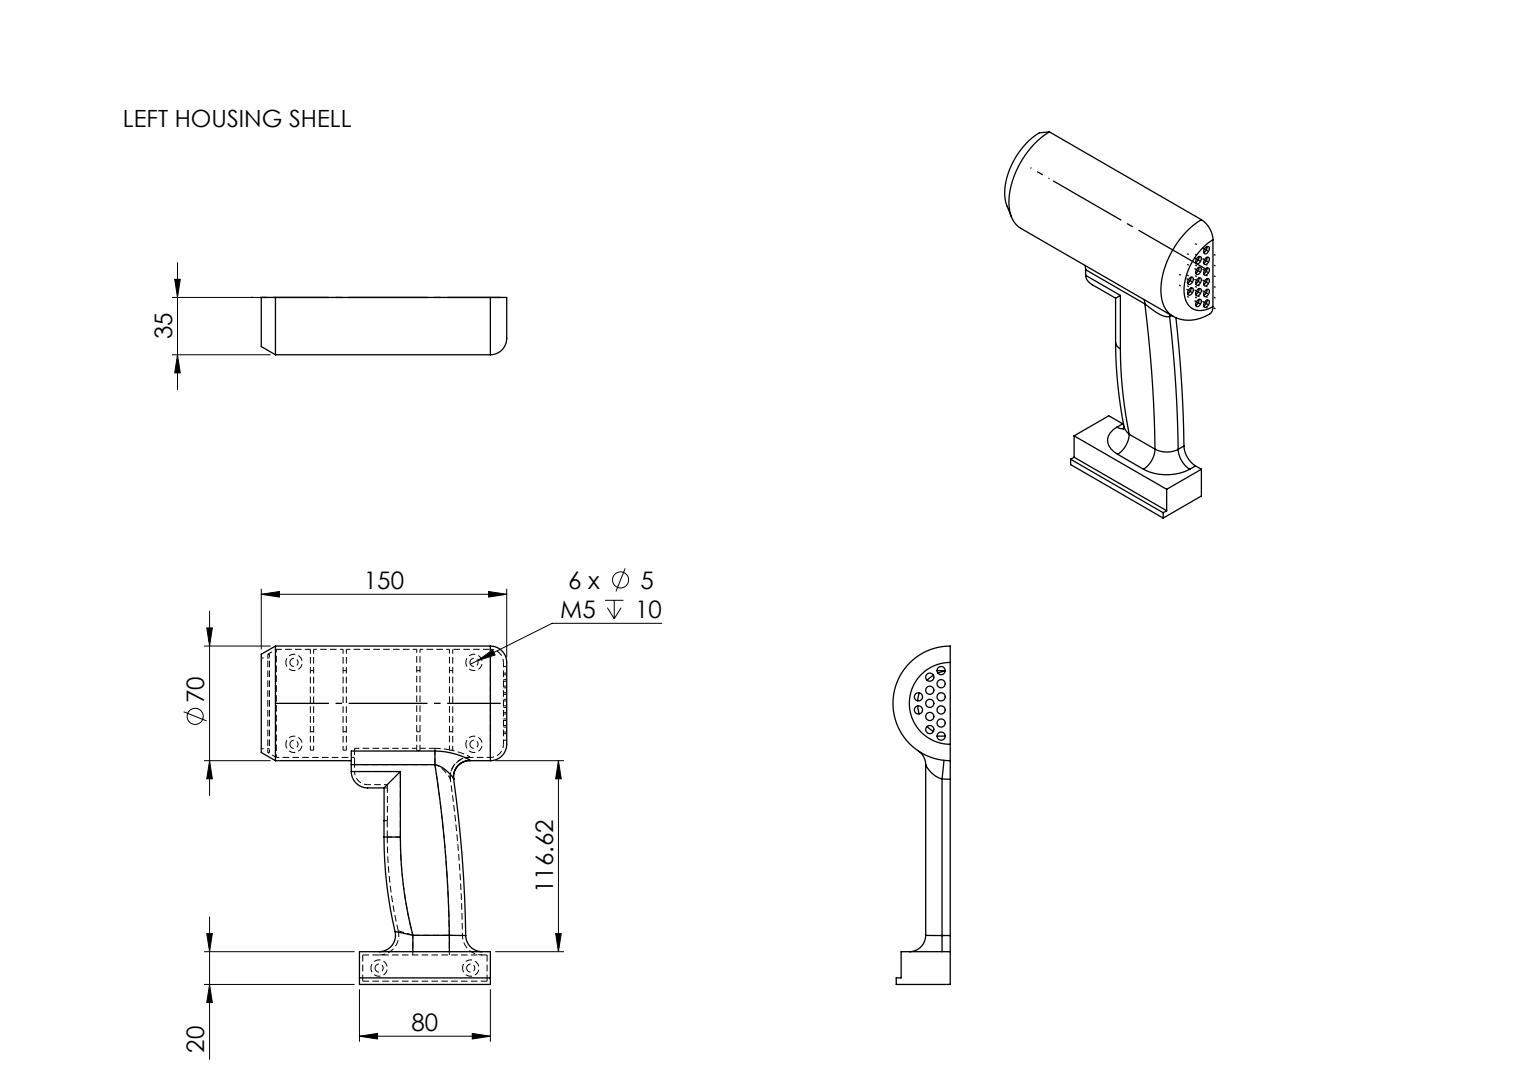
ISO-10303-21;
HEADER;
FILE_DESCRIPTION (('STEP AP214'),
    '1' );
FILE_NAME ('Left Housing Shell.step',
    '2026-10-05T20:22:16',
    ( '' ),
    ( '' ),
    'SwSTEP 2.0',
    'SolidWorks 2026',
    '' );
FILE_SCHEMA (( 'AUTOMOTIVE_DESIGN' ));
ENDSEC;

DATA;
#11=CARTESIAN_POINT ( 'NONE',  ( -70.00000000000000000, 171.6227766016838245, 0.000000000000000000 ) ) ;
#12=ORIENTED_EDGE ( 'NONE', *, *, #6579, .T. ) ;
#17=CARTESIAN_POINT ( 'NONE',  ( 196.0000000000000000, 191.6227766016837677, 3.071800142134975431 ) ) ;
#19=CYLINDRICAL_SURFACE ( 'NONE', #8941, 2.500000000000000444 ) ;
#20=ORIENTED_EDGE ( 'NONE', *, *, #455, .F. ) ;
#21=CARTESIAN_POINT ( 'NONE',  ( -12.77984573873758656, 20.00000000000230216, 11.87289823213939854 ) ) ;
#22=CARTESIAN_POINT ( 'NONE',  ( 14.63750484765316706, 138.5418767416829837, 5.508738673615532377 ) ) ;
#24=CARTESIAN_POINT ( 'NONE',  ( 21.36708699129162881, 19.99999999999999645, 23.94811280430947420 ) ) ;
#25=EDGE_CURVE ( 'NONE', #5251, #13584, #2714, .T. ) ;
#30=CARTESIAN_POINT ( 'NONE',  ( -15.00000000000002132, 100.0000000000000142, 4.999999999999999112 ) ) ;
#33=ADVANCED_FACE ( 'NONE', ( #8260 ), #11261, .F. ) ;
#34=EDGE_CURVE ( 'NONE', #17370, #11003, #7190, .T. ) ;
#39=FACE_OUTER_BOUND ( 'NONE', #11505, .T. ) ;
#42=ORIENTED_EDGE ( 'NONE', *, *, #11841, .T. ) ;
#44=CARTESIAN_POINT ( 'NONE',  ( 9.986687348566183786, 132.8041431104223307, 14.33374896416919064 ) ) ;
#47=CARTESIAN_POINT ( 'NONE',  ( -40.85786437626905609, 120.0000000000000142, 10.85786437626904721 ) ) ;
#52=DIRECTION ( 'NONE',  ( 0.000000000000000000, 0.000000000000000000, -1.000000000000000000 ) ) ;
#53=CARTESIAN_POINT ( 'NONE',  ( -80.79725519073433304, 151.5627461462769929, 26.20297826401936803 ) ) ;
#56=CARTESIAN_POINT ( 'NONE',  ( 14.34366722128227067, 129.4994645064758174, 11.74322308516846647 ) ) ;
#58=CARTESIAN_POINT ( 'NONE',  ( -43.00000000000000000, 144.1839557653416080, 18.33333333333335702 ) ) ;
#59=PLANE ( 'NONE',  #13735 ) ;
#61=EDGE_CURVE ( 'NONE', #735, #11290, #4368, .T. ) ;
#63=FACE_OUTER_BOUND ( 'NONE', #17014, .T. ) ;
#64=ORIENTED_EDGE ( 'NONE', *, *, #1601, .F. ) ;
#66=LINE ( 'NONE', #2892, #16980 ) ;
#69=CARTESIAN_POINT ( 'NONE',  ( 0.000000000000000000, 20.00000000000000000, 25.00000000000000000 ) ) ;
#74=( NAMED_UNIT ( * ) PLANE_ANGLE_UNIT ( ) SI_UNIT ( $, .RADIAN. ) );
#76=ADVANCED_FACE ( 'NONE', ( #15069 ), #3033, .F. ) ;
#78=EDGE_CURVE ( 'NONE', #10896, #7127, #13853, .T. ) ;
#81=EDGE_CURVE ( 'NONE', #4275, #9730, #165, .T. ) ;
#85=DIRECTION ( 'NONE',  ( -1.000000000000000000, -0.000000000000000000, -0.000000000000000000 ) ) ;
#91=LINE ( 'NONE', #4168, #1104 ) ;
#96=EDGE_LOOP ( 'NONE', ( #1824, #2335, #11852, #6103 ) ) ;
#100=PLANE ( 'NONE',  #16536 ) ;
#104=ORIENTED_EDGE ( 'NONE', *, *, #3991, .F. ) ;
#106=DIRECTION ( 'NONE',  ( -1.000000000000000000, 0.000000000000000000, 0.000000000000000000 ) ) ;
#120=ORIENTED_EDGE ( 'NONE', *, *, #14822, .T. ) ;
#124=CARTESIAN_POINT ( 'NONE',  ( 10.15450428991780285, 132.7081580017661224, 14.27405243007192581 ) ) ;
#132=CARTESIAN_POINT ( 'NONE',  ( -24.99999999999999289, 100.0000000000000142, 0.000000000000000000 ) ) ;
#133=CIRCLE ( 'NONE', #1548, 2.499999999999998668 ) ;
#135=CYLINDRICAL_SURFACE ( 'NONE', #5598, 8.000000000000007105 ) ;
#139=LINE ( 'NONE', #14923, #9291 ) ;
#140=FACE_OUTER_BOUND ( 'NONE', #14292, .T. ) ;
#142=CARTESIAN_POINT ( 'NONE',  ( -82.50000000000001421, 196.6227766016838245, 0.000000000000000000 ) ) ;
#143=ORIENTED_EDGE ( 'NONE', *, *, #14951, .F. ) ;
#144=EDGE_CURVE ( 'NONE', #16894, #7251, #3853, .T. ) ;
#154=CARTESIAN_POINT ( 'NONE',  ( 196.0000000000000000, 175.6227766016838530, 21.92820660268601074 ) ) ;
#156=CARTESIAN_POINT ( 'NONE',  ( -3.000000000000000888, 171.6227766016838245, 0.000000000000000000 ) ) ;
#161=DIRECTION ( 'NONE',  ( 0.000000000000000000, 0.000000000000000000, -1.000000000000000000 ) ) ;
#163=EDGE_LOOP ( 'NONE', ( #2201, #7278 ) ) ;
#165=CIRCLE ( 'NONE', #16002, 2.500000000000002220 ) ;
#167=CARTESIAN_POINT ( 'NONE',  ( -7.379000772444994638, 30.00000000000000000, 25.00000000000000000 ) ) ;
#168=CIRCLE ( 'NONE', #8369, 12.00000000000000000 ) ;
#170=CARTESIAN_POINT ( 'NONE',  ( 17.00000000000000000, 154.3022685259950038, 9.999999999999900524 ) ) ;
#172=CARTESIAN_POINT ( 'NONE',  ( 15.46067906867578046, 29.98929614515185804, 13.00000000000000533 ) ) ;
#174=EDGE_CURVE ( 'NONE', #6874, #11959, #3395, .T. ) ;
#179=CARTESIAN_POINT ( 'NONE',  ( 49.99999999999998579, 187.6227766016837961, 12.50000337241049309 ) ) ;
#186=ORIENTED_EDGE ( 'NONE', *, *, #12034, .F. ) ;
#187=CARTESIAN_POINT ( 'NONE',  ( -25.16839285024614625, 19.99999999999999645, 15.12082343620048519 ) ) ;
#189=DIRECTION ( 'NONE',  ( 0.000000000000000000, 1.000000000000000000, 0.000000000000000000 ) ) ;
#190=VERTEX_POINT ( 'NONE', #15337 ) ;
#193=CARTESIAN_POINT ( 'NONE',  ( -95.00000000000000000, 171.6227766016838245, 0.000000000000000000 ) ) ;
#199=CYLINDRICAL_SURFACE ( 'NONE', #1827, 5.000000000000000888 ) ;
#202=FACE_OUTER_BOUND ( 'NONE', #3833, .T. ) ;
#206=B_SPLINE_CURVE_WITH_KNOTS ( 'NONE', 3,
 ( #3287, #16669, #445, #365, #283, #11345, #15732, #8689, #8323, #15407, #4447, #11249, #548, #7099, #5687, #9833, #14096, #7178, #17064, #1960, #11419, #12580, #4538, #1702, #8592, #1874 ),
 .UNSPECIFIED., .F., .F.,
 ( 4, 2, 2, 2, 2, 2, 2, 2, 2, 2, 2, 2, 4 ),
 ( 0.000000000000000000, 0.002002783134349999609, 0.004005566268699999218, 0.008011132537399998435, 0.01001391567174999414, 0.01201669880609998985, 0.01602226507479997952, 0.01802504820914997002, 0.02002783134349995706, 0.02403339761219993806, 0.02603618074654992856, 0.02803896388089991906, 0.03204453014959990353 ),
 .UNSPECIFIED. ) ;
#208=ORIENTED_EDGE ( 'NONE', *, *, #12480, .F. ) ;
#210=CARTESIAN_POINT ( 'NONE',  ( 15.00000000000000000, 204.6227766016838245, -2.020667218593133100E-15 ) ) ;
#212=CARTESIAN_POINT ( 'NONE',  ( 17.58250999372313927, 125.2198453307267414, 1.671679122699602171 ) ) ;
#213=DIRECTION ( 'NONE',  ( -1.000000000000000000, 0.000000000000000000, 0.000000000000000000 ) ) ;
#215=CIRCLE ( 'NONE', #1923, 5.000000000000018652 ) ;
#216=VERTEX_POINT ( 'NONE', #8789 ) ;
#223=CARTESIAN_POINT ( 'NONE',  ( 27.44407568426044364, 136.8394969516870958, 3.888888888888887063 ) ) ;
#225=ORIENTED_EDGE ( 'NONE', *, *, #16801, .F. ) ;
#231=CARTESIAN_POINT ( 'NONE',  ( -45.00000000000000000, 122.0000000000000142, 15.00000000000000000 ) ) ;
#236=LINE ( 'NONE', #5641, #6716 ) ;
#237=EDGE_LOOP ( 'NONE', ( #1431, #15859, #12881, #16657, #10889, #7991, #12906, #8862 ) ) ;
#239=CARTESIAN_POINT ( 'NONE',  ( 196.0000000000000000, 179.6227766016838245, 15.00000337241049486 ) ) ;
#241=AXIS2_PLACEMENT_3D ( 'NONE', #3615, #7420, #699 ) ;
#244=CARTESIAN_POINT ( 'NONE',  ( -100.0000000000000000, 143.9321776784423150, -5.086680500673126297E-15 ) ) ;
#247=FACE_BOUND ( 'NONE', #9621, .T. ) ;
#248=ADVANCED_FACE ( 'NONE', ( #14797, #17095 ), #7707, .F. ) ;
#250=EDGE_CURVE ( 'NONE', #2500, #6282, #1348, .T. ) ;
#252=CIRCLE ( 'NONE', #11000, 2.500000000000000000 ) ;
#254=VERTEX_POINT ( 'NONE', #2317 ) ;
#255=FACE_BOUND ( 'NONE', #9759, .T. ) ;
#262=CIRCLE ( 'NONE', #2818, 2.499999999999998668 ) ;
#264=AXIS2_PLACEMENT_3D ( 'NONE', #14224, #8819, #502 ) ;
#266=CARTESIAN_POINT ( 'NONE',  ( 19.82112781281243130, 29.90253658286262350, 11.35562597552217845 ) ) ;
#276=CARTESIAN_POINT ( 'NONE',  ( -15.53366225407947354, 31.76144936975385136, 11.66511309525283835 ) ) ;
#277=CIRCLE ( 'NONE', #6204, 20.00000000000000355 ) ;
#279=EDGE_CURVE ( 'NONE', #3972, #817, #6479, .T. ) ;
#280=ORIENTED_EDGE ( 'NONE', *, *, #8979, .F. ) ;
#283=CARTESIAN_POINT ( 'NONE',  ( -27.70723240392776887, 18.00000000000000000, 8.328409877367404235 ) ) ;
#288=LINE ( 'NONE', #8596, #3725 ) ;
#291=DIRECTION ( 'NONE',  ( -1.000000000000000000, 0.000000000000000000, 0.000000000000000000 ) ) ;
#292=EDGE_LOOP ( 'NONE', ( #6190, #15449, #12115, #5130, #6244, #17037, #12475 ) ) ;
#294=EDGE_LOOP ( 'NONE', ( #280, #3412, #14427, #14815 ) ) ;
#306=CARTESIAN_POINT ( 'NONE',  ( 16.12877328687227774, 136.8349817083154676, 4.209125965272636272 ) ) ;
#310=CARTESIAN_POINT ( 'NONE',  ( -50.00000000000000000, 171.6227766016838245, 0.000000000000000000 ) ) ;
#312=FACE_OUTER_BOUND ( 'NONE', #3125, .T. ) ;
#315=CIRCLE ( 'NONE', #13889, 10.00000000000000178 ) ;
#317=DIRECTION ( 'NONE',  ( -1.000000000000000000, 0.000000000000000000, 0.000000000000000000 ) ) ;
#319=ORIENTED_EDGE ( 'NONE', *, *, #15425, .T. ) ;
#320=EDGE_CURVE ( 'NONE', #5614, #12465, #7243, .T. ) ;
#322=PLANE ( 'NONE',  #5083 ) ;
#324=DIRECTION ( 'NONE',  ( 0.8571673013836870192, 1.049727191973306873E-16, -0.5150380737757234151 ) ) ;
#333=CARTESIAN_POINT ( 'NONE',  ( -100.0000000000000000, 171.6227766016838245, 0.000000000000000000 ) ) ;
#335=FACE_BOUND ( 'NONE', #8357, .T. ) ;
#339=ORIENTED_EDGE ( 'NONE', *, *, #6159, .F. ) ;
#342=ORIENTED_EDGE ( 'NONE', *, *, #14528, .T. ) ;
#343=FILL_AREA_STYLE_COLOUR ( '', #7574 ) ;
#347=CARTESIAN_POINT ( 'NONE',  ( 25.75727093772393061, 193.9598103731634637, 24.29383909379279061 ) ) ;
#351=CARTESIAN_POINT ( 'NONE',  ( -79.90458729923355463, 201.6232707959690060, 13.74664867617476460 ) ) ;
#354=ORIENTED_EDGE ( 'NONE', *, *, #25, .T. ) ;
#359=CARTESIAN_POINT ( 'NONE',  ( -27.98221281347032274, 19.99999999999999645, 4.999999999999996447 ) ) ;
#364=EDGE_CURVE ( 'NONE', #14743, #3326, #2669, .T. ) ;
#365=CARTESIAN_POINT ( 'NONE',  ( -27.81025873171734375, 18.00000000000000355, 7.666431193274476641 ) ) ;
#368=DIRECTION ( 'NONE',  ( -1.000000000000000000, -0.000000000000000000, -0.000000000000000000 ) ) ;
#370=FACE_OUTER_BOUND ( 'NONE', #15719, .T. ) ;
#380=CARTESIAN_POINT ( 'NONE',  ( 15.95607457770042181, 136.6882381644217048, 2.475222843549475638 ) ) ;
#381=CARTESIAN_POINT ( 'NONE',  ( 13.38958197704232056, 130.3612470323695902, 12.52688079436099144 ) ) ;
#382=ORIENTED_EDGE ( 'NONE', *, *, #10198, .F. ) ;
#385=CARTESIAN_POINT ( 'NONE',  ( -81.89019958151206424, 191.9899036175949618, 25.96511099662697930 ) ) ;
#386=DIRECTION ( 'NONE',  ( 0.000000000000000000, 0.000000000000000000, 1.000000000000000000 ) ) ;
#387=CARTESIAN_POINT ( 'NONE',  ( 17.50698843878764777, 29.94827730614627725, 12.57924512168886011 ) ) ;
#391=ADVANCED_FACE ( 'NONE', ( #9825 ), #19, .F. ) ;
#394=EDGE_CURVE ( 'NONE', #12251, #2211, #12340, .T. ) ;
#400=ORIENTED_EDGE ( 'NONE', *, *, #61, .T. ) ;
#401=CARTESIAN_POINT ( 'NONE',  ( 8.997728150919979129, 132.8900016178789372, 12.55705910147062099 ) ) ;
#402=EDGE_LOOP ( 'NONE', ( #8088, #12658, #10491, #2591 ) ) ;
#404=CARTESIAN_POINT ( 'NONE',  ( 30.00000000000000355, 196.6227766016838245, 35.00200000000000244 ) ) ;
#405=FACE_OUTER_BOUND ( 'NONE', #3645, .T. ) ;
#407=CARTESIAN_POINT ( 'NONE',  ( -96.00000000000001421, 201.6227766016838245, 0.000000000000000000 ) ) ;
#412=CARTESIAN_POINT ( 'NONE',  ( 27.31119513844540947, 142.3932571782017931, 15.32207027268389510 ) ) ;
#414=FACE_BOUND ( 'NONE', #1666, .T. ) ;
#416=AXIS2_PLACEMENT_3D ( 'NONE', #17010, #17352, #6371 ) ;
#420=CARTESIAN_POINT ( 'NONE',  ( -50.00000000000000000, 191.6227766016837961, -1.224646799147353454E-15 ) ) ;
#423=CARTESIAN_POINT ( 'NONE',  ( 40.00000000000000711, 146.6227766016838245, 0.000000000000000000 ) ) ;
#426=FACE_BOUND ( 'NONE', #13934, .T. ) ;
#429=DIRECTION ( 'NONE',  ( -0.000000000000000000, -0.000000000000000000, -1.000000000000000000 ) ) ;
#431=CARTESIAN_POINT ( 'NONE',  ( -80.14161447679168759, 201.6221756766236979, 13.74903839801200789 ) ) ;
#435=EDGE_LOOP ( 'NONE', ( #4715, #8702, #12659, #943, #16358, #4658 ) ) ;
#438=ORIENTED_EDGE ( 'NONE', *, *, #11422, .T. ) ;
#439=CARTESIAN_POINT ( 'NONE',  ( -14.83003349241583813, 19.99999999999883116, 8.298189366023557056 ) ) ;
#445=CARTESIAN_POINT ( 'NONE',  ( -27.94760966554430937, 18.00000000000000355, 6.338314452217974626 ) ) ;
#449=PLANE ( 'NONE',  #5426 ) ;
#455=EDGE_CURVE ( 'NONE', #7796, #10705, #11208, .T. ) ;
#461=DIRECTION ( 'NONE',  ( -0.000000000000000000, -0.000000000000000000, -1.000000000000000000 ) ) ;
#465=CARTESIAN_POINT ( 'NONE',  ( 24.34257225596279639, 138.6622241066778543, 11.80661878326775494 ) ) ;
#466=VECTOR ( 'NONE', #9041, 1000.000000000000000 ) ;
#476=CARTESIAN_POINT ( 'NONE',  ( -78.09342651567857274, 191.9854139975492160, 25.96938468333279104 ) ) ;
#477=DIRECTION ( 'NONE',  ( -1.000000000000000000, -0.000000000000000000, -0.000000000000000000 ) ) ;
#478=CARTESIAN_POINT ( 'NONE',  ( 19.81659905433974700, 29.90262535319825332, 11.35915249282563444 ) ) ;
#481=DIRECTION ( 'NONE',  ( 0.000000000000000000, 1.000000000000000000, 0.000000000000000000 ) ) ;
#484=DIRECTION ( 'NONE',  ( -1.000000000000000000, 0.000000000000000000, 0.000000000000000000 ) ) ;
#488=ORIENTED_EDGE ( 'NONE', *, *, #9995, .F. ) ;
#491=CIRCLE ( 'NONE', #16041, 33.00000000000000000 ) ;
#494=CARTESIAN_POINT ( 'NONE',  ( 40.00000000000000711, 171.6227766016838245, 0.000000000000000000 ) ) ;
#501=CARTESIAN_POINT ( 'NONE',  ( 40.00000000000000711, 204.6227766016838245, -2.020667218593133100E-15 ) ) ;
#502=DIRECTION ( 'NONE',  ( -1.000000000000000000, 0.000000000000000000, 0.000000000000000000 ) ) ;
#504=AXIS2_PLACEMENT_3D ( 'NONE', #14770, #8028, #16194 ) ;
#512=LINE ( 'NONE', #4502, #12581 ) ;
#515=CIRCLE ( 'NONE', #6739, 8.000000000000000000 ) ;
#517=CARTESIAN_POINT ( 'NONE',  ( -75.00000000000002842, 146.6227766016838245, 0.000000000000000000 ) ) ;
#519=ORIENTED_EDGE ( 'NONE', *, *, #4625, .F. ) ;
#520=EDGE_CURVE ( 'NONE', #7447, #15746, #3010, .T. ) ;
#522=ADVANCED_FACE ( 'NONE', ( #13830 ), #1695, .F. ) ;
#524=EDGE_LOOP ( 'NONE', ( #9216, #14969 ) ) ;
#529=CARTESIAN_POINT ( 'NONE',  ( 27.99999999999998224, 9.999999999999998224, 0.000000000000000000 ) ) ;
#530=CARTESIAN_POINT ( 'NONE',  ( -77.50000000000001421, 196.6227766016838245, 10.00000000000000178 ) ) ;
#531=AXIS2_PLACEMENT_3D ( 'NONE', #7704, #6212, #3646 ) ;
#532=CARTESIAN_POINT ( 'NONE',  ( -79.43217333917553447, 201.5917424073650182, 13.81529814621275953 ) ) ;
#536=ORIENTED_EDGE ( 'NONE', *, *, #1514, .F. ) ;
#540=ADVANCED_FACE ( 'NONE', ( #12491 ), #2116, .T. ) ;
#541=CARTESIAN_POINT ( 'NONE',  ( 35.00000000000000711, 146.6227766016838245, 35.00200000000000244 ) ) ;
#544=VERTEX_POINT ( 'NONE', #5945 ) ;
#545=AXIS2_PLACEMENT_3D ( 'NONE', #15355, #5797, #5891 ) ;
#547=AXIS2_PLACEMENT_3D ( 'NONE', #310, #15173, #4211 ) ;
#548=CARTESIAN_POINT ( 'NONE',  ( -22.79696676584440596, 18.00000000000000711, 18.34105320469107170 ) ) ;
#549=CYLINDRICAL_SURFACE ( 'NONE', #11760, 35.00000000000000000 ) ;
#551=CARTESIAN_POINT ( 'NONE',  ( -7.379000772444995526, 18.00000000000000355, 12.99999999999999822 ) ) ;
#552=DIRECTION ( 'NONE',  ( 1.000000000000000000, 0.000000000000000000, 0.000000000000000000 ) ) ;
#557=VECTOR ( 'NONE', #9968, 1000.000000000000114 ) ;
#558=AXIS2_PLACEMENT_3D ( 'NONE', #9560, #17361, #13561 ) ;
#560=CARTESIAN_POINT ( 'NONE',  ( -90.80384757729339640, 204.6227766016838245, 0.000000000000000000 ) ) ;
#563=ORIENTED_EDGE ( 'NONE', *, *, #11755, .F. ) ;
#565=CARTESIAN_POINT ( 'NONE',  ( 23.79315516583586643, 19.99999999999999645, 22.94240041036162836 ) ) ;
#567=CARTESIAN_POINT ( 'NONE',  ( 15.80099858973940030, 127.9994182179736413, 10.08996921773076316 ) ) ;
#570=VERTEX_POINT ( 'NONE', #6023 ) ;
#572=EDGE_CURVE ( 'NONE', #3368, #13835, #6120, .T. ) ;
#573=CIRCLE ( 'NONE', #11580, 2.500000000000000444 ) ;
#576=DIRECTION ( 'NONE',  ( 0.000000000000000000, 0.000000000000000000, 1.000000000000000000 ) ) ;
#577=DIRECTION ( 'NONE',  ( -1.000000000000000000, 1.040834085586084059E-15, 0.000000000000000000 ) ) ;
#578=CARTESIAN_POINT ( 'NONE',  ( 17.01529014380724192, 17.99999999999942801, 12.76845467807931733 ) ) ;
#580=ORIENTED_EDGE ( 'NONE', *, *, #7866, .T. ) ;
#581=CARTESIAN_POINT ( 'NONE',  ( -725.0000000000000000, 30.00000000000000000, 13.00000000000000000 ) ) ;
#582=CARTESIAN_POINT ( 'NONE',  ( 225.0000000000000000, 89.99999999999997158, 4.999999999999999112 ) ) ;
#586=AXIS2_PLACEMENT_3D ( 'NONE', #156, #1313, #13701 ) ;
#587=ORIENTED_EDGE ( 'NONE', *, *, #6448, .T. ) ;
#589=ORIENTED_EDGE ( 'NONE', *, *, #4843, .T. ) ;
#591=CARTESIAN_POINT ( 'NONE',  ( 11.63249183333955017, 139.6944596454877114, 10.84829254633709184 ) ) ;
#592=ORIENTED_EDGE ( 'NONE', *, *, #11333, .F. ) ;
#594=ORIENTED_EDGE ( 'NONE', *, *, #13777, .F. ) ;
#596=DIRECTION ( 'NONE',  ( 1.000000000000000000, 0.000000000000000000, 0.000000000000000000 ) ) ;
#597=CARTESIAN_POINT ( 'NONE',  ( 13.91851620013868995, 127.9827558526829563, 9.294367823883964874 ) ) ;
#605=PLANE ( 'NONE',  #3116 ) ;
#610=ORIENTED_EDGE ( 'NONE', *, *, #4593, .T. ) ;
#611=LINE ( 'NONE', #16893, #6704 ) ;
#618=DIRECTION ( 'NONE',  ( 0.000000000000000000, 0.000000000000000000, -1.000000000000000000 ) ) ;
#620=CARTESIAN_POINT ( 'NONE',  ( -80.49255897422042949, 201.5998317580112200, 13.79770299781518972 ) ) ;
#622=ORIENTED_EDGE ( 'NONE', *, *, #10511, .F. ) ;
#629=LINE ( 'NONE', #6194, #9795 ) ;
#634=CARTESIAN_POINT ( 'NONE',  ( -27.98221281347037959, 20.00000000000000000, 4.999999999999999112 ) ) ;
#639=CARTESIAN_POINT ( 'NONE',  ( -12.55890155933014363, 17.99999999999884182, 7.515612101507582743 ) ) ;
#640=LINE ( 'NONE', #12678, #3519 ) ;
#642=ORIENTED_EDGE ( 'NONE', *, *, #1514, .T. ) ;
#647=VERTEX_POINT ( 'NONE', #3540 ) ;
#649=CARTESIAN_POINT ( 'NONE',  ( 24.93507336697333798, 29.86842105264641845, 5.660862367392566874 ) ) ;
#650=CARTESIAN_POINT ( 'NONE',  ( 14.18611645313626290, 129.6406627243902676, 11.87032202561248617 ) ) ;
#653=DIRECTION ( 'NONE',  ( -1.000000000000000000, -0.000000000000000000, -0.000000000000000000 ) ) ;
#655=CARTESIAN_POINT ( 'NONE',  ( -75.10425368493336862, 195.5720014495396981, 22.70655749026625614 ) ) ;
#658=EDGE_CURVE ( 'NONE', #1654, #17318, #629, .T. ) ;
#660=DIRECTION ( 'NONE',  ( 0.8571673013836867971, 1.049727191973306626E-16, -0.5150380737757237481 ) ) ;
#663=DIRECTION ( 'NONE',  ( 1.000000000000000000, 0.000000000000000000, -0.000000000000000000 ) ) ;
#669=ORIENTED_EDGE ( 'NONE', *, *, #10810, .F. ) ;
#670=ORIENTED_EDGE ( 'NONE', *, *, #4740, .F. ) ;
#673=LINE ( 'NONE', #4749, #14088 ) ;
#674=EDGE_LOOP ( 'NONE', ( #1760, #15151, #9125, #15624 ) ) ;
#676=DIRECTION ( 'NONE',  ( 0.000000000000000000, 1.000000000000000000, 0.000000000000000000 ) ) ;
#677=CARTESIAN_POINT ( 'NONE',  ( 11.61330907248435018, 130.6704317944142986, 11.35602788888950698 ) ) ;
#682=CARTESIAN_POINT ( 'NONE',  ( 32.67951861369070343, 142.3872899932706844, 15.31067380954020862 ) ) ;
#687=EDGE_CURVE ( 'NONE', #15915, #10010, #12076, .T. ) ;
#688=ADVANCED_FACE ( 'NONE', ( #5209 ), #12027, .F. ) ;
#692=ORIENTED_EDGE ( 'NONE', *, *, #13103, .T. ) ;
#693=CARTESIAN_POINT ( 'NONE',  ( 196.0000000000000000, 175.6227766016838245, 8.071800142134975431 ) ) ;
#695=ORIENTED_EDGE ( 'NONE', *, *, #11443, .F. ) ;
#699=DIRECTION ( 'NONE',  ( 0.000000000000000000, 0.000000000000000000, -1.000000000000000000 ) ) ;
#700=EDGE_CURVE ( 'NONE', #11501, #8340, #15923, .T. ) ;
#703=FACE_OUTER_BOUND ( 'NONE', #16932, .T. ) ;
#704=DIRECTION ( 'NONE',  ( 0.000000000000000000, 0.000000000000000000, -1.000000000000000000 ) ) ;
#705=CARTESIAN_POINT ( 'NONE',  ( -75.98683855290481404, 199.6193856840139631, 17.47499078086475777 ) ) ;
#706=CARTESIAN_POINT ( 'NONE',  ( 50.00000000000000000, 171.6227766016838245, 0.000000000000000000 ) ) ;
#708=ORIENTED_EDGE ( 'NONE', *, *, #14469, .F. ) ;
#710=ORIENTED_EDGE ( 'NONE', *, *, #6159, .T. ) ;
#712=DIRECTION ( 'NONE',  ( -0.8571673013836867971, 0.000000000000000000, -0.5150380737757237481 ) ) ;
#715=DIRECTION ( 'NONE',  ( -0.000000000000000000, -0.000000000000000000, -1.000000000000000000 ) ) ;
#716=EDGE_LOOP ( 'NONE', ( #4936, #15212, #7223, #17300 ) ) ;
#719=EDGE_CURVE ( 'NONE', #2134, #4864, #6633, .T. ) ;
#722=VECTOR ( 'NONE', #15291, 1000.000000000000000 ) ;
#723=CARTESIAN_POINT ( 'NONE',  ( 48.00000000000000000, 171.6227766016838245, 10.00000337241048953 ) ) ;
#725=CARTESIAN_POINT ( 'NONE',  ( -9.392228533940972568, 30.65825049985634010, 12.80200153553487752 ) ) ;
#728=ORIENTED_EDGE ( 'NONE', *, *, #8884, .T. ) ;
#729=LINE ( 'NONE', #14192, #7026 ) ;
#734=CIRCLE ( 'NONE', #12313, 12.00000000000000000 ) ;
#735=VERTEX_POINT ( 'NONE', #16202 ) ;
#736=CARTESIAN_POINT ( 'NONE',  ( 20.13757169487763576, 19.99999999999999289, 24.32197800972832624 ) ) ;
#738=CARTESIAN_POINT ( 'NONE',  ( 19.35452547490215736, 29.94096051140668280, 13.97567760708249551 ) ) ;
#740=EDGE_LOOP ( 'NONE', ( #2992, #17252, #2513 ) ) ;
#742=CARTESIAN_POINT ( 'NONE',  ( -27.98221281347037959, 18.00000000000000355, 0.000000000000000000 ) ) ;
#744=CARTESIAN_POINT ( 'NONE',  ( -75.75631164580342158, 193.9611582889532428, 24.29263104154016872 ) ) ;
#745=PLANE ( 'NONE',  #2292 ) ;
#747=AXIS2_PLACEMENT_3D ( 'NONE', #1269, #14466, #10656 ) ;
#748=CARTESIAN_POINT ( 'NONE',  ( -95.00000000000000000, 171.6227766016838245, 0.000000000000000000 ) ) ;
#757=ORIENTED_EDGE ( 'NONE', *, *, #700, .T. ) ;
#758=AXIS2_PLACEMENT_3D ( 'NONE', #15657, #11594, #14252 ) ;
#767=CARTESIAN_POINT ( 'NONE',  ( 6.471945315774715546, 134.1315750335306518, 12.99999999999999822 ) ) ;
#768=DIRECTION ( 'NONE',  ( 1.000000000000000000, 0.000000000000000000, 0.000000000000000000 ) ) ;
#769=CYLINDRICAL_SURFACE ( 'NONE', #12299, 20.00000000000000355 ) ;
#781=ORIENTED_EDGE ( 'NONE', *, *, #1682, .T. ) ;
#783=FACE_OUTER_BOUND ( 'NONE', #7773, .T. ) ;
#786=CARTESIAN_POINT ( 'NONE',  ( 12.82244027866276426, 141.9777490571136696, 18.60671400555900235 ) ) ;
#790=EDGE_CURVE ( 'NONE', #4054, #1871, #14156, .T. ) ;
#792=ADVANCED_FACE ( 'NONE', ( #11571 ), #7415, .T. ) ;
#798=( BOUNDED_CURVE ( )  B_SPLINE_CURVE ( 3, ( #13819, #11137, #7085, #11329 ),
 .UNSPECIFIED., .F., .F. ) 
 B_SPLINE_CURVE_WITH_KNOTS ( ( 4, 4 ),
 ( -8.881784197001252323E-16, 1.570796326794898556 ),
 .UNSPECIFIED. ) 
 CURVE ( )  GEOMETRIC_REPRESENTATION_ITEM ( )  RATIONAL_B_SPLINE_CURVE ( ( 1.000000000000000000, 0.8047378541243643824, 0.8047378541243643824, 1.000000000000000000 ) ) 
 REPRESENTATION_ITEM ( '' )  );
#805=VERTEX_POINT ( 'NONE', #8484 ) ;
#806=CARTESIAN_POINT ( 'NONE',  ( -80.00000000000002842, 146.6227766016838245, 35.00200000000000244 ) ) ;
#808=ORIENTED_EDGE ( 'NONE', *, *, #995, .F. ) ;
#810=VECTOR ( 'NONE', #1968, 1000.000000000000000 ) ;
#812=LINE ( 'NONE', #2307, #4993 ) ;
#813=CARTESIAN_POINT ( 'NONE',  ( -95.00000000000000000, 171.6227766016838245, 0.000000000000000000 ) ) ;
#814=CARTESIAN_POINT ( 'NONE',  ( -10.13698291596435119, 17.99999999999999645, 11.46558158188963539 ) ) ;
#816=CARTESIAN_POINT ( 'NONE',  ( 25.49999999999998579, 9.999999999999998224, 10.00000000000000178 ) ) ;
#817=VERTEX_POINT ( 'NONE', #15375 ) ;
#819=ORIENTED_EDGE ( 'NONE', *, *, #81, .F. ) ;
#823=EDGE_CURVE ( 'NONE', #16300, #1130, #11027, .T. ) ;
#826=DIRECTION ( 'NONE',  ( -1.000000000000000000, 0.000000000000000000, 0.000000000000000000 ) ) ;
#827=VECTOR ( 'NONE', #14654, 1000.000000000000000 ) ;
#828=CARTESIAN_POINT ( 'NONE',  ( 19.05951714192248403, 29.94485528828719367, 14.11495713418740294 ) ) ;
#830=CARTESIAN_POINT ( 'NONE',  ( 196.0000000000000000, 187.6227766016837961, 12.50000337241049309 ) ) ;
#832=VECTOR ( 'NONE', #2538, 1000.000000000000000 ) ;
#837=ORIENTED_EDGE ( 'NONE', *, *, #15585, .T. ) ;
#847=EDGE_CURVE ( 'NONE', #16728, #15915, #15300, .T. ) ;
#855=CARTESIAN_POINT ( 'NONE',  ( -13.87134331504352325, 32.05147385205248867, 10.53504704850738705 ) ) ;
#857=DIRECTION ( 'NONE',  ( 0.000000000000000000, 0.000000000000000000, -1.000000000000000000 ) ) ;
#861=CARTESIAN_POINT ( 'NONE',  ( 26.51307711398865408, 139.5431919169737967, 7.747420853565629706 ) ) ;
#869=CARTESIAN_POINT ( 'NONE',  ( 25.52968048427065284, 198.8808217108463055, 18.60648811928370350 ) ) ;
#870=ORIENTED_EDGE ( 'NONE', *, *, #16889, .F. ) ;
#871=CARTESIAN_POINT ( 'NONE',  ( 0.000000000000000000, 20.00000000000000000, 0.000000000000000000 ) ) ;
#872=CARTESIAN_POINT ( 'NONE',  ( 48.00000000000000711, 175.6227766016838245, 5.571800142134975431 ) ) ;
#873=CIRCLE ( 'NONE', #2278, 5.000000000000004441 ) ;
#875=DIRECTION ( 'NONE',  ( 0.000000000000000000, 0.9938079899999064937, -0.1111111111111109523 ) ) ;
#878=DIRECTION ( 'NONE',  ( 1.000000000000000000, 0.000000000000000000, 0.000000000000000000 ) ) ;
#882=ADVANCED_FACE ( 'NONE', ( #12736 ), #11219, .T. ) ;
#883=DIRECTION ( 'NONE',  ( -0.000000000000000000, -0.000000000000000000, -1.000000000000000000 ) ) ;
#887=CIRCLE ( 'NONE', #13615, 8.000000000000000000 ) ;
#892=FACE_OUTER_BOUND ( 'NONE', #9411, .T. ) ;
#895=ORIENTED_EDGE ( 'NONE', *, *, #16793, .T. ) ;
#900=CARTESIAN_POINT ( 'NONE',  ( -13.23954943057894873, 31.86042443463173157, 11.05847410484002680 ) ) ;
#901=CARTESIAN_POINT ( 'NONE',  ( -27.99999999999998224, 10.00000000000000000, 0.000000000000000000 ) ) ;
#906=CARTESIAN_POINT ( 'NONE',  ( 49.99999999999998579, 171.6227766016838245, 12.50000337241049131 ) ) ;
#911=FACE_OUTER_BOUND ( 'NONE', #5499, .T. ) ;
#912=CARTESIAN_POINT ( 'NONE',  ( 23.61360151038711308, 29.88540148010350705, 10.01045486545366181 ) ) ;
#917=EDGE_CURVE ( 'NONE', #1967, #544, #4724, .T. ) ;
#920=CARTESIAN_POINT ( 'NONE',  ( 48.00000000000000711, 155.6227766016839098, 15.00000337241049486 ) ) ;
#923=DIRECTION ( 'NONE',  ( 0.000000000000000000, 1.387778780781445676E-14, -1.000000000000000000 ) ) ;
#926=ORIENTED_EDGE ( 'NONE', *, *, #9179, .F. ) ;
#934=CARTESIAN_POINT ( 'NONE',  ( 23.09107716886297013, 17.99999999999083045, 5.538990817933215460 ) ) ;
#938=VERTEX_POINT ( 'NONE', #7842 ) ;
#941=DIRECTION ( 'NONE',  ( -0.000000000000000000, -0.000000000000000000, -1.000000000000000000 ) ) ;
#942=CARTESIAN_POINT ( 'NONE',  ( 17.53512989260226362, 29.96507997281579350, 14.66107963853301399 ) ) ;
#943=ORIENTED_EDGE ( 'NONE', *, *, #15549, .T. ) ;
#945=CARTESIAN_POINT ( 'NONE',  ( 30.21607733469937429, 201.6195082837481038, 13.75486997215867291 ) ) ;
#948=ORIENTED_EDGE ( 'NONE', *, *, #5128, .T. ) ;
#949=CARTESIAN_POINT ( 'NONE',  ( -79.08361844431172472, 141.7021811473759669, 13.91989935049637062 ) ) ;
#950=DIRECTION ( 'NONE',  ( 1.000000000000000000, 0.000000000000000000, 0.000000000000000000 ) ) ;
#956=CARTESIAN_POINT ( 'NONE',  ( 48.00000000000000000, 196.6227766016838245, 0.000000000000000000 ) ) ;
#958=ORIENTED_EDGE ( 'NONE', *, *, #11073, .T. ) ;
#961=VECTOR ( 'NONE', #878, 1000.000000000000000 ) ;
#963=ORIENTED_EDGE ( 'NONE', *, *, #823, .F. ) ;
#967=DIRECTION ( 'NONE',  ( -0.000000000000000000, -0.000000000000000000, -1.000000000000000000 ) ) ;
#968=EDGE_CURVE ( 'NONE', #15581, #8813, #1708, .T. ) ;
#973=CARTESIAN_POINT ( 'NONE',  ( -12.54944958582184888, 31.64997543288135873, 11.54276402733058937 ) ) ;
#974=DIRECTION ( 'NONE',  ( -0.000000000000000000, -0.000000000000000000, -1.000000000000000000 ) ) ;
#977=DIRECTION ( 'NONE',  ( -0.000000000000000000, -0.000000000000000000, -1.000000000000000000 ) ) ;
#978=VERTEX_POINT ( 'NONE', #10499 ) ;
#981=ORIENTED_EDGE ( 'NONE', *, *, #16898, .T. ) ;
#983=CARTESIAN_POINT ( 'NONE',  ( 25.87766738269754541, 139.8661988410599406, 8.984976992518891592 ) ) ;
#984=CIRCLE ( 'NONE', #416, 2.500000000000000000 ) ;
#986=CARTESIAN_POINT ( 'NONE',  ( 34.42312820345349422, 19.99999999999999645, 9.539278825327816236 ) ) ;
#995=EDGE_CURVE ( 'NONE', #13884, #3234, #12362, .T. ) ;
#999=ORIENTED_EDGE ( 'NONE', *, *, #17387, .F. ) ;
#1001=AXIS2_PLACEMENT_3D ( 'NONE', #7737, #14563, #8984 ) ;
#1002=DIRECTION ( 'NONE',  ( -1.000000000000000000, 0.000000000000000000, 0.000000000000000000 ) ) ;
#1007=UNCERTAINTY_MEASURE_WITH_UNIT (LENGTH_MEASURE( 1.000000000000000082E-05 ), #2734, 'distance_accuracy_value', 'NONE');
#1011=DIRECTION ( 'NONE',  ( -1.000000000000000000, 0.000000000000000000, 0.000000000000000000 ) ) ;
#1014=CARTESIAN_POINT ( 'NONE',  ( 17.00000000000000000, 171.6227766016838245, 20.00000000000000355 ) ) ;
#1015=CARTESIAN_POINT ( 'NONE',  ( 22.25017171248248005, 17.99999999999771916, 8.611421531743401303 ) ) ;
#1018=CARTESIAN_POINT ( 'NONE',  ( 27.44407568426044008, 138.8271129316868837, 3.666666666666658081 ) ) ;
#1020=DIRECTION ( 'NONE',  ( -0.000000000000000000, -0.000000000000000000, -1.000000000000000000 ) ) ;
#1023=ORIENTED_EDGE ( 'NONE', *, *, #8940, .T. ) ;
#1024=DIRECTION ( 'NONE',  ( 0.000000000000000000, 0.000000000000000000, -1.000000000000000000 ) ) ;
#1027=AXIS2_PLACEMENT_3D ( 'NONE', #6143, #14706, #8870 ) ;
#1033=EDGE_LOOP ( 'NONE', ( #17321, #14333 ) ) ;
#1038=CARTESIAN_POINT ( 'NONE',  ( -82.95659350918997177, 142.5787592618052315, 15.67196037041395229 ) ) ;
#1044=VERTEX_POINT ( 'NONE', #16092 ) ;
#1045=DIRECTION ( 'NONE',  ( -0.000000000000000000, -0.000000000000000000, 1.000000000000000000 ) ) ;
#1046=CARTESIAN_POINT ( 'NONE',  ( -96.00000000000001421, 171.6227766016838245, 0.000000000000000000 ) ) ;
#1048=B_SPLINE_CURVE_WITH_KNOTS ( 'NONE', 3,
 ( #12094, #12187, #1202, #6519, #10675, #4125, #1292, #10927, #56, #16350, #4049, #11910, #9347, #7932, #5456, #17316, #14830, #4218, #5184, #6605, #17502, #15985 ),
 .UNSPECIFIED., .F., .F.,
 ( 4, 2, 2, 2, 2, 2, 2, 2, 2, 2, 4 ),
 ( 0.000000000000000000, 0.002375333402909271790, 0.004750666805818540978, 0.007126000208727810599, 0.009501333611637081955, 0.01068900031309169378, 0.01187666701454630908, 0.01425200041745553273, 0.01543966711891012200, 0.01662733382036471128, 0.01900266722327392452 ),
 .UNSPECIFIED. ) ;
#1050=ORIENTED_EDGE ( 'NONE', *, *, #14204, .T. ) ;
#1051=DIRECTION ( 'NONE',  ( -1.000000000000000000, -0.000000000000000000, -0.000000000000000000 ) ) ;
#1052=EDGE_CURVE ( 'NONE', #16728, #16016, #10683, .T. ) ;
#1056=DIRECTION ( 'NONE',  ( 0.000000000000000000, -1.000000000000000000, 7.341990890863118602E-16 ) ) ;
#1059=ORIENTED_EDGE ( 'NONE', *, *, #1533, .T. ) ;
#1061=CARTESIAN_POINT ( 'NONE',  ( -43.00000000000000000, 130.0000000000000000, 15.00000000000000000 ) ) ;
#1063=CARTESIAN_POINT ( 'NONE',  ( -90.80384757729339640, 204.6227766016838245, 0.000000000000000000 ) ) ;
#1066=DIRECTION ( 'NONE',  ( -1.000000000000000000, 0.000000000000000000, 0.000000000000000000 ) ) ;
#1069=CARTESIAN_POINT ( 'NONE',  ( -725.0000000000000000, 19.99999999999995737, 13.00000000000000000 ) ) ;
#1073=CYLINDRICAL_SURFACE ( 'NONE', #5904, 9.999999999999994671 ) ;
#1074=VERTEX_POINT ( 'NONE', #5461 ) ;
#1075=EDGE_CURVE ( 'NONE', #1461, #805, #9519, .T. ) ;
#1080=CARTESIAN_POINT ( 'NONE',  ( 26.57417986947462651, 139.5089559931849692, 7.600184560211070917 ) ) ;
#1082=VECTOR ( 'NONE', #2070, 1000.000000000000000 ) ;
#1085=ORIENTED_EDGE ( 'NONE', *, *, #3481, .T. ) ;
#1087=CARTESIAN_POINT ( 'NONE',  ( -45.00000000000000000, 171.6227766016838245, 0.000000000000000000 ) ) ;
#1090=ORIENTED_EDGE ( 'NONE', *, *, #11674, .T. ) ;
#1099=ORIENTED_EDGE ( 'NONE', *, *, #6963, .F. ) ;
#1103=EDGE_CURVE ( 'NONE', #1074, #16221, #15014, .T. ) ;
#1104=VECTOR ( 'NONE', #1505, 1000.000000000000000 ) ;
#1107=VECTOR ( 'NONE', #12507, 1000.000000000000000 ) ;
#1108=CARTESIAN_POINT ( 'NONE',  ( -12.31336727611479631, 31.57746213708666971, 11.68681022658133806 ) ) ;
#1109=AXIS2_PLACEMENT_3D ( 'NONE', #12893, #768, #9885 ) ;
#1112=CARTESIAN_POINT ( 'NONE',  ( 20.95008785553089581, 29.88049067427350280, 10.28044474760307914 ) ) ;
#1113=CARTESIAN_POINT ( 'NONE',  ( -84.53126297072897444, 148.7415597018667199, 23.77993541092453000 ) ) ;
#1115=DIRECTION ( 'NONE',  ( -1.000000000000000000, 0.000000000000000000, -8.673617379884037937E-17 ) ) ;
#1117=LINE ( 'NONE', #9603, #8779 ) ;
#1118=CARTESIAN_POINT ( 'NONE',  ( 17.55923266082603007, 17.99999999999999645, 24.87049340120105612 ) ) ;
#1120=ORIENTED_EDGE ( 'NONE', *, *, #16638, .T. ) ;
#1124=AXIS2_PLACEMENT_3D ( 'NONE', #7031, #4466, #16505 ) ;
#1130=VERTEX_POINT ( 'NONE', #142 ) ;
#1136=CARTESIAN_POINT ( 'NONE',  ( -34.99999999999999289, 130.0000000000000000, 15.00000000000000000 ) ) ;
#1141=DIRECTION ( 'NONE',  ( -0.000000000000000000, -0.000000000000000000, -1.000000000000000000 ) ) ;
#1144=DIRECTION ( 'NONE',  ( -1.000000000000000000, -0.000000000000000000, -0.000000000000000000 ) ) ;
#1145=ORIENTED_EDGE ( 'NONE', *, *, #11841, .F. ) ;
#1150=CARTESIAN_POINT ( 'NONE',  ( 34.93420767853316988, 18.00000000000000355, 0.000000000000000000 ) ) ;
#1151=CARTESIAN_POINT ( 'NONE',  ( 49.99999999999998579, 163.6227766016838530, 12.50000337241049309 ) ) ;
#1152=DIRECTION ( 'NONE',  ( -1.000000000000000000, -0.000000000000000000, -0.000000000000000000 ) ) ;
#1154=DIRECTION ( 'NONE',  ( 1.000000000000000000, 0.000000000000000000, 0.000000000000000000 ) ) ;
#1157=AXIS2_PLACEMENT_3D ( 'NONE', #9341, #15001, #16173 ) ;
#1158=CARTESIAN_POINT ( 'NONE',  ( -16.30611068361784532, 32.76923076923076650, 4.999999999999998224 ) ) ;
#1164=VERTEX_POINT ( 'NONE', #10039 ) ;
#1165=LINE ( 'NONE', #11957, #3637 ) ;
#1171=DIRECTION ( 'NONE',  ( -1.156482317317868274E-16, 1.000000000000000000, 0.000000000000000000 ) ) ;
#1172=CARTESIAN_POINT ( 'NONE',  ( 18.85693063297101801, 142.3798671548016159, 15.29581099734062022 ) ) ;
#1175=ORIENTED_EDGE ( 'NONE', *, *, #17079, .T. ) ;
#1178=CYLINDRICAL_SURFACE ( 'NONE', #9082, 2.500000000000000444 ) ;
#1180=ORIENTED_EDGE ( 'NONE', *, *, #2081, .F. ) ;
#1181=DIRECTION ( 'NONE',  ( -1.000000000000000000, -6.938893903907228378E-16, 0.000000000000000000 ) ) ;
#1182=ORIENTED_EDGE ( 'NONE', *, *, #17382, .T. ) ;
#1186=ORIENTED_EDGE ( 'NONE', *, *, #14469, .T. ) ;
#1189=ORIENTED_EDGE ( 'NONE', *, *, #10276, .T. ) ;
#1191=ADVANCED_FACE ( 'NONE', ( #911 ), #322, .T. ) ;
#1193=EDGE_CURVE ( 'NONE', #16427, #7978, #1741, .T. ) ;
#1198=CARTESIAN_POINT ( 'NONE',  ( -75.46486027377252981, 148.7497411309094844, 23.78985390322973714 ) ) ;
#1199=VERTEX_POINT ( 'NONE', #3236 ) ;
#1201=DIRECTION ( 'NONE',  ( 1.000000000000000000, -0.000000000000000000, -0.000000000000000000 ) ) ;
#1202=CARTESIAN_POINT ( 'NONE',  ( 17.39133856982844506, 125.9242906883583970, 6.521754810248964418 ) ) ;
#1207=CARTESIAN_POINT ( 'NONE',  ( 29.50744102577957761, 201.5998317580112200, 13.79770299781523413 ) ) ;
#1215=AXIS2_PLACEMENT_3D ( 'NONE', #10912, #3879, #6436 ) ;
#1218=CARTESIAN_POINT ( 'NONE',  ( -12.63167751028161589, 20.00000000000000355, 24.35243221814332060 ) ) ;
#1220=CARTESIAN_POINT ( 'NONE',  ( -40.00000000000000000, 4.000000000000000000, 30.00000000000000711 ) ) ;
#1222=DIRECTION ( 'NONE',  ( 0.000000000000000000, 0.000000000000000000, -1.000000000000000000 ) ) ;
#1224=ADVANCED_FACE ( 'NONE', ( #3655 ), #8591, .T. ) ;
#1227=VERTEX_POINT ( 'NONE', #10461 ) ;
#1230=LINE ( 'NONE', #13183, #8950 ) ;
#1233=EDGE_CURVE ( 'NONE', #8974, #10007, #14992, .T. ) ;
#1234=CARTESIAN_POINT ( 'NONE',  ( 49.99999999999998579, 183.6227766016837961, 5.571800142134975431 ) ) ;
#1237=CARTESIAN_POINT ( 'NONE',  ( -38.00000000000000000, 2.000000000000000000, 0.000000000000000000 ) ) ;
#1238=LINE ( 'NONE', #9294, #4157 ) ;
#1249=CARTESIAN_POINT ( 'NONE',  ( -40.00000000000000000, 0.000000000000000000, 30.00000000000000355 ) ) ;
#1251=CARTESIAN_POINT ( 'NONE',  ( -10.84365596476886395, 30.77158821550125722, 14.49076147631418721 ) ) ;
#1252=CARTESIAN_POINT ( 'NONE',  ( 15.56337975240378846, 125.2134999403455851, 5.000000000000001776 ) ) ;
#1257=EDGE_CURVE ( 'NONE', #4434, #6774, #2765, .T. ) ;
#1266=CARTESIAN_POINT ( 'NONE',  ( 31.88903224608757014, 151.2561509761041521, 25.96550485207007242 ) ) ;
#1267=ORIENTED_EDGE ( 'NONE', *, *, #10879, .F. ) ;
#1269=CARTESIAN_POINT ( 'NONE',  ( 6.134011831684059501, 134.2062027339443944, 24.99999999999999645 ) ) ;
#1271=VECTOR ( 'NONE', #13608, 1000.000000000000000 ) ;
#1274=ORIENTED_EDGE ( 'NONE', *, *, #7864, .F. ) ;
#1276=ADVANCED_FACE ( 'NONE', ( #8318 ), #3109, .F. ) ;
#1277=DIRECTION ( 'NONE',  ( 0.000000000000000000, 0.000000000000000000, -1.000000000000000000 ) ) ;
#1282=PLANE ( 'NONE',  #4700 ) ;
#1287=CIRCLE ( 'NONE', #12024, 33.00000000000000000 ) ;
#1288=ORIENTED_EDGE ( 'NONE', *, *, #2762, .F. ) ;
#1289=CARTESIAN_POINT ( 'NONE',  ( -95.00000000000000000, 141.6227766016838245, -5.510910596163088767E-15 ) ) ;
#1292=CARTESIAN_POINT ( 'NONE',  ( 15.65639489742288681, 128.1581396164810940, 10.28488489824641761 ) ) ;
#1293=CARTESIAN_POINT ( 'NONE',  ( 24.94691999498327206, 18.00000000000000711, 22.32501294936691139 ) ) ;
#1301=VERTEX_POINT ( 'NONE', #12231 ) ;
#1303=EDGE_LOOP ( 'NONE', ( #11441, #8846, #10583, #13960 ) ) ;
#1305=CARTESIAN_POINT ( 'NONE',  ( -40.00000000000000000, 4.000000000000000000, 33.00000000000000711 ) ) ;
#1312=CARTESIAN_POINT ( 'NONE',  ( 25.49999999999998579, 9.999999999999998224, 0.000000000000000000 ) ) ;
#1313=DIRECTION ( 'NONE',  ( 1.000000000000000000, 0.000000000000000000, 0.000000000000000000 ) ) ;
#1316=ORIENTED_EDGE ( 'NONE', *, *, #2532, .T. ) ;
#1321=VECTOR ( 'NONE', #8240, 1000.000000000000000 ) ;
#1323=VECTOR ( 'NONE', #16410, 1000.000000000000000 ) ;
#1325=DIRECTION ( 'NONE',  ( 0.000000000000000000, 0.000000000000000000, 1.000000000000000000 ) ) ;
#1326=AXIS2_PLACEMENT_3D ( 'NONE', #7125, #1990, #12349 ) ;
#1329=EDGE_CURVE ( 'NONE', #16720, #11161, #11838, .T. ) ;
#1333=DIRECTION ( 'NONE',  ( -0.000000000000000000, -0.000000000000000000, -1.000000000000000000 ) ) ;
#1337=DIRECTION ( 'NONE',  ( -0.000000000000000000, -0.000000000000000000, -1.000000000000000000 ) ) ;
#1339=AXIS2_PLACEMENT_3D ( 'NONE', #16014, #2207, #14432 ) ;
#1344=ORIENTED_EDGE ( 'NONE', *, *, #16537, .T. ) ;
#1348=LINE ( 'NONE', #12051, #466 ) ;
#1349=VERTEX_POINT ( 'NONE', #6910 ) ;
#1350=CARTESIAN_POINT ( 'NONE',  ( -12.14981508666162036, 19.99999999999543121, 12.53017279448777366 ) ) ;
#1356=CYLINDRICAL_SURFACE ( 'NONE', #8665, 27.69059892324149530 ) ;
#1359=DIRECTION ( 'NONE',  ( -1.000000000000000000, 0.000000000000000000, 0.000000000000000000 ) ) ;
#1361=CARTESIAN_POINT ( 'NONE',  ( 29.00744693363358806, 151.5270838226223873, 26.17568438743891335 ) ) ;
#1365=DIRECTION ( 'NONE',  ( -1.000000000000000000, 0.000000000000000000, 0.000000000000000000 ) ) ;
#1366=( BOUNDED_SURFACE ( )  B_SPLINE_SURFACE ( 3, 2, ( 
 ( #1877, #551, #4626 ),
 ( #10001, #15412, #17087 ),
 ( #2309, #9116, #15760 ),
 ( #11605, #6287, #725 ),
 ( #7615, #12844, #11514 ),
 ( #11678, #5050, #3550 ),
 ( #14188, #814, #12937 ),
 ( #6032, #8935, #7699 ),
 ( #13106, #15505, #13029 ),
 ( #3382, #11426, #973 ),
 ( #6373, #11768, #10352 ),
 ( #15857, #14350, #900 ),
 ( #2049, #16835, #7528 ),
 ( #16926, #3642, #6208 ),
 ( #3730, #2127, #17011 ),
 ( #10266, #4959, #4877 ),
 ( #9032, #639, #8853 ),
 ( #4707, #17178, #10190 ),
 ( #14261, #2218, #10448 ),
 ( #14443, #4798, #1963 ),
 ( #7367, #15668, #15591 ),
 ( #12768, #10097, #3466 ),
 ( #7442, #8780, #6118 ),
 ( #13374, #13554, #1158 ) ),
 .UNSPECIFIED., .F., .F., .F. ) 
 B_SPLINE_SURFACE_WITH_KNOTS ( ( 4, 2, 2, 2, 2, 2, 2, 2, 2, 2, 2, 4 ),
 ( 3, 3 ),
 ( 0.01427588378380421734, 0.01824401167166928364, 0.02022807561560181766, 0.02221213955953435168, 0.02618026744739941625, 0.02816433139133195027, 0.03014839533526448428, 0.03411652322312955232, 0.03610058716706208287, 0.03808465111099461342, 0.04205277899885968146, 0.04602090688672474950 ),
 ( 0.000000000000000000, 1.000000000000000000 ),
 .UNSPECIFIED. ) 
 GEOMETRIC_REPRESENTATION_ITEM ( )  RATIONAL_B_SPLINE_SURFACE ( (
 ( 1.000000000000000000, 0.7071067811865476838, 1.000000000000000000),
 ( 1.000000000000000000, 0.7013659285812973154, 1.000000000000000000),
 ( 1.000000000000000000, 0.6957352470445186121, 1.000000000000000000),
 ( 1.000000000000000000, 0.6874449304734518984, 1.000000000000000000),
 ( 1.000000000000000000, 0.6847075230360146758, 1.000000000000000000),
 ( 1.000000000000000000, 0.6792848743381181276, 1.000000000000000000),
 ( 1.000000000000000000, 0.6765866164120997173, 1.000000000000000000),
 ( 1.000000000000000000, 0.6687223666255138754, 1.000000000000000000),
 ( 1.000000000000000000, 0.6637534122519734847, 1.000000000000000000),
 ( 1.000000000000000000, 0.6567012635109988894, 1.000000000000000000),
 ( 1.000000000000000000, 0.6544178910916050862, 1.000000000000000000),
 ( 1.000000000000000000, 0.6499901663948596253, 1.000000000000000000),
 ( 1.000000000000000000, 0.6478648508490586488, 1.000000000000000000),
 ( 1.000000000000000000, 0.6418284244075036504, 1.000000000000000000),
 ( 1.000000000000000000, 0.6382188548936987837, 1.000000000000000000),
 ( 1.000000000000000000, 0.6334349500989925330, 1.000000000000000000),
 ( 1.000000000000000000, 0.6319385063093012622, 1.000000000000000000),
 ( 1.000000000000000000, 0.6292162870120669993, 1.000000000000000000),
 ( 1.000000000000000000, 0.6279881568153810045, 1.000000000000000000),
 ( 1.000000000000000000, 0.6246939197237914021, 1.000000000000000000),
 ( 1.000000000000000000, 0.6230139244306683866, 1.000000000000000000),
 ( 1.000000000000000000, 0.6207349535630238835, 1.000000000000000000),
 ( 1.000000000000000000, 0.6201739322038456459, 1.000000000000000000),
 ( 1.000000000000000000, 0.6201736729460424202, 1.000000000000000000) ) ) 
 REPRESENTATION_ITEM ( '' )  SURFACE ( )  );
#1369=ORIENTED_EDGE ( 'NONE', *, *, #3514, .F. ) ;
#1370=EDGE_LOOP ( 'NONE', ( #2054, #9589, #12874, #6617, #1090, #12711, #3516 ) ) ;
#1373=CARTESIAN_POINT ( 'NONE',  ( 12.56741672263968290, 142.0153054307823481, 18.66563201629009328 ) ) ;
#1377=DIRECTION ( 'NONE',  ( 0.000000000000000000, 0.000000000000000000, -1.000000000000000000 ) ) ;
#1379=DIRECTION ( 'NONE',  ( 0.000000000000000000, 1.000000000000000000, 0.000000000000000000 ) ) ;
#1380=DIRECTION ( 'NONE',  ( 0.000000000000000000, 0.000000000000000000, -1.000000000000000000 ) ) ;
#1381=AXIS2_PLACEMENT_3D ( 'NONE', #2085, #3164, #6248 ) ;
#1382=ORIENTED_EDGE ( 'NONE', *, *, #14861, .F. ) ;
#1388=CARTESIAN_POINT ( 'NONE',  ( 14.93242934743711992, 18.00000000000000355, 25.00000000000000000 ) ) ;
#1390=FACE_OUTER_BOUND ( 'NONE', #16381, .T. ) ;
#1391=AXIS2_PLACEMENT_3D ( 'NONE', #9461, #9297, #14520 ) ;
#1397=ORIENTED_EDGE ( 'NONE', *, *, #15063, .T. ) ;
#1399=CARTESIAN_POINT ( 'NONE',  ( -85.00000000000007105, 146.0036328918051254, 20.82208359987473401 ) ) ;
#1402=DIRECTION ( 'NONE',  ( -1.000000000000000000, 0.000000000000000000, 0.000000000000000000 ) ) ;
#1403=ORIENTED_EDGE ( 'NONE', *, *, #4744, .T. ) ;
#1404=FACE_OUTER_BOUND ( 'NONE', #12164, .T. ) ;
#1405=CIRCLE ( 'NONE', #11292, 2.499999999999998668 ) ;
#1406=AXIS2_PLACEMENT_3D ( 'NONE', #10309, #6169, #7577 ) ;
#1407=DIRECTION ( 'NONE',  ( -2.674902700537819740E-31, 2.312964634635742267E-15, 1.000000000000000000 ) ) ;
#1408=CIRCLE ( 'NONE', #2527, 2.500000000000000444 ) ;
#1414=CARTESIAN_POINT ( 'NONE',  ( 48.00000000000000000, 171.6227766016838245, 0.000000000000000000 ) ) ;
#1418=ORIENTED_EDGE ( 'NONE', *, *, #10636, .F. ) ;
#1431=ORIENTED_EDGE ( 'NONE', *, *, #12069, .F. ) ;
#1435=EDGE_LOOP ( 'NONE', ( #16840, #13854, #4027, #12176 ) ) ;
#1436=CARTESIAN_POINT ( 'NONE',  ( 37.99999999999998579, 20.00000000000000000, 30.00000000000001066 ) ) ;
#1437=CONICAL_SURFACE ( 'NONE', #13880, 2.499999999999998668, 1.029744260000002187 ) ;
#1438=EDGE_CURVE ( 'NONE', #1227, #11461, #1405, .T. ) ;
#1439=ORIENTED_EDGE ( 'NONE', *, *, #968, .T. ) ;
#1442=ORIENTED_EDGE ( 'NONE', *, *, #3814, .T. ) ;
#1444=CIRCLE ( 'NONE', #11332, 5.000000000000004441 ) ;
#1449=ORIENTED_EDGE ( 'NONE', *, *, #16449, .F. ) ;
#1452=CARTESIAN_POINT ( 'NONE',  ( -45.00000000000000000, 120.0000000000000142, 15.00000000000000000 ) ) ;
#1456=CARTESIAN_POINT ( 'NONE',  ( -38.00000000000000000, 2.000000000000000000, 28.00000000000000355 ) ) ;
#1459=DIRECTION ( 'NONE',  ( 0.000000000000000000, 0.000000000000000000, -1.000000000000000000 ) ) ;
#1461=VERTEX_POINT ( 'NONE', #7436 ) ;
#1462=DIRECTION ( 'NONE',  ( 0.000000000000000000, 0.000000000000000000, -1.000000000000000000 ) ) ;
#1466=CARTESIAN_POINT ( 'NONE',  ( 40.00000000000000711, 136.6227766016838245, 0.000000000000000000 ) ) ;
#1471=CARTESIAN_POINT ( 'NONE',  ( -84.24740733152653149, 149.2783667126899445, 24.28707720053398944 ) ) ;
#1472=ORIENTED_EDGE ( 'NONE', *, *, #1487, .T. ) ;
#1473=( BOUNDED_SURFACE ( )  B_SPLINE_SURFACE ( 3, 2, ( 
 ( #15073, #11091, #5618 ),
 ( #212, #9763, #8612 ),
 ( #13759, #380, #4554 ),
 ( #14023, #9853, #7285 ) ),
 .UNSPECIFIED., .F., .F., .F. ) 
 B_SPLINE_SURFACE_WITH_KNOTS ( ( 4, 4 ),
 ( 3, 3 ),
 ( 0.1516087691302827056, 0.1566150273425061523 ),
 ( 0.000000000000000000, 1.000000000000000000 ),
 .UNSPECIFIED. ) 
 GEOMETRIC_REPRESENTATION_ITEM ( )  RATIONAL_B_SPLINE_SURFACE ( (
 ( 1.000000000000000000, 0.6556320892438534109, 1.000000000000000000),
 ( 1.000000000000000000, 0.6556321914870764100, 1.000000000000000000),
 ( 1.000000000000000000, 0.6556957163104859543, 1.000000000000000000),
 ( 1.000000000000000000, 0.6558243695371223092, 1.000000000000000000) ) ) 
 REPRESENTATION_ITEM ( '' )  SURFACE ( )  );
#1477=FACE_OUTER_BOUND ( 'NONE', #237, .T. ) ;
#1480=CARTESIAN_POINT ( 'NONE',  ( 196.0000000000000000, 163.6227766016838530, 10.00000337241049309 ) ) ;
#1482=CARTESIAN_POINT ( 'NONE',  ( -77.50000000000001421, 196.6227766016838245, 10.00000000000000178 ) ) ;
#1487=EDGE_CURVE ( 'NONE', #3421, #15746, #11599, .T. ) ;
#1488=CARTESIAN_POINT ( 'NONE',  ( 49.99999999999998579, 171.6227766016838245, 12.50000337241049131 ) ) ;
#1492=FACE_OUTER_BOUND ( 'NONE', #8201, .T. ) ;
#1496=ORIENTED_EDGE ( 'NONE', *, *, #10090, .T. ) ;
#1502=CARTESIAN_POINT ( 'NONE',  ( 27.13113508426156173, 192.5125816722295156, 25.54797519334865896 ) ) ;
#1503=DIRECTION ( 'NONE',  ( -1.000000000000000000, -6.938893903907228378E-16, -0.000000000000000000 ) ) ;
#1505=DIRECTION ( 'NONE',  ( -0.000000000000000000, -0.000000000000000000, -1.000000000000000000 ) ) ;
#1508=ORIENTED_EDGE ( 'NONE', *, *, #174, .T. ) ;
#1512=CARTESIAN_POINT ( 'NONE',  ( 27.99999999999998224, 9.999999999999998224, 0.000000000000000000 ) ) ;
#1513=ORIENTED_EDGE ( 'NONE', *, *, #15423, .T. ) ;
#1514=EDGE_CURVE ( 'NONE', #12210, #16876, #12837, .T. ) ;
#1515=CARTESIAN_POINT ( 'NONE',  ( -27.84784281930893357, 19.99999999999999645, 7.647248539284095870 ) ) ;
#1519=ORIENTED_EDGE ( 'NONE', *, *, #9584, .F. ) ;
#1520=LINE ( 'NONE', #2601, #13482 ) ;
#1521=LINE ( 'NONE', #13740, #16390 ) ;
#1527=ORIENTED_EDGE ( 'NONE', *, *, #15762, .F. ) ;
#1529=CARTESIAN_POINT ( 'NONE',  ( -23.00000000000000000, 122.0000000000000284, 15.00000000000000000 ) ) ;
#1533=EDGE_CURVE ( 'NONE', #4748, #5251, #15321, .T. ) ;
#1537=CARTESIAN_POINT ( 'NONE',  ( 11.58137902169779920, 142.1604892273610687, 18.89461017025931966 ) ) ;
#1541=DIRECTION ( 'NONE',  ( 1.000000000000000000, 0.000000000000000000, -0.000000000000000000 ) ) ;
#1542=ADVANCED_FACE ( 'NONE', ( #1869 ), #4791, .F. ) ;
#1544=EDGE_CURVE ( 'NONE', #3796, #17220, #2987, .T. ) ;
#1545=FACE_OUTER_BOUND ( 'NONE', #435, .T. ) ;
#1547=LINE ( 'NONE', #5180, #15428 ) ;
#1548=AXIS2_PLACEMENT_3D ( 'NONE', #901, #2310, #7701 ) ;
#1549=ORIENTED_EDGE ( 'NONE', *, *, #279, .F. ) ;
#1551=AXIS2_PLACEMENT_3D ( 'NONE', #11, #2488, #8234 ) ;
#1554=DIRECTION ( 'NONE',  ( -1.000000000000000000, -0.000000000000000000, -0.000000000000000000 ) ) ;
#1563=LINE ( 'NONE', #15191, #7080 ) ;
#1576=AXIS2_PLACEMENT_3D ( 'NONE', #14573, #2356, #8015 ) ;
#1577=VECTOR ( 'NONE', #9354, 1000.000000000000000 ) ;
#1583=VERTEX_POINT ( 'NONE', #10868 ) ;
#1590=DIRECTION ( 'NONE',  ( -0.000000000000000000, 0.000000000000000000, -1.000000000000000000 ) ) ;
#1592=CARTESIAN_POINT ( 'NONE',  ( 21.29916379186985154, 29.87370047437059384, 9.875089623381150261 ) ) ;
#1593=CARTESIAN_POINT ( 'NONE',  ( -45.00000000000000000, 134.2062027339443944, 25.00000000000000000 ) ) ;
#1598=EDGE_CURVE ( 'NONE', #5268, #5255, #15155, .T. ) ;
#1601=EDGE_CURVE ( 'NONE', #647, #15581, #1677, .T. ) ;
#1603=CIRCLE ( 'NONE', #9796, 20.00000000000000355 ) ;
#1618=FACE_OUTER_BOUND ( 'NONE', #10580, .T. ) ;
#1623=CARTESIAN_POINT ( 'NONE',  ( 49.99999999999998579, 151.6227766016839098, 5.571800142134973655 ) ) ;
#1628=EDGE_LOOP ( 'NONE', ( #8218, #8255, #7962, #5508 ) ) ;
#1630=CARTESIAN_POINT ( 'NONE',  ( -100.0000000000000000, 136.6227766016838245, 0.000000000000000000 ) ) ;
#1632=CARTESIAN_POINT ( 'NONE',  ( -48.00000000000000000, 171.6227766016838245, 20.00000000000000355 ) ) ;
#1634=CARTESIAN_POINT ( 'NONE',  ( 13.88882648224844907, 138.0291231684843751, 11.40862608215693008 ) ) ;
#1635=AXIS2_PLACEMENT_3D ( 'NONE', #14995, #2869, #1277 ) ;
#1636=ORIENTED_EDGE ( 'NONE', *, *, #12412, .T. ) ;
#1638=CARTESIAN_POINT ( 'NONE',  ( 40.00000000000000711, 171.6227766016838245, 0.000000000000000000 ) ) ;
#1641=FACE_OUTER_BOUND ( 'NONE', #10671, .T. ) ;
#1643=ORIENTED_EDGE ( 'NONE', *, *, #16262, .F. ) ;
#1645=AXIS2_PLACEMENT_3D ( 'NONE', #1452, #13317, #1181 ) ;
#1646=CARTESIAN_POINT ( 'NONE',  ( 34.93420767853316988, 30.00000000000000000, 0.000000000000000000 ) ) ;
#1650=CARTESIAN_POINT ( 'NONE',  ( 32.50000000000000000, 196.6227766016838245, 10.00000000000000178 ) ) ;
#1654=VERTEX_POINT ( 'NONE', #16205 ) ;
#1657=DIRECTION ( 'NONE',  ( 1.000000000000000000, 0.000000000000000000, 0.000000000000000000 ) ) ;
#1659=CARTESIAN_POINT ( 'NONE',  ( -45.00000000000000000, 130.0000000000000000, 0.000000000000000000 ) ) ;
#1666=EDGE_LOOP ( 'NONE', ( #926, #20 ) ) ;
#1667=DIRECTION ( 'NONE',  ( -1.000000000000000000, 0.000000000000000000, 0.000000000000000000 ) ) ;
#1675=ORIENTED_EDGE ( 'NONE', *, *, #5899, .T. ) ;
#1677=LINE ( 'NONE', #5658, #4973 ) ;
#1682=EDGE_CURVE ( 'NONE', #14446, #5655, #10962, .T. ) ;
#1686=CARTESIAN_POINT ( 'NONE',  ( -80.00000000000001421, 196.6227766016838245, 0.000000000000000000 ) ) ;
#1687=FACE_OUTER_BOUND ( 'NONE', #6399, .T. ) ;
#1689=CARTESIAN_POINT ( 'NONE',  ( -81.15920507698956499, 201.4909985710883404, 14.03234625026782645 ) ) ;
#1691=ORIENTED_EDGE ( 'NONE', *, *, #15361, .T. ) ;
#1695=PLANE ( 'NONE',  #2738 ) ;
#1697=CARTESIAN_POINT ( 'NONE',  ( -14.66060021943786751, 20.00000000000115818, 8.782938007015319570 ) ) ;
#1702=CARTESIAN_POINT ( 'NONE',  ( -10.03891356649073785, 18.00000000000000355, 24.87483525495233394 ) ) ;
#1704=EDGE_CURVE ( 'NONE', #11501, #11034, #7847, .T. ) ;
#1705=EDGE_CURVE ( 'NONE', #12616, #16016, #6950, .T. ) ;
#1708=CIRCLE ( 'NONE', #4246, 5.000000000000018652 ) ;
#1709=DIRECTION ( 'NONE',  ( -1.156482317317868274E-16, 1.000000000000000000, 0.000000000000000000 ) ) ;
#1723=LINE ( 'NONE', #1632, #8183 ) ;
#1724=CARTESIAN_POINT ( 'NONE',  ( 16.97810798871989135, 126.5456571586929044, 7.842726245482330327 ) ) ;
#1730=CARTESIAN_POINT ( 'NONE',  ( 18.93266870823487125, 29.92002005853035840, 11.93384102663519997 ) ) ;
#1738=CARTESIAN_POINT ( 'NONE',  ( 37.99999999999998579, 20.00000000000000000, 28.00000000000001066 ) ) ;
#1739=ORIENTED_EDGE ( 'NONE', *, *, #2762, .T. ) ;
#1741=LINE ( 'NONE', #5801, #6222 ) ;
#1742=ORIENTED_EDGE ( 'NONE', *, *, #3445, .F. ) ;
#1749=DIRECTION ( 'NONE',  ( -1.000000000000000000, 0.000000000000000000, 0.000000000000000000 ) ) ;
#1752=CARTESIAN_POINT ( 'NONE',  ( 31.13043979496999114, 141.7478424248371596, 14.01801864773823070 ) ) ;
#1753=DIRECTION ( 'NONE',  ( -0.000000000000000000, -0.000000000000000000, -1.000000000000000000 ) ) ;
#1754=DIRECTION ( 'NONE',  ( -1.156482317317868274E-16, 1.000000000000000000, 0.000000000000000000 ) ) ;
#1755=DIRECTION ( 'NONE',  ( 0.000000000000000000, 0.000000000000000000, -1.000000000000000000 ) ) ;
#1760=ORIENTED_EDGE ( 'NONE', *, *, #1075, .F. ) ;
#1763=DIRECTION ( 'NONE',  ( -0.000000000000000000, -0.000000000000000000, -1.000000000000000000 ) ) ;
#1765=CARTESIAN_POINT ( 'NONE',  ( 32.57588347945782914, 192.3210352480456891, 25.70268529851925265 ) ) ;
#1766=EDGE_CURVE ( 'NONE', #8027, #5289, #14022, .T. ) ;
#1771=CARTESIAN_POINT ( 'NONE',  ( -83.64566403027420449, 200.0568792608332558, 16.75365501014451297 ) ) ;
#1779=CARTESIAN_POINT ( 'NONE',  ( -25.81900932159183526, 19.99999999999999645, 13.95463872937544991 ) ) ;
#1782=PRODUCT ( 'Left Housing Shell', 'Left Housing Shell', '', ( #15076 ) ) ;
#1787=CARTESIAN_POINT ( 'NONE',  ( -24.99999999999999645, 120.0000000000000284, 15.00000000000000000 ) ) ;
#1790=ORIENTED_EDGE ( 'NONE', *, *, #15077, .T. ) ;
#1796=EDGE_CURVE ( 'NONE', #4487, #8664, #5540, .T. ) ;
#1798=ADVANCED_FACE ( 'NONE', ( #12354 ), #7047, .F. ) ;
#1802=CARTESIAN_POINT ( 'NONE',  ( 14.43747245749253416, 129.4010981426196736, 11.63709869316310908 ) ) ;
#1808=CARTESIAN_POINT ( 'NONE',  ( 18.47042353409679194, 29.92915261368834479, 12.18054208566702279 ) ) ;
#1816=AXIS2_PLACEMENT_3D ( 'NONE', #4935, #14324, #11582 ) ;
#1818=ORIENTED_EDGE ( 'NONE', *, *, #3538, .T. ) ;
#1819=EDGE_CURVE ( 'NONE', #2616, #2637, #12891, .T. ) ;
#1822=CARTESIAN_POINT ( 'NONE',  ( 6.134011831684059501, 134.2062027339443944, 13.00000000000000000 ) ) ;
#1824=ORIENTED_EDGE ( 'NONE', *, *, #17265, .F. ) ;
#1827=AXIS2_PLACEMENT_3D ( 'NONE', #10901, #9486, #1359 ) ;
#1828=CARTESIAN_POINT ( 'NONE',  ( 0.000000000000000000, 20.00000000000000000, 0.000000000000000000 ) ) ;
#1831=EDGE_LOOP ( 'NONE', ( #6276, #7051, #12, #6157 ) ) ;
#1835=ADVANCED_FACE ( 'NONE', ( #4126 ), #5632, .F. ) ;
#1838=DIRECTION ( 'NONE',  ( 1.000000000000000000, 0.000000000000000000, 0.000000000000000000 ) ) ;
#1841=CARTESIAN_POINT ( 'NONE',  ( 14.93242934743711992, 20.00000000000000000, 25.00000000000000000 ) ) ;
#1847=CARTESIAN_POINT ( 'NONE',  ( 48.00000000000000711, 179.6227766016838245, 10.00000337241049309 ) ) ;
#1848=CARTESIAN_POINT ( 'NONE',  ( 21.44211297938456084, 29.87092986353274426, 9.660732976998257726 ) ) ;
#1852=CARTESIAN_POINT ( 'NONE',  ( 15.98317902225257470, 29.97876603371781457, 12.94822346880645902 ) ) ;
#1854=CARTESIAN_POINT ( 'NONE',  ( -78.29008794608814981, 201.3251192758334582, 14.38044245167806423 ) ) ;
#1859=EDGE_CURVE ( 'NONE', #15841, #6861, #3373, .T. ) ;
#1860=ORIENTED_EDGE ( 'NONE', *, *, #2897, .F. ) ;
#1864=EDGE_LOOP ( 'NONE', ( #10980, #15166, #1947, #7705 ) ) ;
#1868=CLOSED_SHELL ( 'NONE', ( #6036, #7114, #11055, #5318, #17494, #5701, #5862, #391, #9641, #2040, #1798, #8408, #12670, #15046, #6749, #6790, #6995, #3837, #14323, #10466, #12178, #17096, #6391, #16760, #7971, #15007, #16774, #3602, #13406, #7593, #2605, #17289, #16476, #16402, #3138, #8922, #8192, #13603, #6578, #11483, #14202, #76, #3297, #15872, #10123, #5597, #13427, #4544, #10743, #540, #11103, #14161, #9647, #7625, #6284, #8136, #8266, #6925, #2131, #1542, #15587, #14762, #12845, #9828, #14511, #16386, #8426, #17332, #9333, #10127, #16315, #2168, #4742, #1191, #15446, #12099, #688, #1835, #4084, #11756, #5647, #15658, #16639, #14788, #15761, #14281, #8463, #5666, #14905, #12248, #7646, #13752, #14715, #16220, #1224, #2524, #4529, #9748, #12628, #5386, #792, #248, #3904, #4562, #13708, #4367, #13052, #7187, #11623, #16026, #6644, #5812, #12131, #10093, #3286, #13601, #13660, #10340, #13898, #7502, #17008, #14142, #10827, #6449, #8259, #3659, #4620, #5448, #16513, #1276, #12774, #12899, #7776, #17063, #12679, #17497, #11566, #4892, #3097, #9739, #8287, #13230, #16316, #14689, #9429, #882, #13111, #15835, #9703, #11699, #16619, #15517, #7312, #33, #6593, #11586, #12738, #5761, #522 ) ) ;
#1869=FACE_OUTER_BOUND ( 'NONE', #11982, .T. ) ;
#1870=CIRCLE ( 'NONE', #12604, 2.500000000000000444 ) ;
#1871=VERTEX_POINT ( 'NONE', #2360 ) ;
#1874=CARTESIAN_POINT ( 'NONE',  ( -7.379000772445021283, 18.00000000000000000, 25.00000000000000355 ) ) ;
#1875=FACE_OUTER_BOUND ( 'NONE', #4435, .T. ) ;
#1877=CARTESIAN_POINT ( 'NONE',  ( -7.379000772444995526, 18.00000000000000000, 25.00000000000000000 ) ) ;
#1879=AXIS2_PLACEMENT_3D ( 'NONE', #17279, #5151, #3919 ) ;
#1880=CARTESIAN_POINT ( 'NONE',  ( 48.00000000000000000, 171.6227766016838245, 15.00000337241049131 ) ) ;
#1884=ORIENTED_EDGE ( 'NONE', *, *, #9370, .T. ) ;
#1885=CARTESIAN_POINT ( 'NONE',  ( 27.48361012698968864, 136.6227766016838245, 0.000000000000000000 ) ) ;
#1886=CARTESIAN_POINT ( 'NONE',  ( 49.99999999999998579, 155.6227766016839098, 12.50000337241049309 ) ) ;
#1888=CARTESIAN_POINT ( 'NONE',  ( -50.00000000000000000, 154.3022685259950038, 9.999999999999900524 ) ) ;
#1889=CARTESIAN_POINT ( 'NONE',  ( 49.99999999999998579, 171.6227766016838245, 10.00000337241048953 ) ) ;
#1890=CARTESIAN_POINT ( 'NONE',  ( 17.19546515351294147, 126.2270863594749670, 7.189547039408070717 ) ) ;
#1892=EDGE_LOOP ( 'NONE', ( #13134, #12511 ) ) ;
#1898=DIRECTION ( 'NONE',  ( 0.000000000000000000, 0.000000000000000000, -1.000000000000000000 ) ) ;
#1900=CARTESIAN_POINT ( 'NONE',  ( 17.75267852353177034, 29.94338869414745830, 12.49131726690029254 ) ) ;
#1906=DIRECTION ( 'NONE',  ( 0.000000000000000000, 0.000000000000000000, -1.000000000000000000 ) ) ;
#1910=CARTESIAN_POINT ( 'NONE',  ( 10.58901158398830766, 139.9616134764785329, 11.54438095561596000 ) ) ;
#1916=CARTESIAN_POINT ( 'NONE',  ( 15.53715976346056493, 125.3980538582347748, 5.670872899454017180 ) ) ;
#1917=LINE ( 'NONE', #1828, #8747 ) ;
#1919=EDGE_CURVE ( 'NONE', #7945, #11482, #11675, .T. ) ;
#1923=AXIS2_PLACEMENT_3D ( 'NONE', #17345, #13283, #11944 ) ;
#1925=CARTESIAN_POINT ( 'NONE',  ( 25.53083208230110657, 144.3624319200458785, 18.60312384224725335 ) ) ;
#1926=LINE ( 'NONE', #14228, #557 ) ;
#1934=DIRECTION ( 'NONE',  ( -1.000000000000000000, 0.000000000000000000, 0.000000000000000000 ) ) ;
#1935=AXIS2_PLACEMENT_3D ( 'NONE', #13905, #1763, #7161 ) ;
#1936=ORIENTED_EDGE ( 'NONE', *, *, #13599, .F. ) ;
#1939=PLANE ( 'NONE',  #10931 ) ;
#1947=ORIENTED_EDGE ( 'NONE', *, *, #3864, .F. ) ;
#1956=AXIS2_PLACEMENT_3D ( 'NONE', #16087, #3964, #1906 ) ;
#1959=VECTOR ( 'NONE', #5162, 1000.000000000000000 ) ;
#1960=CARTESIAN_POINT ( 'NONE',  ( -14.54670497998689171, 17.99999999999999645, 23.76610458325318831 ) ) ;
#1961=CARTESIAN_POINT ( 'NONE',  ( -50.00000000000000000, 204.6227766016838245, -2.020667218593133100E-15 ) ) ;
#1963=CARTESIAN_POINT ( 'NONE',  ( -15.84134677353521070, 32.63429591450738343, 7.614689697697072823 ) ) ;
#1967=VERTEX_POINT ( 'NONE', #14492 ) ;
#1968=DIRECTION ( 'NONE',  ( -0.000000000000000000, -1.000000000000000000, -0.000000000000000000 ) ) ;
#1970=VECTOR ( 'NONE', #3890, 1000.000000000000000 ) ;
#1973=CIRCLE ( 'NONE', #8755, 5.000000000000000888 ) ;
#1974=DIRECTION ( 'NONE',  ( 0.000000000000000000, 0.000000000000000000, -1.000000000000000000 ) ) ;
#1976=CARTESIAN_POINT ( 'NONE',  ( 27.15273249069231198, 19.99999999999999645, 20.88767039909325973 ) ) ;
#1977=CARTESIAN_POINT ( 'NONE',  ( 21.59801423301730239, 20.00000000000000000, 12.60094170202890140 ) ) ;
#1980=VECTOR ( 'NONE', #3970, 1000.000000000000000 ) ;
#1986=CARTESIAN_POINT ( 'NONE',  ( -27.99999999999998224, 10.00000000000000000, 0.000000000000000000 ) ) ;
#1987=CARTESIAN_POINT ( 'NONE',  ( -79.59850409272017657, 191.6349927435749692, 26.23951396249187340 ) ) ;
#1989=CARTESIAN_POINT ( 'NONE',  ( -7.379000772444994638, 20.00000000000000000, 25.00000000000000000 ) ) ;
#1990=DIRECTION ( 'NONE',  ( -1.000000000000000000, -0.000000000000000000, -0.000000000000000000 ) ) ;
#1992=EDGE_CURVE ( 'NONE', #14157, #15093, #16951, .T. ) ;
#1993=EDGE_CURVE ( 'NONE', #17220, #3796, #3393, .T. ) ;
#2000=AXIS2_PLACEMENT_3D ( 'NONE', #12733, #11043, #8650 ) ;
#2003=EDGE_LOOP ( 'NONE', ( #342, #15510, #2783, #16048 ) ) ;
#2005=EDGE_CURVE ( 'NONE', #11482, #7945, #1973, .T. ) ;
#2006=ORIENTED_EDGE ( 'NONE', *, *, #3078, .T. ) ;
#2012=B_SPLINE_CURVE_WITH_KNOTS ( 'NONE', 3,
 ( #7126, #13437, #12202, #2462, #3047, #13264, #5392, #14768, #6624, #16106, #13354, #7949, #3982, #6715, #2725, #16192, #12114, #12015, #2559, #14844, #8452, #1218, #6809, #9272, #17418, #6539 ),
 .UNSPECIFIED., .F., .F.,
 ( 4, 2, 2, 2, 2, 2, 2, 2, 2, 2, 2, 2, 4 ),
 ( 0.000000000000000000, 0.002002783134349993537, 0.004005566268699987074, 0.008011132537399970679, 0.01001391567174996812, 0.01201669880609996383, 0.01602226507479994830, 0.01802504820914994227, 0.02002783134349994318, 0.02403339761219993459, 0.02603618074654993550, 0.02803896388089993641, 0.03204453014959993129 ),
 .UNSPECIFIED. ) ;
#2015=CARTESIAN_POINT ( 'NONE',  ( 34.86532646282766024, 145.4324535730256684, 20.08206597984641917 ) ) ;
#2017=FACE_BOUND ( 'NONE', #3086, .T. ) ;
#2026=ORIENTED_EDGE ( 'NONE', *, *, #9908, .T. ) ;
#2027=CARTESIAN_POINT ( 'NONE',  ( 27.41872110558518116, 136.9783011792879392, 5.130391642808777242 ) ) ;
#2032=DIRECTION ( 'NONE',  ( -1.000000000000000000, 0.000000000000000000, 0.000000000000000000 ) ) ;
#2040=ADVANCED_FACE ( 'NONE', ( #12516 ), #12338, .F. ) ;
#2041=ORIENTED_EDGE ( 'NONE', *, *, #7584, .T. ) ;
#2049=CARTESIAN_POINT ( 'NONE',  ( -21.36854569161881301, 18.00000000000000000, 19.70709815271291632 ) ) ;
#2053=CARTESIAN_POINT ( 'NONE',  ( 30.49999999999998224, 9.999999999999998224, 10.00000000000000178 ) ) ;
#2054=ORIENTED_EDGE ( 'NONE', *, *, #12667, .T. ) ;
#2060=CARTESIAN_POINT ( 'NONE',  ( 19.38030756396766563, 20.00000000000227018, 14.02844645440659654 ) ) ;
#2061=CARTESIAN_POINT ( 'NONE',  ( 17.03671980602049985, 126.4628225884666932, 7.681944018317823364 ) ) ;
#2062=VERTEX_POINT ( 'NONE', #1889 ) ;
#2063=DIRECTION ( 'NONE',  ( -1.000000000000000000, 0.000000000000000000, 0.000000000000000000 ) ) ;
#2064=CARTESIAN_POINT ( 'NONE',  ( -83.41681137195966755, 192.9554221994868044, 25.17938093289616575 ) ) ;
#2070=DIRECTION ( 'NONE',  ( -0.000000000000000000, -0.000000000000000000, -1.000000000000000000 ) ) ;
#2074=DIRECTION ( 'NONE',  ( -1.000000000000000000, -0.000000000000000000, -0.000000000000000000 ) ) ;
#2080=CARTESIAN_POINT ( 'NONE',  ( 30.00000000000000355, 196.6227766016838245, 10.00000000000000178 ) ) ;
#2081=EDGE_CURVE ( 'NONE', #14731, #11875, #1723, .T. ) ;
#2082=ORIENTED_EDGE ( 'NONE', *, *, #6415, .T. ) ;
#2084=CARTESIAN_POINT ( 'NONE',  ( 6.803110712587624676, 134.0269829078799262, 12.98040381008119759 ) ) ;
#2085=CARTESIAN_POINT ( 'NONE',  ( 49.99999999999998579, 155.6227766016839098, 12.50000337241049309 ) ) ;
#2086=CARTESIAN_POINT ( 'NONE',  ( 13.65319468154008042, 138.6827642936709424, 2.302653601763912761 ) ) ;
#2093=PLANE ( 'NONE',  #12038 ) ;
#2095=VERTEX_POINT ( 'NONE', #7116 ) ;
#2097=VECTOR ( 'NONE', #15350, 1000.000000000000000 ) ;
#2098=ORIENTED_EDGE ( 'NONE', *, *, #8388, .F. ) ;
#2105=DIRECTION ( 'NONE',  ( 0.000000000000000000, -1.000000000000000000, 0.000000000000000000 ) ) ;
#2106=CARTESIAN_POINT ( 'NONE',  ( -725.0000000000000000, 19.99999999999995737, 4.999999999999999112 ) ) ;
#2107=EDGE_CURVE ( 'NONE', #6775, #938, #14139, .T. ) ;
#2108=EDGE_CURVE ( 'NONE', #11290, #14157, #14407, .T. ) ;
#2116=CYLINDRICAL_SURFACE ( 'NONE', #9223, 750.0000000000001137 ) ;
#2117=EDGE_LOOP ( 'NONE', ( #2692, #12862 ) ) ;
#2118=CYLINDRICAL_SURFACE ( 'NONE', #8106, 5.000000000000004441 ) ;
#2122=VECTOR ( 'NONE', #14100, 1000.000000000000114 ) ;
#2127=CARTESIAN_POINT ( 'NONE',  ( -12.35971836118926959, 18.00000000000229861, 8.238707107740440350 ) ) ;
#2131=ADVANCED_FACE ( 'NONE', ( #11267 ), #1473, .F. ) ;
#2134=VERTEX_POINT ( 'NONE', #8529 ) ;
#2143=CARTESIAN_POINT ( 'NONE',  ( 33.66001102075547635, 19.99999999999999645, 12.05479157725600459 ) ) ;
#2146=DIRECTION ( 'NONE',  ( -1.000000000000000000, -0.000000000000000000, -0.000000000000000000 ) ) ;
#2148=CARTESIAN_POINT ( 'NONE',  ( -79.79487623779336047, 191.6231342001797771, 26.24853702829032542 ) ) ;
#2151=AXIS2_PLACEMENT_3D ( 'NONE', #14988, #10829, #1365 ) ;
#2153=ORIENTED_EDGE ( 'NONE', *, *, #13026, .T. ) ;
#2156=EDGE_LOOP ( 'NONE', ( #8329, #5068, #5967, #8726 ) ) ;
#2158=LINE ( 'NONE', #15696, #16584 ) ;
#2166=CIRCLE ( 'NONE', #14325, 747.9999999999998863 ) ;
#2168=ADVANCED_FACE ( 'NONE', ( #4811 ), #14803, .F. ) ;
#2169=CARTESIAN_POINT ( 'NONE',  ( -13.00560346926692645, 31.78932620563996281, 11.23370548922391521 ) ) ;
#2170=EDGE_CURVE ( 'NONE', #14731, #13379, #277, .T. ) ;
#2172=CARTESIAN_POINT ( 'NONE',  ( 49.99999999999998579, 183.6227766016837961, 5.571800142134975431 ) ) ;
#2180=CARTESIAN_POINT ( 'NONE',  ( 24.87028194210262910, 29.86925052300016858, 6.309743549972420595 ) ) ;
#2181=DIRECTION ( 'NONE',  ( 1.000000000000000000, 1.156482317317868274E-16, -0.000000000000000000 ) ) ;
#2183=CARTESIAN_POINT ( 'NONE',  ( 30.90732076053024002, 201.5450689758320095, 13.91624649103840206 ) ) ;
#2189=CIRCLE ( 'NONE', #16051, 20.00000000000000355 ) ;
#2192=AXIS2_PLACEMENT_3D ( 'NONE', #12032, #5215, #12128 ) ;
#2193=CARTESIAN_POINT ( 'NONE',  ( -34.99999999999999289, 120.0000000000000000, 0.000000000000000000 ) ) ;
#2194=DIRECTION ( 'NONE',  ( 0.000000000000000000, 1.000000000000000000, 0.000000000000000000 ) ) ;
#2201=ORIENTED_EDGE ( 'NONE', *, *, #520, .F. ) ;
#2203=ORIENTED_EDGE ( 'NONE', *, *, #12801, .F. ) ;
#2205=CIRCLE ( 'NONE', #12109, 10.00000000000000178 ) ;
#2207=DIRECTION ( 'NONE',  ( 0.000000000000000000, -1.000000000000000000, 0.000000000000000000 ) ) ;
#2209=DIRECTION ( 'NONE',  ( -1.000000000000000000, -0.000000000000000000, -0.000000000000000000 ) ) ;
#2211=VERTEX_POINT ( 'NONE', #6388 ) ;
#2217=CARTESIAN_POINT ( 'NONE',  ( -24.94987437106622252, 120.0000000000000284, 6.000000000000001776 ) ) ;
#2218=CARTESIAN_POINT ( 'NONE',  ( -12.66151707385296987, 17.99999999999770495, 6.998435355972849159 ) ) ;
#2220=CYLINDRICAL_SURFACE ( 'NONE', #16819, 250.0000000000000000 ) ;
#2224=EDGE_LOOP ( 'NONE', ( #692, #3818, #4573, #8253 ) ) ;
#2226=AXIS2_PLACEMENT_3D ( 'NONE', #15939, #7882, #17448 ) ;
#2230=ORIENTED_EDGE ( 'NONE', *, *, #15704, .T. ) ;
#2231=CARTESIAN_POINT ( 'NONE',  ( 24.94691999498327206, 20.00000000000000355, 22.32501294936691139 ) ) ;
#2232=AXIS2_PLACEMENT_3D ( 'NONE', #17127, #11810, #7925 ) ;
#2236=CARTESIAN_POINT ( 'NONE',  ( 30.80964797964808000, 19.99999999999999645, 17.18170494867160514 ) ) ;
#2238=ORIENTED_EDGE ( 'NONE', *, *, #12023, .F. ) ;
#2241=CIRCLE ( 'NONE', #7608, 2.499999999999998668 ) ;
#2245=ORIENTED_EDGE ( 'NONE', *, *, #12411, .F. ) ;
#2246=DIRECTION ( 'NONE',  ( -1.000000000000000000, -0.000000000000000000, -0.000000000000000000 ) ) ;
#2250=ORIENTED_EDGE ( 'NONE', *, *, #9908, .F. ) ;
#2251=ORIENTED_EDGE ( 'NONE', *, *, #4788, .T. ) ;
#2252=ORIENTED_EDGE ( 'NONE', *, *, #4685, .F. ) ;
#2259=CARTESIAN_POINT ( 'NONE',  ( -16.28901493728125160, 32.76428253546148284, 5.573780508339472028 ) ) ;
#2265=CARTESIAN_POINT ( 'NONE',  ( 26.66247177481912800, 139.4607352144954007, 7.398570892697257761 ) ) ;
#2268=CARTESIAN_POINT ( 'NONE',  ( -100.0000000000000000, 120.0000000000000284, 6.000000000000001776 ) ) ;
#2269=CARTESIAN_POINT ( 'NONE',  ( 196.0000000000000000, 167.6227766016838814, 19.42820660268601074 ) ) ;
#2270=CARTESIAN_POINT ( 'NONE',  ( 23.07174175064647059, 29.89240369784053897, 10.82181213433699618 ) ) ;
#2272=CARTESIAN_POINT ( 'NONE',  ( 39.99999999999998579, 4.000000000000000000, 30.00000000000001066 ) ) ;
#2274=CARTESIAN_POINT ( 'NONE',  ( 25.00000000000000355, 197.2415780845127244, 20.82248078717325157 ) ) ;
#2276=LINE ( 'NONE', #17413, #10935 ) ;
#2278=AXIS2_PLACEMENT_3D ( 'NONE', #6951, #14041, #13872 ) ;
#2280=CARTESIAN_POINT ( 'NONE',  ( -78.47034442031463186, 141.8580068101642553, 14.25043922611179248 ) ) ;
#2292=AXIS2_PLACEMENT_3D ( 'NONE', #10372, #2325, #14539 ) ;
#2302=CARTESIAN_POINT ( 'NONE',  ( -70.00000000000000000, 171.6227766016838245, 0.000000000000000000 ) ) ;
#2305=AXIS2_PLACEMENT_3D ( 'NONE', #16232, #4102, #9485 ) ;
#2306=CARTESIAN_POINT ( 'NONE',  ( 27.99999999999998224, 9.999999999999998224, 10.00000000000000178 ) ) ;
#2307=CARTESIAN_POINT ( 'NONE',  ( 196.0000000000000000, 183.6227766016837961, 8.071800142134975431 ) ) ;
#2309=CARTESIAN_POINT ( 'NONE',  ( -10.04118010627651181, 18.00000000000000000, 24.87462214922868142 ) ) ;
#2310=DIRECTION ( 'NONE',  ( -0.000000000000000000, -0.000000000000000000, -1.000000000000000000 ) ) ;
#2313=DIRECTION ( 'NONE',  ( -1.000000000000000000, -0.000000000000000000, -0.000000000000000000 ) ) ;
#2317=CARTESIAN_POINT ( 'NONE',  ( -38.00000000000000000, 2.000000000000000000, 0.000000000000000000 ) ) ;
#2319=CARTESIAN_POINT ( 'NONE',  ( -12.97728802729275088, 19.99999999999883826, 11.64645903342270827 ) ) ;
#2320=CARTESIAN_POINT ( 'NONE',  ( 10.61972500670372277, 131.6239249143206393, 11.92364046234351527 ) ) ;
#2321=CARTESIAN_POINT ( 'NONE',  ( 34.93420767853318409, 19.99999999999999645, 5.000000000000010658 ) ) ;
#2324=CARTESIAN_POINT ( 'NONE',  ( -100.0000000000000000, 144.1839557653416080, 18.33333333333335702 ) ) ;
#2325=DIRECTION ( 'NONE',  ( 0.000000000000000000, -0.4999999999999952816, -0.8660254037844413721 ) ) ;
#2327=ORIENTED_EDGE ( 'NONE', *, *, #3162, .F. ) ;
#2329=EDGE_CURVE ( 'NONE', #11846, #11660, #15586, .T. ) ;
#2331=EDGE_CURVE ( 'NONE', #9736, #4487, #9028, .T. ) ;
#2332=ORIENTED_EDGE ( 'NONE', *, *, #13564, .T. ) ;
#2334=DIRECTION ( 'NONE',  ( -1.000000000000000000, -0.000000000000000000, -0.000000000000000000 ) ) ;
#2335=ORIENTED_EDGE ( 'NONE', *, *, #14223, .T. ) ;
#2336=VERTEX_POINT ( 'NONE', #634 ) ;
#2341=CARTESIAN_POINT ( 'NONE',  ( -14.26174088910747706, 32.16828253888332512, 10.14247415352539683 ) ) ;
#2342=CARTESIAN_POINT ( 'NONE',  ( -9.725435201701724708, 30.52647059548997888, 14.77261045527475147 ) ) ;
#2344=CARTESIAN_POINT ( 'NONE',  ( 15.00000000000903455, 143.2885527162398489, 16.91661185963483760 ) ) ;
#2345=CARTESIAN_POINT ( 'NONE',  ( -100.0000000000000000, 143.0439382767972347, 16.49999999999984368 ) ) ;
#2346=ORIENTED_EDGE ( 'NONE', *, *, #1682, .F. ) ;
#2347=CARTESIAN_POINT ( 'NONE',  ( 24.75325409605274274, 140.3706687641101212, 10.61653890585399296 ) ) ;
#2352=CARTESIAN_POINT ( 'NONE',  ( 34.93420767853314146, 18.00000000000000355, 6.320602137672510779 ) ) ;
#2356=DIRECTION ( 'NONE',  ( 0.000000000000000000, 0.000000000000000000, -1.000000000000000000 ) ) ;
#2358=VERTEX_POINT ( 'NONE', #15756 ) ;
#2360=CARTESIAN_POINT ( 'NONE',  ( -70.00000000000000000, 191.6227766016837961, -1.224646799147353454E-15 ) ) ;
#2363=CARTESIAN_POINT ( 'NONE',  ( -81.72853406442757773, 141.9273338169157626, 14.39467838667816579 ) ) ;
#2366=EDGE_CURVE ( 'NONE', #938, #6775, #5074, .T. ) ;
#2367=CARTESIAN_POINT ( 'NONE',  ( -100.0000000000000000, 201.6227766016838245, 0.000000000000000000 ) ) ;
#2376=VECTOR ( 'NONE', #9308, 1000.000000000000000 ) ;
#2382=DIRECTION ( 'NONE',  ( 0.000000000000000000, 0.000000000000000000, -1.000000000000000000 ) ) ;
#2384=CARTESIAN_POINT ( 'NONE',  ( 34.53584570369260831, 194.4969340293141045, 23.78882387388086173 ) ) ;
#2386=LINE ( 'NONE', #15855, #5557 ) ;
#2388=LINE ( 'NONE', #7782, #12021 ) ;
#2390=AXIS2_PLACEMENT_3D ( 'NONE', #13418, #6695, #12090 ) ;
#2391=CARTESIAN_POINT ( 'NONE',  ( 27.48361012698979877, 126.6227766016837819, 9.278408830390956550E-15 ) ) ;
#2394=DIRECTION ( 'NONE',  ( -1.000000000000000000, 0.000000000000000000, 0.000000000000000000 ) ) ;
#2395=VERTEX_POINT ( 'NONE', #14002 ) ;
#2401=CARTESIAN_POINT ( 'NONE',  ( -7.379000772444995526, 20.00000000000000355, 15.00000000000000178 ) ) ;
#2402=CARTESIAN_POINT ( 'NONE',  ( 11.61604111307750209, 130.6582085322020532, 11.34316963496758390 ) ) ;
#2403=CIRCLE ( 'NONE', #6661, 2.500000000000002220 ) ;
#2406=DIRECTION ( 'NONE',  ( 0.000000000000000000, 0.000000000000000000, -1.000000000000000000 ) ) ;
#2408=ORIENTED_EDGE ( 'NONE', *, *, #13777, .T. ) ;
#2409=DIRECTION ( 'NONE',  ( 0.000000000000000000, 0.000000000000000000, -1.000000000000000000 ) ) ;
#2417=EDGE_LOOP ( 'NONE', ( #3578, #120, #11351, #6584 ) ) ;
#2419=DIRECTION ( 'NONE',  ( 0.000000000000000000, 0.000000000000000000, -1.000000000000000000 ) ) ;
#2422=ORIENTED_EDGE ( 'NONE', *, *, #1329, .F. ) ;
#2429=CIRCLE ( 'NONE', #8090, 5.000000000000000888 ) ;
#2430=CARTESIAN_POINT ( 'NONE',  ( -12.61248932541308676, 31.15232071419451643, 13.80069170922183375 ) ) ;
#2432=CARTESIAN_POINT ( 'NONE',  ( 21.38389869590487891, 18.00000000000114753, 9.948751090973035005 ) ) ;
#2434=CARTESIAN_POINT ( 'NONE',  ( -84.64785531711687838, 148.4718376841440204, 23.51742847763245337 ) ) ;
#2436=CARTESIAN_POINT ( 'NONE',  ( 17.57170338634705331, 142.7189882356449857, 15.92841986281182187 ) ) ;
#2438=CARTESIAN_POINT ( 'NONE',  ( 17.00000000000000000, 204.6227766016838245, -2.020667218593133100E-15 ) ) ;
#2439=CARTESIAN_POINT ( 'NONE',  ( 32.91012024024373517, 17.99999999999999645, 13.86436652238006673 ) ) ;
#2441=VERTEX_POINT ( 'NONE', #16830 ) ;
#2444=VECTOR ( 'NONE', #4957, 1000.000000000000000 ) ;
#2447=CARTESIAN_POINT ( 'NONE',  ( 32.94631475844272472, 200.6745000914694117, 15.65774685523815890 ) ) ;
#2451=ORIENTED_EDGE ( 'NONE', *, *, #1601, .T. ) ;
#2455=CARTESIAN_POINT ( 'NONE',  ( -24.99999999999999289, 100.0000000000000142, 15.00000000000000000 ) ) ;
#2462=CARTESIAN_POINT ( 'NONE',  ( -27.81025873171733664, 19.99999999999999289, 7.666431193274479305 ) ) ;
#2464=ORIENTED_EDGE ( 'NONE', *, *, #13937, .F. ) ;
#2465=CARTESIAN_POINT ( 'NONE',  ( 27.48361012698979522, 126.6227766016837819, 6.072704737864100906E-13 ) ) ;
#2466=CARTESIAN_POINT ( 'NONE',  ( 12.11856678106299512, 143.7750213247282431, 17.70723251555758537 ) ) ;
#2469=ORIENTED_EDGE ( 'NONE', *, *, #10090, .F. ) ;
#2473=ORIENTED_EDGE ( 'NONE', *, *, #2718, .F. ) ;
#2475=CIRCLE ( 'NONE', #12661, 5.000000000000004441 ) ;
#2477=VERTEX_POINT ( 'NONE', #15930 ) ;
#2478=CARTESIAN_POINT ( 'NONE',  ( -27.99999999999998224, 10.00000000000000000, 10.00000000000000178 ) ) ;
#2481=FACE_OUTER_BOUND ( 'NONE', #13023, .T. ) ;
#2485=CARTESIAN_POINT ( 'NONE',  ( 225.0000000000000000, 89.99999999999997158, 15.00000000000000000 ) ) ;
#2488=DIRECTION ( 'NONE',  ( -1.000000000000000000, -0.000000000000000000, -0.000000000000000000 ) ) ;
#2490=DIRECTION ( 'NONE',  ( 0.000000000000000000, -1.000000000000000000, 0.000000000000000000 ) ) ;
#2493=CARTESIAN_POINT ( 'NONE',  ( 48.00000000000000711, 175.6227766016838530, 19.42820660268601074 ) ) ;
#2495=CARTESIAN_POINT ( 'NONE',  ( -27.99999999999998224, 10.00000000000000000, 0.000000000000000000 ) ) ;
#2499=CARTESIAN_POINT ( 'NONE',  ( 13.23724818701972161, 139.1606502921264905, 9.139539437136063427 ) ) ;
#2500=VERTEX_POINT ( 'NONE', #7964 ) ;
#2502=CARTESIAN_POINT ( 'NONE',  ( 14.93242934743711814, 20.00000000000000355, 15.00000000000000000 ) ) ;
#2505=DIRECTION ( 'NONE',  ( 0.000000000000000000, 0.000000000000000000, -1.000000000000000000 ) ) ;
#2506=EDGE_CURVE ( 'NONE', #12384, #4864, #8481, .T. ) ;
#2511=CARTESIAN_POINT ( 'NONE',  ( 28.44374398009894023, 151.3901271056992925, 26.07015880384262729 ) ) ;
#2513=ORIENTED_EDGE ( 'NONE', *, *, #15448, .T. ) ;
#2515=AXIS2_PLACEMENT_3D ( 'NONE', #9598, #4298, #16250 ) ;
#2521=CARTESIAN_POINT ( 'NONE',  ( 196.0000000000000000, 179.6227766016838245, 10.00000337241049309 ) ) ;
#2524=ADVANCED_FACE ( 'NONE', ( #13453 ), #14982, .F. ) ;
#2527=AXIS2_PLACEMENT_3D ( 'NONE', #906, #6294, #11684 ) ;
#2531=CARTESIAN_POINT ( 'NONE',  ( -18.25212770525997286, 32.30769230769230660, 4.999999999999999112 ) ) ;
#2532=EDGE_CURVE ( 'NONE', #12169, #6282, #17262, .T. ) ;
#2533=DIRECTION ( 'NONE',  ( -1.000000000000000000, 0.000000000000000000, 0.000000000000000000 ) ) ;
#2534=CARTESIAN_POINT ( 'NONE',  ( 48.00000000000000711, 183.6227766016837961, 5.571800142134975431 ) ) ;
#2535=CARTESIAN_POINT ( 'NONE',  ( -80.40558230539225804, 151.6102025845144112, 26.23924109008941130 ) ) ;
#2536=EDGE_LOOP ( 'NONE', ( #10221, #42, #10080 ) ) ;
#2538=DIRECTION ( 'NONE',  ( 0.000000000000000000, 0.000000000000000000, 1.000000000000000000 ) ) ;
#2543=PLANE ( 'NONE',  #1576 ) ;
#2547=CARTESIAN_POINT ( 'NONE',  ( 28.84079492301047765, 201.4909985710883689, 14.03234625026787619 ) ) ;
#2548=VERTEX_POINT ( 'NONE', #14438 ) ;
#2549=LINE ( 'NONE', #871, #15753 ) ;
#2553=CARTESIAN_POINT ( 'NONE',  ( -75.02794788578133023, 146.0169975363980370, 20.82225907110315788 ) ) ;
#2555=AXIS2_PLACEMENT_3D ( 'NONE', #4671, #1838, #11481 ) ;
#2559=CARTESIAN_POINT ( 'NONE',  ( -16.40540729975244005, 20.00000000000000000, 23.03124090058168960 ) ) ;
#2565=EDGE_CURVE ( 'NONE', #14379, #1461, #573, .T. ) ;
#2566=EDGE_CURVE ( 'NONE', #6747, #5655, #4534, .T. ) ;
#2570=AXIS2_PLACEMENT_3D ( 'NONE', #6870, #9425, #13248 ) ;
#2576=ORIENTED_EDGE ( 'NONE', *, *, #17330, .F. ) ;
#2577=LINE ( 'NONE', #14514, #5309 ) ;
#2582=DIRECTION ( 'NONE',  ( 0.000000000000000000, -1.000000000000000000, 0.000000000000000000 ) ) ;
#2584=LINE ( 'NONE', #14786, #11225 ) ;
#2586=CARTESIAN_POINT ( 'NONE',  ( 196.0000000000000000, 171.6227766016838245, 12.50000337241049131 ) ) ;
#2591=ORIENTED_EDGE ( 'NONE', *, *, #78, .F. ) ;
#2592=DIRECTION ( 'NONE',  ( 0.000000000000000000, 1.000000000000000000, 0.000000000000000000 ) ) ;
#2593=DIRECTION ( 'NONE',  ( 1.000000000000000000, 0.000000000000000000, -0.000000000000000000 ) ) ;
#2595=CARTESIAN_POINT ( 'NONE',  ( -11.99122994684825549, 19.99999999999999645, 24.50500383881168176 ) ) ;
#2596=CARTESIAN_POINT ( 'NONE',  ( 23.14977753070779087, 141.0007991078602743, 12.30735618844933832 ) ) ;
#2597=AXIS2_PLACEMENT_3D ( 'NONE', #16693, #14032, #1898 ) ;
#2598=ORIENTED_EDGE ( 'NONE', *, *, #9370, .F. ) ;
#2601=CARTESIAN_POINT ( 'NONE',  ( 15.00000000000000000, 154.3022685259950038, 9.999999999999900524 ) ) ;
#2605=ADVANCED_FACE ( 'NONE', ( #9197 ), #10613, .F. ) ;
#2606=VERTEX_POINT ( 'NONE', #4000 ) ;
#2607=CARTESIAN_POINT ( 'NONE',  ( 25.75259266847351469, 149.2783667126899445, 24.28707720053400720 ) ) ;
#2610=DIRECTION ( 'NONE',  ( -0.000000000000000000, -0.000000000000000000, -1.000000000000000000 ) ) ;
#2613=ORIENTED_EDGE ( 'NONE', *, *, #10834, .T. ) ;
#2615=FACE_OUTER_BOUND ( 'NONE', #17467, .T. ) ;
#2616=VERTEX_POINT ( 'NONE', #5044 ) ;
#2621=CARTESIAN_POINT ( 'NONE',  ( -83.66276280984922664, 150.0417915422717385, 24.96744664354709897 ) ) ;
#2622=EDGE_CURVE ( 'NONE', #5481, #16728, #12437, .T. ) ;
#2628=CYLINDRICAL_SURFACE ( 'NONE', #16666, 20.00000000000000355 ) ;
#2637=VERTEX_POINT ( 'NONE', #5483 ) ;
#2643=DIRECTION ( 'NONE',  ( 0.000000000000000000, 0.000000000000000000, 1.000000000000000000 ) ) ;
#2644=CARTESIAN_POINT ( 'NONE',  ( -23.00000000000000000, 120.0000000000000426, 15.00000000000000000 ) ) ;
#2645=DIRECTION ( 'NONE',  ( 0.000000000000000000, 0.000000000000000000, -1.000000000000000000 ) ) ;
#2646=LINE ( 'NONE', #14593, #6086 ) ;
#2653=CARTESIAN_POINT ( 'NONE',  ( -3.000000000000000888, 171.6227766016838245, 0.000000000000000000 ) ) ;
#2664=CIRCLE ( 'NONE', #10279, 2.500000000000002220 ) ;
#2665=VERTEX_POINT ( 'NONE', #16469 ) ;
#2669=LINE ( 'NONE', #1249, #1321 ) ;
#2670=EDGE_LOOP ( 'NONE', ( #5847, #14722, #17390, #10744, #8749 ) ) ;
#2672=CARTESIAN_POINT ( 'NONE',  ( 15.54198151645489645, 125.3641151175237667, 5.547502007357641318 ) ) ;
#2675=AXIS2_PLACEMENT_3D ( 'NONE', #8938, #9298, #10533 ) ;
#2679=VECTOR ( 'NONE', #4455, 1000.000000000000000 ) ;
#2687=CARTESIAN_POINT ( 'NONE',  ( 33.41665845754520348, 150.2902214191208259, 25.17945278758671890 ) ) ;
#2691=VECTOR ( 'NONE', #11767, 1000.000000000000000 ) ;
#2692=ORIENTED_EDGE ( 'NONE', *, *, #3359, .F. ) ;
#2693=CIRCLE ( 'NONE', #1551, 33.00000000000000000 ) ;
#2697=CARTESIAN_POINT ( 'NONE',  ( -30.49999999999998224, 10.00000000000000000, 10.00000000000000178 ) ) ;
#2698=ORIENTED_EDGE ( 'NONE', *, *, #10082, .T. ) ;
#2701=DIRECTION ( 'NONE',  ( 0.000000000000000000, -1.000000000000000000, 0.000000000000000000 ) ) ;
#2702=CIRCLE ( 'NONE', #4118, 27.69059892324149530 ) ;
#2705=CARTESIAN_POINT ( 'NONE',  ( -100.0000000000000000, 171.6227766016838245, 0.000000000000000000 ) ) ;
#2706=COLOUR_RGB ( '', 0.09019608, 0.27058824, 0.51372549) ;
#2708=EDGE_LOOP ( 'NONE', ( #3084, #10998, #13647, #592, #17481 ) ) ;
#2711=CARTESIAN_POINT ( 'NONE',  ( 21.38845554303141938, 18.00000000000000000, 23.94082098111162082 ) ) ;
#2712=FACE_OUTER_BOUND ( 'NONE', #6902, .T. ) ;
#2713=CARTESIAN_POINT ( 'NONE',  ( -48.00000000000000000, 171.6227766016838245, 0.000000000000000000 ) ) ;
#2714=CIRCLE ( 'NONE', #8655, 2.500000000000002220 ) ;
#2718=EDGE_CURVE ( 'NONE', #12692, #5700, #12173, .T. ) ;
#2719=LINE ( 'NONE', #1482, #12080 ) ;
#2722=LINE ( 'NONE', #3240, #17258 ) ;
#2725=CARTESIAN_POINT ( 'NONE',  ( -20.85266279178580362, 19.99999999999999645, 20.15433268689462665 ) ) ;
#2733=CYLINDRICAL_SURFACE ( 'NONE', #3415, 5.000000000000004441 ) ;
#2734=( LENGTH_UNIT ( ) NAMED_UNIT ( * ) SI_UNIT ( .MILLI., .METRE. ) );
#2738=AXIS2_PLACEMENT_3D ( 'NONE', #8314, #7091, #15047 ) ;
#2740=VECTOR ( 'NONE', #16391, 1000.000000000000000 ) ;
#2742=( NAMED_UNIT ( * ) SI_UNIT ( $, .STERADIAN. ) SOLID_ANGLE_UNIT ( ) );
#2762=EDGE_CURVE ( 'NONE', #11801, #11737, #11321, .T. ) ;
#2764=CARTESIAN_POINT ( 'NONE',  ( -14.90344812367316685, 20.00000000000343547, 8.058388986520416353 ) ) ;
#2765=LINE ( 'NONE', #5591, #10463 ) ;
#2766=ORIENTED_EDGE ( 'NONE', *, *, #16955, .F. ) ;
#2769=DIRECTION ( 'NONE',  ( -1.000000000000000000, 0.000000000000000000, 0.000000000000000000 ) ) ;
#2771=DIRECTION ( 'NONE',  ( 0.000000000000000000, 1.000000000000000000, 0.000000000000000000 ) ) ;
#2775=CARTESIAN_POINT ( 'NONE',  ( 25.30103246056163968, 148.3373224442694891, 23.38426449892925163 ) ) ;
#2776=ORIENTED_EDGE ( 'NONE', *, *, #9372, .F. ) ;
#2780=CARTESIAN_POINT ( 'NONE',  ( 48.00000000000000711, 167.6227766016838530, 5.571800142134975431 ) ) ;
#2781=EDGE_CURVE ( 'NONE', #7251, #3946, #15477, .T. ) ;
#2783=ORIENTED_EDGE ( 'NONE', *, *, #14471, .F. ) ;
#2786=CIRCLE ( 'NONE', #3355, 10.00000000000000000 ) ;
#2787=STYLED_ITEM ( 'NONE', ( #5571 ), #5730 ) ;
#2788=CARTESIAN_POINT ( 'NONE',  ( 8.956670050029527985, 133.3372912347335841, 14.64653510947197645 ) ) ;
#2792=FACE_OUTER_BOUND ( 'NONE', #17024, .T. ) ;
#2793=PLANE ( 'NONE',  #16096 ) ;
#2795=FACE_BOUND ( 'NONE', #4897, .T. ) ;
#2801=CARTESIAN_POINT ( 'NONE',  ( -3.000000000000000888, 171.6227766016838245, 0.000000000000000000 ) ) ;
#2804=EDGE_CURVE ( 'NONE', #15613, #5268, #4856, .T. ) ;
#2806=AXIS2_PLACEMENT_3D ( 'NONE', #7466, #12875, #16519 ) ;
#2815=PLANE ( 'NONE',  #504 ) ;
#2818=AXIS2_PLACEMENT_3D ( 'NONE', #4014, #14796, #10630 ) ;
#2819=CARTESIAN_POINT ( 'NONE',  ( -27.99999999999998224, 10.00000000000000000, 35.00200000000000244 ) ) ;
#2821=AXIS2_PLACEMENT_3D ( 'NONE', #8907, #17143, #9086 ) ;
#2825=CARTESIAN_POINT ( 'NONE',  ( -50.00000000000000000, 171.6227766016838245, 0.000000000000000000 ) ) ;
#2827=ORIENTED_EDGE ( 'NONE', *, *, #1859, .T. ) ;
#2830=DIRECTION ( 'NONE',  ( 0.000000000000000000, 0.000000000000000000, 1.000000000000000000 ) ) ;
#2831=CARTESIAN_POINT ( 'NONE',  ( -3.000000000000000888, 171.6227766016838245, 20.00000000000000355 ) ) ;
#2832=CARTESIAN_POINT ( 'NONE',  ( 0.000000000000000000, 0.000000000000000000, 0.000000000000000000 ) ) ;
#2836=EDGE_CURVE ( 'NONE', #11548, #9285, #15263, .T. ) ;
#2840=EDGE_LOOP ( 'NONE', ( #6962, #7913, #16156, #16780 ) ) ;
#2841=DIRECTION ( 'NONE',  ( -1.156482317317868274E-16, 1.000000000000000000, 0.000000000000000000 ) ) ;
#2842=AXIS2_PLACEMENT_3D ( 'NONE', #9417, #13506, #13766 ) ;
#2843=EDGE_CURVE ( 'NONE', #17386, #17370, #15829, .T. ) ;
#2845=ORIENTED_EDGE ( 'NONE', *, *, #12069, .T. ) ;
#2847=CARTESIAN_POINT ( 'NONE',  ( -14.56452549316047040, 19.99999999999883826, 9.027778560947799846 ) ) ;
#2850=ORIENTED_EDGE ( 'NONE', *, *, #9138, .T. ) ;
#2852=CIRCLE ( 'NONE', #3131, 8.000000000000000000 ) ;
#2853=EDGE_LOOP ( 'NONE', ( #12287, #8763, #9631, #8160 ) ) ;
#2860=CARTESIAN_POINT ( 'NONE',  ( 30.37952724349399958, 151.6237922324447709, 26.24958334688938422 ) ) ;
#2862=DIRECTION ( 'NONE',  ( -1.000000000000000000, 0.000000000000000000, 0.000000000000000000 ) ) ;
#2869=DIRECTION ( 'NONE',  ( 1.000000000000000000, 0.000000000000000000, 0.000000000000000000 ) ) ;
#2870=ORIENTED_EDGE ( 'NONE', *, *, #11598, .T. ) ;
#2875=EDGE_CURVE ( 'NONE', #15013, #15924, #15730, .T. ) ;
#2881=CARTESIAN_POINT ( 'NONE',  ( -725.0000000000001137, 129.9999999999995453, 4.999999999999999112 ) ) ;
#2890=DIRECTION ( 'NONE',  ( 1.000000000000000000, -0.000000000000000000, -0.000000000000000000 ) ) ;
#2891=EDGE_LOOP ( 'NONE', ( #3034, #15944 ) ) ;
#2892=CARTESIAN_POINT ( 'NONE',  ( -95.00000000000000000, 143.9321776784423150, -5.086680500673126297E-15 ) ) ;
#2896=EDGE_CURVE ( 'NONE', #9911, #12513, #15559, .T. ) ;
#2897=EDGE_CURVE ( 'NONE', #5896, #15148, #11320, .T. ) ;
#2900=DIRECTION ( 'NONE',  ( -0.000000000000000000, -0.000000000000000000, -1.000000000000000000 ) ) ;
#2907=FACE_BOUND ( 'NONE', #16814, .T. ) ;
#2910=( NAMED_UNIT ( * ) PLANE_ANGLE_UNIT ( ) SI_UNIT ( $, .RADIAN. ) );
#2914=CARTESIAN_POINT ( 'NONE',  ( 30.40149590727984830, 191.6349927435749407, 26.23951396249186274 ) ) ;
#2920=ORIENTED_EDGE ( 'NONE', *, *, #16954, .F. ) ;
#2924=DIRECTION ( 'NONE',  ( 1.000000000000000000, 0.000000000000000000, 0.000000000000000000 ) ) ;
#2925=ORIENTED_EDGE ( 'NONE', *, *, #3825, .F. ) ;
#2926=CARTESIAN_POINT ( 'NONE',  ( -22.80699178664306004, 19.99999999999999645, 18.33022619056923119 ) ) ;
#2930=EDGE_CURVE ( 'NONE', #10705, #8790, #10941, .T. ) ;
#2932=DIRECTION ( 'NONE',  ( 0.000000000000000000, 0.000000000000000000, 1.000000000000000000 ) ) ;
#2934=DIRECTION ( 'NONE',  ( 1.000000000000000000, 1.156482317317868274E-16, -0.000000000000000000 ) ) ;
#2937=EDGE_CURVE ( 'NONE', #7044, #14845, #10755, .T. ) ;
#2938=EDGE_CURVE ( 'NONE', #10721, #4086, #9697, .T. ) ;
#2939=DIRECTION ( 'NONE',  ( 1.000000000000000000, 0.000000000000000000, 0.000000000000000000 ) ) ;
#2941=FACE_BOUND ( 'NONE', #12143, .T. ) ;
#2943=CARTESIAN_POINT ( 'NONE',  ( -80.00000000000002842, 146.6227766016838245, 10.00000000000000178 ) ) ;
#2945=CARTESIAN_POINT ( 'NONE',  ( -80.00000000000002842, 146.6227766016838245, 0.000000000000000000 ) ) ;
#2946=ORIENTED_EDGE ( 'NONE', *, *, #7071, .T. ) ;
#2947=ORIENTED_EDGE ( 'NONE', *, *, #16713, .T. ) ;
#2950=DIRECTION ( 'NONE',  ( -1.000000000000000000, -0.000000000000000000, -0.000000000000000000 ) ) ;
#2951=CARTESIAN_POINT ( 'NONE',  ( 10.98422133653362920, 132.2143956889292724, 13.95899527751216240 ) ) ;
#2954=CARTESIAN_POINT ( 'NONE',  ( -34.99999999999999289, 120.0000000000000284, 4.999999999999999112 ) ) ;
#2955=LINE ( 'NONE', #8091, #11169 ) ;
#2957=DIRECTION ( 'NONE',  ( 1.000000000000000000, 0.000000000000000000, 0.000000000000000000 ) ) ;
#2960=CIRCLE ( 'NONE', #7194, 2.500000000000000444 ) ;
#2962=CARTESIAN_POINT ( 'NONE',  ( 40.00000000000000711, 206.6227766016838245, 0.000000000000000000 ) ) ;
#2964=DIRECTION ( 'NONE',  ( -1.000000000000000000, 0.000000000000000000, 0.000000000000000000 ) ) ;
#2968=ORIENTED_EDGE ( 'NONE', *, *, #5699, .F. ) ;
#2970=EDGE_CURVE ( 'NONE', #4551, #3929, #1563, .T. ) ;
#2975=CARTESIAN_POINT ( 'NONE',  ( -15.00000000000002487, 120.0000000000000284, 4.999999999999999112 ) ) ;
#2977=VECTOR ( 'NONE', #12756, 1000.000000000000000 ) ;
#2983=CARTESIAN_POINT ( 'NONE',  ( 30.00000000000001066, 146.6227766016838245, 0.000000000000000000 ) ) ;
#2987=CIRCLE ( 'NONE', #15139, 2.500000000000002220 ) ;
#2989=EDGE_CURVE ( 'NONE', #1199, #13489, #66, .T. ) ;
#2990=EDGE_CURVE ( 'NONE', #11907, #13275, #11597, .T. ) ;
#2992=ORIENTED_EDGE ( 'NONE', *, *, #5206, .F. ) ;
#2993=FACE_BOUND ( 'NONE', #10684, .T. ) ;
#2995=ORIENTED_EDGE ( 'NONE', *, *, #1705, .T. ) ;
#2996=( LENGTH_UNIT ( ) NAMED_UNIT ( * ) SI_UNIT ( .MILLI., .METRE. ) );
#2999=DIRECTION ( 'NONE',  ( -1.000000000000000000, -0.000000000000000000, -0.000000000000000000 ) ) ;
#3002=LINE ( 'NONE', #8400, #961 ) ;
#3003=CARTESIAN_POINT ( 'NONE',  ( 48.00000000000000711, 175.6227766016838530, 16.92820660268601429 ) ) ;
#3004=CARTESIAN_POINT ( 'NONE',  ( -95.00000000000000000, 199.3133755249253056, 1.695560166891042033E-15 ) ) ;
#3009=DIRECTION ( 'NONE',  ( -0.000000000000000000, -0.000000000000000000, -1.000000000000000000 ) ) ;
#3010=CIRCLE ( 'NONE', #10354, 2.499999999999998668 ) ;
#3013=EDGE_LOOP ( 'NONE', ( #12312, #16569, #9690, #2870 ) ) ;
#3016=CARTESIAN_POINT ( 'NONE',  ( -80.00000000000002842, 146.6227766016838245, 0.000000000000000000 ) ) ;
#3022=CARTESIAN_POINT ( 'NONE',  ( -24.94987437106621542, 20.00000000000004263, 5.999999999999992895 ) ) ;
#3024=DIRECTION ( 'NONE',  ( 0.000000000000000000, 0.000000000000000000, -1.000000000000000000 ) ) ;
#3027=ORIENTED_EDGE ( 'NONE', *, *, #11645, .T. ) ;
#3033=CYLINDRICAL_SURFACE ( 'NONE', #7235, 33.00000000000000000 ) ;
#3034=ORIENTED_EDGE ( 'NONE', *, *, #7584, .F. ) ;
#3040=CARTESIAN_POINT ( 'NONE',  ( 17.54349574104657705, 125.4948194589026684, 5.000000000000002665 ) ) ;
#3041=ORIENTED_EDGE ( 'NONE', *, *, #9973, .F. ) ;
#3042=DIRECTION ( 'NONE',  ( 0.000000000000000000, 0.000000000000000000, -1.000000000000000000 ) ) ;
#3046=CARTESIAN_POINT ( 'NONE',  ( 16.23725950538872809, 18.00000000000000000, 24.99999999982344789 ) ) ;
#3047=CARTESIAN_POINT ( 'NONE',  ( -27.70723240392776532, 19.99999999999999289, 8.328409877367407788 ) ) ;
#3049=CARTESIAN_POINT ( 'NONE',  ( 30.00000000000000355, 196.6227766016838245, 11.50215154306610188 ) ) ;
#3050=VECTOR ( 'NONE', #663, 1000.000000000000000 ) ;
#3051=CARTESIAN_POINT ( 'NONE',  ( 48.00000000000000711, 179.6227766016838245, 15.00000337241049486 ) ) ;
#3054=DIRECTION ( 'NONE',  ( -0.000000000000000000, -0.000000000000000000, -1.000000000000000000 ) ) ;
#3055=AXIS2_PLACEMENT_3D ( 'NONE', #7290, #653, #3634 ) ;
#3057=ORIENTED_EDGE ( 'NONE', *, *, #10246, .F. ) ;
#3061=VERTEX_POINT ( 'NONE', #14840 ) ;
#3062=EDGE_CURVE ( 'NONE', #8265, #8813, #2722, .T. ) ;
#3067=CIRCLE ( 'NONE', #15787, 2.500000000000000000 ) ;
#3070=DIRECTION ( 'NONE',  ( 1.000000000000000000, -0.000000000000000000, -0.000000000000000000 ) ) ;
#3073=FACE_OUTER_BOUND ( 'NONE', #8687, .T. ) ;
#3075=ORIENTED_EDGE ( 'NONE', *, *, #16199, .F. ) ;
#3076=CARTESIAN_POINT ( 'NONE',  ( 34.78753451919190098, 145.1525832006840631, 19.71138291685209154 ) ) ;
#3077=FACE_OUTER_BOUND ( 'NONE', #3670, .T. ) ;
#3078=EDGE_CURVE ( 'NONE', #6948, #14253, #5806, .T. ) ;
#3079=FACE_BOUND ( 'NONE', #524, .T. ) ;
#3080=DIRECTION ( 'NONE',  ( 1.000000000000000000, 0.000000000000000000, -0.000000000000000000 ) ) ;
#3084=ORIENTED_EDGE ( 'NONE', *, *, #15675, .F. ) ;
#3086=EDGE_LOOP ( 'NONE', ( #13012, #5925 ) ) ;
#3090=AXIS2_PLACEMENT_3D ( 'NONE', #16541, #15024, #16633 ) ;
#3092=CARTESIAN_POINT ( 'NONE',  ( 30.79456682210174634, 191.6823464236538541, 26.20333082749370135 ) ) ;
#3097=ADVANCED_FACE ( 'NONE', ( #16878 ), #7403, .F. ) ;
#3100=EDGE_CURVE ( 'NONE', #2211, #5446, #15287, .T. ) ;
#3106=ORIENTED_EDGE ( 'NONE', *, *, #4473, .F. ) ;
#3107=CARTESIAN_POINT ( 'NONE',  ( -13.51825462539708056, 19.99999999999884892, 10.94502331224290259 ) ) ;
#3109=CYLINDRICAL_SURFACE ( 'NONE', #12742, 2.500000000000000444 ) ;
#3114=FACE_OUTER_BOUND ( 'NONE', #11893, .T. ) ;
#3116=AXIS2_PLACEMENT_3D ( 'NONE', #8384, #7067, #7149 ) ;
#3117=FACE_OUTER_BOUND ( 'NONE', #9378, .T. ) ;
#3120=AXIS2_PLACEMENT_3D ( 'NONE', #16364, #4317, #4403 ) ;
#3124=FACE_BOUND ( 'NONE', #13387, .T. ) ;
#3125=EDGE_LOOP ( 'NONE', ( #5478, #12634, #10559, #14036 ) ) ;
#3126=DIRECTION ( 'NONE',  ( -0.000000000000000000, -1.000000000000000000, 2.312964634635742267E-15 ) ) ;
#3130=CARTESIAN_POINT ( 'NONE',  ( -80.00000000000001421, 196.6227766016838245, 35.00200000000000244 ) ) ;
#3131=AXIS2_PLACEMENT_3D ( 'NONE', #6029, #10323, #8270 ) ;
#3133=CARTESIAN_POINT ( 'NONE',  ( 16.78995144247101123, 126.8031893778130410, 8.318227863269529010 ) ) ;
#3134=VECTOR ( 'NONE', #1541, 1000.000000000000000 ) ;
#3138=ADVANCED_FACE ( 'NONE', ( #12806 ), #11299, .T. ) ;
#3140=CARTESIAN_POINT ( 'NONE',  ( -85.00000000000001421, 196.1091490972146119, 22.13677318565945740 ) ) ;
#3143=CARTESIAN_POINT ( 'NONE',  ( 16.75727253400481942, 18.00000000000057199, 12.82782196133976704 ) ) ;
#3155=CARTESIAN_POINT ( 'NONE',  ( 15.42236477930291549, 143.2198172345435410, 16.80652640733168823 ) ) ;
#3162=EDGE_CURVE ( 'NONE', #254, #2477, #11202, .T. ) ;
#3164=DIRECTION ( 'NONE',  ( 1.000000000000000000, 0.000000000000000000, 0.000000000000000000 ) ) ;
#3167=CARTESIAN_POINT ( 'NONE',  ( 32.06308580867288072, 142.0644190903623496, 14.67410160148081211 ) ) ;
#3170=FACE_BOUND ( 'NONE', #10254, .T. ) ;
#3176=ORIENTED_EDGE ( 'NONE', *, *, #4744, .F. ) ;
#3181=CARTESIAN_POINT ( 'NONE',  ( 27.48361012698968864, 138.6227766016838245, 1.063447695028166570E-14 ) ) ;
#3182=CARTESIAN_POINT ( 'NONE',  ( 25.35096429952119834, 194.7608640721562949, 23.53240337055841991 ) ) ;
#3183=DIRECTION ( 'NONE',  ( -1.000000000000000000, -0.000000000000000000, -0.000000000000000000 ) ) ;
#3184=CARTESIAN_POINT ( 'NONE',  ( -70.00000000000000000, 171.6227766016838245, 0.000000000000000000 ) ) ;
#3185=CARTESIAN_POINT ( 'NONE',  ( 18.47699279854304777, 29.92902263789611439, 12.17729482734268132 ) ) ;
#3192=ORIENTED_EDGE ( 'NONE', *, *, #13843, .T. ) ;
#3200=CARTESIAN_POINT ( 'NONE',  ( -68.00000000000000000, 206.6227766016838245, -2.143131898507868248E-15 ) ) ;
#3201=CARTESIAN_POINT ( 'NONE',  ( -27.98221281347037959, 20.00000000000000000, -15.00000000000000000 ) ) ;
#3205=EDGE_LOOP ( 'NONE', ( #12031, #3572 ) ) ;
#3206=CARTESIAN_POINT ( 'NONE',  ( -40.00000000000000000, 20.00000000000000000, 30.00000000000000355 ) ) ;
#3208=CARTESIAN_POINT ( 'NONE',  ( 196.0000000000000000, 155.6227766016839098, 12.50000337241049309 ) ) ;
#3211=DIRECTION ( 'NONE',  ( 0.000000000000000000, 1.000000000000000000, 0.000000000000000000 ) ) ;
#3214=DIRECTION ( 'NONE',  ( 0.000000000000000000, 0.000000000000000000, 1.000000000000000000 ) ) ;
#3215=EDGE_CURVE ( 'NONE', #15544, #5268, #7727, .T. ) ;
#3216=CARTESIAN_POINT ( 'NONE',  ( 27.25143353317894324, 137.1251711682953385, 6.002437647192902404 ) ) ;
#3223=CARTESIAN_POINT ( 'NONE',  ( 17.58250999373989742, 125.2198453306090045, 1.666666666666656749 ) ) ;
#3226=CARTESIAN_POINT ( 'NONE',  ( 30.00000000000001066, 146.6227766016838245, 11.50215154306610188 ) ) ;
#3228=ORIENTED_EDGE ( 'NONE', *, *, #5445, .F. ) ;
#3229=DIRECTION ( 'NONE',  ( 0.000000000000000000, 0.000000000000000000, 1.000000000000000000 ) ) ;
#3234=VERTEX_POINT ( 'NONE', #11715 ) ;
#3236=CARTESIAN_POINT ( 'NONE',  ( -95.00000000000000000, 143.9321776784423150, -5.086680500673126297E-15 ) ) ;
#3240=CARTESIAN_POINT ( 'NONE',  ( -85.00000000000002842, 196.6227766016838245, 35.00200000000000244 ) ) ;
#3241=DIRECTION ( 'NONE',  ( 0.000000000000000000, 0.000000000000000000, -1.000000000000000000 ) ) ;
#3242=AXIS2_PLACEMENT_3D ( 'NONE', #3731, #974, #17089 ) ;
#3244=DIRECTION ( 'NONE',  ( 0.000000000000000000, -1.000000000000000000, 6.123233995736762338E-17 ) ) ;
#3245=CONICAL_SURFACE ( 'NONE', #3812, 2.500000000000002220, 1.029744260000002631 ) ;
#3246=ORIENTED_EDGE ( 'NONE', *, *, #16042, .T. ) ;
#3249=FACE_BOUND ( 'NONE', #5156, .T. ) ;
#3253=EDGE_CURVE ( 'NONE', #13316, #254, #4910, .T. ) ;
#3260=CARTESIAN_POINT ( 'NONE',  ( 8.602893093599609742, 142.4623620169580818, 19.35743923737696903 ) ) ;
#3265=AXIS2_PLACEMENT_3D ( 'NONE', #16625, #13965, #3241 ) ;
#3272=ORIENTED_EDGE ( 'NONE', *, *, #2836, .F. ) ;
#3279=PRODUCT_DEFINITION ( 'UNKNOWN', '', #8129, #4310 ) ;
#3281=AXIS2_PLACEMENT_3D ( 'NONE', #1986, #7386, #12784 ) ;
#3286=ADVANCED_FACE ( 'NONE', ( #15802 ), #1437, .F. ) ;
#3287=CARTESIAN_POINT ( 'NONE',  ( -27.98221281347037959, 18.00000000000000355, 4.999999999999999112 ) ) ;
#3289=DIRECTION ( 'NONE',  ( 0.000000000000000000, -0.4999999999999952816, -0.8660254037844413721 ) ) ;
#3297=ADVANCED_FACE ( 'NONE', ( #10486, #9150 ), #14556, .F. ) ;
#3298=VECTOR ( 'NONE', #15934, 1000.000000000000000 ) ;
#3304=CARTESIAN_POINT ( 'NONE',  ( 29.54149365486396661, 20.00000000000000711, 18.67620474358521676 ) ) ;
#3305=CARTESIAN_POINT ( 'NONE',  ( 24.02621431236828187, 19.99999999999771916, 9.488192989094725860 ) ) ;
#3306=CARTESIAN_POINT ( 'NONE',  ( 17.14535223351611748, 126.3036220646326910, 7.355580850454368047 ) ) ;
#3311=FACE_OUTER_BOUND ( 'NONE', #740, .T. ) ;
#3312=VECTOR ( 'NONE', #14242, 1000.000000000000000 ) ;
#3315=AXIS2_PLACEMENT_3D ( 'NONE', #17142, #12270, #5463 ) ;
#3316=CARTESIAN_POINT ( 'NONE',  ( -76.71739856777422517, 192.8472041258103218, 25.26942977006890345 ) ) ;
#3318=CYLINDRICAL_SURFACE ( 'NONE', #1326, 2.500000000000000444 ) ;
#3319=CYLINDRICAL_SURFACE ( 'NONE', #16808, 30.00000000000000000 ) ;
#3323=EDGE_CURVE ( 'NONE', #14499, #7978, #16139, .T. ) ;
#3326=VERTEX_POINT ( 'NONE', #6687 ) ;
#3330=EDGE_LOOP ( 'NONE', ( #16952, #4145, #14134, #8499, #1403 ) ) ;
#3333=AXIS2_PLACEMENT_3D ( 'NONE', #11530, #6552, #10706 ) ;
#3334=CARTESIAN_POINT ( 'NONE',  ( 10.03770976535549586, 140.0890479961802839, 11.85997561143382661 ) ) ;
#3336=CARTESIAN_POINT ( 'NONE',  ( 48.00000000000000711, 175.6227766016838245, 3.071800142134975431 ) ) ;
#3337=ORIENTED_EDGE ( 'NONE', *, *, #3864, .T. ) ;
#3341=LINE ( 'NONE', #5814, #722 ) ;
#3343=AXIS2_PLACEMENT_3D ( 'NONE', #9331, #16164, #16432 ) ;
#3344=ORIENTED_EDGE ( 'NONE', *, *, #1052, .T. ) ;
#3345=DIRECTION ( 'NONE',  ( -1.000000000000000000, -0.000000000000000000, -0.000000000000000000 ) ) ;
#3347=EDGE_CURVE ( 'NONE', #9730, #4275, #12746, .T. ) ;
#3351=CARTESIAN_POINT ( 'NONE',  ( -3.000000000000000888, 206.6227766016838245, -2.143131898507868248E-15 ) ) ;
#3352=VECTOR ( 'NONE', #10929, 1000.000000000000000 ) ;
#3353=ORIENTED_EDGE ( 'NONE', *, *, #10094, .F. ) ;
#3355=AXIS2_PLACEMENT_3D ( 'NONE', #167, #5574, #4426 ) ;
#3359=EDGE_CURVE ( 'NONE', #13584, #5251, #5104, .T. ) ;
#3360=CARTESIAN_POINT ( 'NONE',  ( -70.00000000000000000, 171.6227766016838245, 20.00000000000000355 ) ) ;
#3361=ORIENTED_EDGE ( 'NONE', *, *, #13937, .T. ) ;
#3362=LINE ( 'NONE', #12825, #3312 ) ;
#3363=DIRECTION ( 'NONE',  ( -0.000000000000000000, -0.000000000000000000, -1.000000000000000000 ) ) ;
#3364=VECTOR ( 'NONE', #12098, 1000.000000000000000 ) ;
#3368=VERTEX_POINT ( 'NONE', #1466 ) ;
#3373=CIRCLE ( 'NONE', #12402, 30.00000000000000000 ) ;
#3378=DIRECTION ( 'NONE',  ( -1.000000000000000000, -0.000000000000000000, -0.000000000000000000 ) ) ;
#3382=CARTESIAN_POINT ( 'NONE',  ( -19.26597175465492739, 18.00000000000000000, 21.35691006828201566 ) ) ;
#3385=VERTEX_POINT ( 'NONE', #9676 ) ;
#3391=EDGE_CURVE ( 'NONE', #15051, #13756, #14704, .T. ) ;
#3392=CARTESIAN_POINT ( 'NONE',  ( 39.99999999999998579, 20.00000000000000000, 30.00000000000001066 ) ) ;
#3393=CIRCLE ( 'NONE', #9880, 2.500000000000002220 ) ;
#3395=LINE ( 'NONE', #4550, #7517 ) ;
#3399=CARTESIAN_POINT ( 'NONE',  ( 14.92319712166297840, 137.6313713749984800, 10.11910373048645440 ) ) ;
#3405=CARTESIAN_POINT ( 'NONE',  ( -75.16864359540511487, 195.3043783022527862, 22.98536326679098707 ) ) ;
#3412=ORIENTED_EDGE ( 'NONE', *, *, #7648, .T. ) ;
#3413=CARTESIAN_POINT ( 'NONE',  ( 48.00000000000000711, 155.6227766016839098, 12.50000337241049309 ) ) ;
#3415=AXIS2_PLACEMENT_3D ( 'NONE', #2819, #10786, #9276 ) ;
#3421=VERTEX_POINT ( 'NONE', #14912 ) ;
#3427=CIRCLE ( 'NONE', #13321, 20.00000000000000355 ) ;
#3430=CARTESIAN_POINT ( 'NONE',  ( 27.50000000000000355, 196.6227766016838245, 10.00000000000000178 ) ) ;
#3432=DIRECTION ( 'NONE',  ( -1.000000000000000000, -0.000000000000000000, -0.000000000000000000 ) ) ;
#3439=ORIENTED_EDGE ( 'NONE', *, *, #3790, .T. ) ;
#3445=EDGE_CURVE ( 'NONE', #1301, #9322, #13675, .T. ) ;
#3449=PLANE ( 'NONE',  #15184 ) ;
#3450=FACE_OUTER_BOUND ( 'NONE', #8697, .T. ) ;
#3453=ORIENTED_EDGE ( 'NONE', *, *, #12739, .T. ) ;
#3459=FACE_OUTER_BOUND ( 'NONE', #12755, .T. ) ;
#3460=DIRECTION ( 'NONE',  ( -1.000000000000000000, 0.000000000000000000, 0.000000000000000000 ) ) ;
#3461=ORIENTED_EDGE ( 'NONE', *, *, #15421, .T. ) ;
#3466=CARTESIAN_POINT ( 'NONE',  ( -16.24840885328083928, 32.75254598042347709, 6.058899415740283345 ) ) ;
#3469=ORIENTED_EDGE ( 'NONE', *, *, #15762, .T. ) ;
#3471=ORIENTED_EDGE ( 'NONE', *, *, #11776, .T. ) ;
#3478=EDGE_CURVE ( 'NONE', #3840, #8790, #11607, .T. ) ;
#3479=CARTESIAN_POINT ( 'NONE',  ( 24.93034343272635667, 19.99999999999999645, 22.33460256652156062 ) ) ;
#3481=EDGE_CURVE ( 'NONE', #2477, #9250, #7696, .T. ) ;
#3482=DIRECTION ( 'NONE',  ( 0.000000000000000000, 0.000000000000000000, 1.000000000000000000 ) ) ;
#3484=CARTESIAN_POINT ( 'NONE',  ( -76.23821662194384885, 193.3250171236886104, 24.86042266551077873 ) ) ;
#3487=DIRECTION ( 'NONE',  ( -1.000000000000000000, -0.000000000000000000, -0.000000000000000000 ) ) ;
#3488=ORIENTED_EDGE ( 'NONE', *, *, #13115, .F. ) ;
#3490=DIRECTION ( 'NONE',  ( 1.000000000000000000, 0.000000000000000000, 0.000000000000000000 ) ) ;
#3494=ORIENTED_EDGE ( 'NONE', *, *, #12359, .F. ) ;
#3499=EDGE_LOOP ( 'NONE', ( #17074, #5080, #669, #10368, #13006 ) ) ;
#3502=CARTESIAN_POINT ( 'NONE',  ( 14.79728876016037198, 126.7368160533725643, 7.941237055946955614 ) ) ;
#3505=CARTESIAN_POINT ( 'NONE',  ( 20.85766706164172035, 17.99999999999999645, 10.55326734450395954 ) ) ;
#3506=CARTESIAN_POINT ( 'NONE',  ( -100.0000000000000000, 141.6227766016838245, 0.000000000000000000 ) ) ;
#3508=ORIENTED_EDGE ( 'NONE', *, *, #3478, .T. ) ;
#3512=CARTESIAN_POINT ( 'NONE',  ( 23.92262868871285519, 29.88142130320016676, 9.432657661123421633 ) ) ;
#3514=EDGE_CURVE ( 'NONE', #11646, #8664, #8503, .T. ) ;
#3515=CARTESIAN_POINT ( 'NONE',  ( 32.22224914908579763, 201.1051302811612516, 14.82644580554060987 ) ) ;
#3516=ORIENTED_EDGE ( 'NONE', *, *, #3445, .T. ) ;
#3517=DIRECTION ( 'NONE',  ( 0.000000000000000000, 0.000000000000000000, -1.000000000000000000 ) ) ;
#3519=VECTOR ( 'NONE', #11349, 1000.000000000000000 ) ;
#3521=CARTESIAN_POINT ( 'NONE',  ( 196.0000000000000000, 155.6227766016839098, 10.00000337241049309 ) ) ;
#3524=CARTESIAN_POINT ( 'NONE',  ( 48.00000000000000711, 175.6227766016838530, 19.42820660268601074 ) ) ;
#3525=ORIENTED_EDGE ( 'NONE', *, *, #9081, .T. ) ;
#3526=LINE ( 'NONE', #3785, #12093 ) ;
#3528=CARTESIAN_POINT ( 'NONE',  ( 48.00000000000000711, 179.6227766016838245, 12.50000337241049309 ) ) ;
#3531=EDGE_LOOP ( 'NONE', ( #16082, #13773 ) ) ;
#3538=EDGE_CURVE ( 'NONE', #9695, #17286, #12519, .T. ) ;
#3540=CARTESIAN_POINT ( 'NONE',  ( -75.00000000000000000, 196.6227766016838245, 21.54065922853802206 ) ) ;
#3541=ORIENTED_EDGE ( 'NONE', *, *, #11525, .T. ) ;
#3542=CYLINDRICAL_SURFACE ( 'NONE', #11779, 2.500000000000000444 ) ;
#3543=DIRECTION ( 'NONE',  ( 1.000000000000000000, 0.000000000000000000, 8.673617379884037937E-17 ) ) ;
#3550=CARTESIAN_POINT ( 'NONE',  ( -10.22933296213221865, 30.92590585860461161, 12.59260918105267457 ) ) ;
#3551=CARTESIAN_POINT ( 'NONE',  ( -15.00000000000001421, 130.0000000000000000, 13.00000000000000000 ) ) ;
#3553=ORIENTED_EDGE ( 'NONE', *, *, #14370, .T. ) ;
#3554=DIRECTION ( 'NONE',  ( -0.000000000000000000, -0.000000000000000000, -1.000000000000000000 ) ) ;
#3558=AXIS2_PLACEMENT_3D ( 'NONE', #17490, #9597, #16342 ) ;
#3563=CARTESIAN_POINT ( 'NONE',  ( 34.80444759362561058, 19.99999999999999645, 7.621511755370173447 ) ) ;
#3569=AXIS2_PLACEMENT_3D ( 'NONE', #11001, #13667, #12332 ) ;
#3571=EDGE_CURVE ( 'NONE', #4864, #12384, #6166, .T. ) ;
#3572=ORIENTED_EDGE ( 'NONE', *, *, #11370, .F. ) ;
#3573=CARTESIAN_POINT ( 'NONE',  ( 48.00000000000000000, 171.6227766016838245, 12.50000337241049131 ) ) ;
#3577=CARTESIAN_POINT ( 'NONE',  ( -22.93725393319379435, 100.0000000000000142, 6.000000000000000000 ) ) ;
#3578=ORIENTED_EDGE ( 'NONE', *, *, #17229, .T. ) ;
#3581=VECTOR ( 'NONE', #11685, 1000.000000000000000 ) ;
#3583=AXIS2_PLACEMENT_3D ( 'NONE', #5482, #6893, #8222 ) ;
#3588=CARTESIAN_POINT ( 'NONE',  ( -11.09520285051611488, 31.19962993084977398, 12.30130330100619673 ) ) ;
#3589=CARTESIAN_POINT ( 'NONE',  ( -16.47274440071381107, 31.95215739789422571, 10.50982007662407725 ) ) ;
#3594=ORIENTED_EDGE ( 'NONE', *, *, #2938, .T. ) ;
#3597=CIRCLE ( 'NONE', #14907, 10.00000000000000000 ) ;
#3598=CARTESIAN_POINT ( 'NONE',  ( 17.54349574104648823, 125.4948194589026684, 4.999999999999997335 ) ) ;
#3601=DIRECTION ( 'NONE',  ( 1.000000000000000000, -0.000000000000000000, -0.000000000000000000 ) ) ;
#3602=ADVANCED_FACE ( 'NONE', ( #3311 ), #13526, .F. ) ;
#3606=CARTESIAN_POINT ( 'NONE',  ( 27.03183975455296917, 200.6580771142793083, 15.68801935549129745 ) ) ;
#3611=DIRECTION ( 'NONE',  ( -1.000000000000000000, 0.000000000000000000, 0.000000000000000000 ) ) ;
#3615=CARTESIAN_POINT ( 'NONE',  ( -48.00000000000000000, 171.6227766016838245, 0.000000000000000000 ) ) ;
#3620=CARTESIAN_POINT ( 'NONE',  ( -90.80384757729339640, 204.6227766016838245, 0.000000000000000000 ) ) ;
#3621=CARTESIAN_POINT ( 'NONE',  ( 48.00000000000000711, 159.6227766016838814, 8.071800142134975431 ) ) ;
#3623=ORIENTED_EDGE ( 'NONE', *, *, #8513, .T. ) ;
#3629=VERTEX_POINT ( 'NONE', #4075 ) ;
#3633=DIRECTION ( 'NONE',  ( 0.000000000000000000, 0.000000000000000000, -1.000000000000000000 ) ) ;
#3634=DIRECTION ( 'NONE',  ( 0.000000000000000000, 1.000000000000000000, 0.000000000000000000 ) ) ;
#3637=VECTOR ( 'NONE', #16218, 1000.000000000000114 ) ;
#3642=CARTESIAN_POINT ( 'NONE',  ( -12.22383789047832181, 18.00000000000231992, 8.612907111650555336 ) ) ;
#3643=CARTESIAN_POINT ( 'NONE',  ( -23.00000000000002132, 122.0000000000000142, 9.686291501015228178 ) ) ;
#3645=EDGE_LOOP ( 'NONE', ( #587, #13764, #622, #8083 ) ) ;
#3646=DIRECTION ( 'NONE',  ( 0.000000000000000000, 0.000000000000000000, 1.000000000000000000 ) ) ;
#3647=ORIENTED_EDGE ( 'NONE', *, *, #11674, .F. ) ;
#3650=DIRECTION ( 'NONE',  ( 0.000000000000000000, 0.000000000000000000, 1.000000000000000000 ) ) ;
#3653=CARTESIAN_POINT ( 'NONE',  ( 14.93242934743711992, 20.00000000000000000, 25.00000000000000000 ) ) ;
#3655=FACE_OUTER_BOUND ( 'NONE', #11920, .T. ) ;
#3657=EDGE_LOOP ( 'NONE', ( #4900, #6020, #8332, #11775 ) ) ;
#3658=EDGE_CURVE ( 'NONE', #2441, #5035, #9555, .T. ) ;
#3659=ADVANCED_FACE ( 'NONE', ( #10441 ), #8137, .F. ) ;
#3661=LINE ( 'NONE', #7635, #5918 ) ;
#3670=EDGE_LOOP ( 'NONE', ( #6155, #6339, #8460 ) ) ;
#3673=EDGE_LOOP ( 'NONE', ( #488, #16999, #5436, #9273 ) ) ;
#3675=ORIENTED_EDGE ( 'NONE', *, *, #4965, .F. ) ;
#3676=VECTOR ( 'NONE', #6174, 1000.000000000000000 ) ;
#3677=AXIS2_PLACEMENT_3D ( 'NONE', #13627, #16196, #10953 ) ;
#3680=VECTOR ( 'NONE', #7873, 1000.000000000000000 ) ;
#3681=ORIENTED_EDGE ( 'NONE', *, *, #2366, .F. ) ;
#3682=CARTESIAN_POINT ( 'NONE',  ( -16.22141882056480355, 32.74469488918423821, 6.141726134091478606 ) ) ;
#3685=CARTESIAN_POINT ( 'NONE',  ( 13.63270490666629975, 138.8028880870465969, 3.449993069226409581 ) ) ;
#3687=CARTESIAN_POINT ( 'NONE',  ( 20.85969470496125666, 141.7883037112096929, 14.11015612222007398 ) ) ;
#3691=VECTOR ( 'NONE', #4231, 1000.000000000000000 ) ;
#3695=CARTESIAN_POINT ( 'NONE',  ( 28.44010998145314417, 201.3777828775944272, 14.27084532960636309 ) ) ;
#3701=ORIENTED_EDGE ( 'NONE', *, *, #16801, .T. ) ;
#3702=CARTESIAN_POINT ( 'NONE',  ( -80.93218705276601099, 141.7051482704754335, 13.92628470286629749 ) ) ;
#3708=VERTEX_POINT ( 'NONE', #16209 ) ;
#3709=PLANE ( 'NONE',  #10946 ) ;
#3716=ORIENTED_EDGE ( 'NONE', *, *, #1544, .T. ) ;
#3718=CARTESIAN_POINT ( 'NONE',  ( 196.0000000000000000, 187.6227766016837961, 10.00000337241049309 ) ) ;
#3722=ORIENTED_EDGE ( 'NONE', *, *, #17017, .F. ) ;
#3723=DIRECTION ( 'NONE',  ( 0.000000000000000000, 0.000000000000000000, -1.000000000000000000 ) ) ;
#3724=DIRECTION ( 'NONE',  ( -1.000000000000000000, -0.000000000000000000, -0.000000000000000000 ) ) ;
#3725=VECTOR ( 'NONE', #11254, 1000.000000000000000 ) ;
#3727=CARTESIAN_POINT ( 'NONE',  ( 30.00000000000000355, 196.6227766016838245, 10.00000000000000178 ) ) ;
#3730=CARTESIAN_POINT ( 'NONE',  ( -23.66837786582113878, 18.00000000000000000, 17.32703391568840345 ) ) ;
#3731=CARTESIAN_POINT ( 'NONE',  ( 30.00000000000000355, 196.6227766016838245, 0.000000000000000000 ) ) ;
#3734=CARTESIAN_POINT ( 'NONE',  ( 48.00000000000000711, 191.6227766016837677, 8.071800142134975431 ) ) ;
#3740=CARTESIAN_POINT ( 'NONE',  ( -7.379000772444995526, 20.00000000000000000, 25.00000000000000000 ) ) ;
#3741=CARTESIAN_POINT ( 'NONE',  ( 48.00000000000000711, 167.6227766016838814, 19.42820660268601074 ) ) ;
#3744=CYLINDRICAL_SURFACE ( 'NONE', #14309, 2.500000000000000444 ) ;
#3750=ORIENTED_EDGE ( 'NONE', *, *, #12229, .T. ) ;
#3752=CARTESIAN_POINT ( 'NONE',  ( -38.00000000000000000, 20.00000000000000000, 30.00000000000000355 ) ) ;
#3764=CARTESIAN_POINT ( 'NONE',  ( 31.20232444244219394, 18.00000000000000000, 16.65183244245019623 ) ) ;
#3767=FACE_OUTER_BOUND ( 'NONE', #9660, .T. ) ;
#3770=CARTESIAN_POINT ( 'NONE',  ( 33.88556156013721932, 18.00000000000000000, 11.42442012027869858 ) ) ;
#3772=VERTEX_POINT ( 'NONE', #4163 ) ;
#3774=CARTESIAN_POINT ( 'NONE',  ( 34.58999572048171700, 198.6265692133321465, 18.97388360722740686 ) ) ;
#3775=EDGE_LOOP ( 'NONE', ( #3681, #9389 ) ) ;
#3780=CARTESIAN_POINT ( 'NONE',  ( 34.93420767853316988, 30.00000000000000000, 0.000000000000000000 ) ) ;
#3784=EDGE_LOOP ( 'NONE', ( #8150, #728, #10938 ) ) ;
#3785=CARTESIAN_POINT ( 'NONE',  ( -45.00000000000000000, 130.0000000000000000, 15.00000000000000000 ) ) ;
#3787=EDGE_CURVE ( 'NONE', #11737, #5404, #11814, .T. ) ;
#3790=EDGE_CURVE ( 'NONE', #3368, #10746, #2205, .T. ) ;
#3796=VERTEX_POINT ( 'NONE', #16648 ) ;
#3803=DIRECTION ( 'NONE',  ( 1.000000000000000000, 0.000000000000000000, 0.000000000000000000 ) ) ;
#3805=LINE ( 'NONE', #1237, #3298 ) ;
#3806=DIRECTION ( 'NONE',  ( -1.000000000000000000, 0.000000000000000000, 0.000000000000000000 ) ) ;
#3808=AXIS2_PLACEMENT_3D ( 'NONE', #8012, #6427, #17224 ) ;
#3812=AXIS2_PLACEMENT_3D ( 'NONE', #16580, #16674, #291 ) ;
#3814=EDGE_CURVE ( 'NONE', #14287, #5825, #4484, .T. ) ;
#3817=CARTESIAN_POINT ( 'NONE',  ( -82.50000000000002842, 146.6227766016838245, 10.00000000000000178 ) ) ;
#3818=ORIENTED_EDGE ( 'NONE', *, *, #8673, .F. ) ;
#3825=EDGE_CURVE ( 'NONE', #3708, #9609, #6987, .T. ) ;
#3826=CARTESIAN_POINT ( 'NONE',  ( 14.24850047812951104, 138.6393229685333779, 3.919138222309279218 ) ) ;
#3828=ORIENTED_EDGE ( 'NONE', *, *, #9046, .F. ) ;
#3829=STYLED_ITEM ( 'NONE', ( #7859 ), #11216 ) ;
#3830=CARTESIAN_POINT ( 'NONE',  ( 17.53546816055562374, 19.99999999999999645, 24.87355917367628422 ) ) ;
#3833=EDGE_LOOP ( 'NONE', ( #9654, #1189, #9148, #16548, #14428, #10658, #5494 ) ) ;
#3837=ADVANCED_FACE ( 'NONE', ( #11056 ), #8398, .F. ) ;
#3840=VERTEX_POINT ( 'NONE', #1847 ) ;
#3842=VECTOR ( 'NONE', #6700, 1000.000000000000000 ) ;
#3845=CARTESIAN_POINT ( 'NONE',  ( 49.99999999999998579, 183.6227766016837961, 8.071800142134975431 ) ) ;
#3847=VECTOR ( 'NONE', #6109, 1000.000000000000000 ) ;
#3849=ORIENTED_EDGE ( 'NONE', *, *, #2108, .F. ) ;
#3853=CIRCLE ( 'NONE', #13744, 2.500000000000000444 ) ;
#3856=CARTESIAN_POINT ( 'NONE',  ( -9.527527117355448993, 30.70225384978374450, 12.78416694138776855 ) ) ;
#3858=CARTESIAN_POINT ( 'NONE',  ( -17.03105419742079363, 32.06459626301238330, 9.633022903854756791 ) ) ;
#3861=CARTESIAN_POINT ( 'NONE',  ( 20.28823715622366919, 18.00000000000000000, 11.10707270023369730 ) ) ;
#3863=CARTESIAN_POINT ( 'NONE',  ( -78.11096775391246183, 151.2561509761041805, 25.96550485207006886 ) ) ;
#3864=EDGE_CURVE ( 'NONE', #1301, #9238, #2786, .T. ) ;
#3866=CARTESIAN_POINT ( 'NONE',  ( 24.26130280265436667, 140.5733633045254578, 11.19213049117091785 ) ) ;
#3867=CARTESIAN_POINT ( 'NONE',  ( 34.93420767853316988, 20.00000000000000000, 15.00000000000000000 ) ) ;
#3868=CARTESIAN_POINT ( 'NONE',  ( -22.99999999999999289, 90.00000000000000000, 15.00000000000000000 ) ) ;
#3870=CARTESIAN_POINT ( 'NONE',  ( 24.41053355130577884, 29.87514852601161763, 8.212591972297857978 ) ) ;
#3872=CARTESIAN_POINT ( 'NONE',  ( 15.00000000000000000, 191.6227766016837961, -1.224646799147353454E-15 ) ) ;
#3876=CARTESIAN_POINT ( 'NONE',  ( 29.85838552320831951, 201.6221756766237831, 13.74903839801206296 ) ) ;
#3879=DIRECTION ( 'NONE',  ( 0.000000000000000000, 0.000000000000000000, 1.000000000000000000 ) ) ;
#3880=ORIENTED_EDGE ( 'NONE', *, *, #16098, .T. ) ;
#3881=CARTESIAN_POINT ( 'NONE',  ( -79.76724320816964564, 141.6224873770942736, 13.74709594552941105 ) ) ;
#3882=CARTESIAN_POINT ( 'NONE',  ( 48.00000000000000711, 167.6227766016838530, 3.071800142134975431 ) ) ;
#3885=AXIS2_PLACEMENT_3D ( 'NONE', #14870, #7084, #10803 ) ;
#3890=DIRECTION ( 'NONE',  ( 2.312964634635742464E-16, 0.000000000000000000, -1.000000000000000000 ) ) ;
#3902=CYLINDRICAL_SURFACE ( 'NONE', #4468, 20.00000000000000355 ) ;
#3904=ADVANCED_FACE ( 'NONE', ( #8491 ), #13815, .T. ) ;
#3906=DIRECTION ( 'NONE',  ( 0.000000000000000000, 1.000000000000000000, 0.000000000000000000 ) ) ;
#3917=ORIENTED_EDGE ( 'NONE', *, *, #16200, .T. ) ;
#3919=DIRECTION ( 'NONE',  ( 0.000000000000000000, 0.000000000000000000, -1.000000000000000000 ) ) ;
#3922=CARTESIAN_POINT ( 'NONE',  ( -8.792264229871568304, 30.31966024794114745, 14.93731107458715357 ) ) ;
#3923=CARTESIAN_POINT ( 'NONE',  ( 12.74723713713078155, 129.4272226793184473, 10.49625762048852451 ) ) ;
#3925=AXIS2_PLACEMENT_3D ( 'NONE', #6291, #977, #2394 ) ;
#3926=CARTESIAN_POINT ( 'NONE',  ( 19.47274266584531333, 19.99999999999999645, 24.48069943974461538 ) ) ;
#3929=VERTEX_POINT ( 'NONE', #2193 ) ;
#3938=CARTESIAN_POINT ( 'NONE',  ( 25.00000000000000711, 146.6227766016838245, 21.54065922853802562 ) ) ;
#3943=AXIS2_PLACEMENT_3D ( 'NONE', #17491, #11017, #576 ) ;
#3944=CARTESIAN_POINT ( 'NONE',  ( -3.000000000000002665, 134.2062027339443944, 25.00000000000000000 ) ) ;
#3945=ORIENTED_EDGE ( 'NONE', *, *, #9705, .F. ) ;
#3946=VERTEX_POINT ( 'NONE', #4680 ) ;
#3947=VERTEX_POINT ( 'NONE', #6267 ) ;
#3948=DIRECTION ( 'NONE',  ( 1.000000000000000000, 0.000000000000000000, 0.000000000000000000 ) ) ;
#3950=EDGE_LOOP ( 'NONE', ( #9098, #10342, #13186, #12335 ) ) ;
#3953=CARTESIAN_POINT ( 'NONE',  ( -7.922882945419460476, 30.18055256556250399, 13.00000000000000355 ) ) ;
#3955=CARTESIAN_POINT ( 'NONE',  ( -15.37994105483213758, 31.72997864396344525, 11.82123051499886479 ) ) ;
#3957=DIRECTION ( 'NONE',  ( 1.000000000000000000, 0.000000000000000000, 0.000000000000000000 ) ) ;
#3958=CARTESIAN_POINT ( 'NONE',  ( -80.20949202752900931, 151.6222428389255015, 26.24840280143448368 ) ) ;
#3960=FACE_BOUND ( 'NONE', #4868, .T. ) ;
#3963=CARTESIAN_POINT ( 'NONE',  ( 23.79315516583586643, 18.00000000000000000, 22.94240041036162836 ) ) ;
#3964=DIRECTION ( 'NONE',  ( 1.000000000000000000, 0.000000000000000000, 0.000000000000000000 ) ) ;
#3965=ORIENTED_EDGE ( 'NONE', *, *, #17384, .F. ) ;
#3970=DIRECTION ( 'NONE',  ( -1.000000000000000000, -0.000000000000000000, -0.000000000000000000 ) ) ;
#3972=VERTEX_POINT ( 'NONE', #14322 ) ;
#3974=ORIENTED_EDGE ( 'NONE', *, *, #8981, .T. ) ;
#3975=EDGE_CURVE ( 'NONE', #14680, #16221, #10130, .T. ) ;
#3976=DIRECTION ( 'NONE',  ( -0.000000000000000000, -0.000000000000000000, -1.000000000000000000 ) ) ;
#3981=VECTOR ( 'NONE', #1011, 1000.000000000000000 ) ;
#3982=CARTESIAN_POINT ( 'NONE',  ( -22.79696676584442017, 19.99999999999999645, 18.34105320469109301 ) ) ;
#3984=DIRECTION ( 'NONE',  ( 1.000000000000000000, 0.000000000000000000, 0.000000000000000000 ) ) ;
#3985=LINE ( 'NONE', #2644, #4236 ) ;
#3987=CARTESIAN_POINT ( 'NONE',  ( -5.000000000000000888, 191.6227766016837961, -1.224646799147353454E-15 ) ) ;
#3991=EDGE_CURVE ( 'NONE', #5446, #14731, #14114, .T. ) ;
#3995=DIRECTION ( 'NONE',  ( 0.000000000000000000, 0.000000000000000000, 1.000000000000000000 ) ) ;
#3999=DIRECTION ( 'NONE',  ( -1.000000000000000000, -0.000000000000000000, -0.000000000000000000 ) ) ;
#4000=CARTESIAN_POINT ( 'NONE',  ( -3.000000000000000888, 154.3022685259950038, 9.999999999999900524 ) ) ;
#4006=AXIS2_PLACEMENT_3D ( 'NONE', #12522, #386, #16602 ) ;
#4008=CYLINDRICAL_SURFACE ( 'NONE', #13003, 2.500000000000000444 ) ;
#4012=ORIENTED_EDGE ( 'NONE', *, *, #6850, .F. ) ;
#4014=CARTESIAN_POINT ( 'NONE',  ( 27.99999999999998224, 9.999999999999998224, 10.00000000000000178 ) ) ;
#4017=CARTESIAN_POINT ( 'NONE',  ( -16.41264213764281976, 19.99999999999999645, 23.02790928165778794 ) ) ;
#4018=CARTESIAN_POINT ( 'NONE',  ( 14.40670567839409344, 127.3124839991112083, 8.619616438334361419 ) ) ;
#4022=DIRECTION ( 'NONE',  ( 0.000000000000000000, -0.8660254037844413721, 0.4999999999999953371 ) ) ;
#4027=ORIENTED_EDGE ( 'NONE', *, *, #5596, .F. ) ;
#4028=CARTESIAN_POINT ( 'NONE',  ( 29.20274480926571314, 151.5627461462769929, 26.20297826401937158 ) ) ;
#4032=FACE_OUTER_BOUND ( 'NONE', #3784, .T. ) ;
#4036=ORIENTED_EDGE ( 'NONE', *, *, #14985, .F. ) ;
#4037=CARTESIAN_POINT ( 'NONE',  ( 12.89436750745977278, 141.9634372303913779, 18.58317047499899743 ) ) ;
#4040=ORIENTED_EDGE ( 'NONE', *, *, #13391, .T. ) ;
#4043=CYLINDRICAL_SURFACE ( 'NONE', #11282, 5.000000000000000888 ) ;
#4045=CARTESIAN_POINT ( 'NONE',  ( -76.34554854693054438, 150.0509117818997709, 24.97535314687243613 ) ) ;
#4047=CARTESIAN_POINT ( 'NONE',  ( 30.00000000000000355, 196.6227766016838245, 0.000000000000000000 ) ) ;
#4049=CARTESIAN_POINT ( 'NONE',  ( 13.34250444320487361, 130.4016344817123070, 12.56142338728217744 ) ) ;
#4050=CARTESIAN_POINT ( 'NONE',  ( 28.15871609335591685, 18.00000000000000000, 20.05978710182010971 ) ) ;
#4051=DIRECTION ( 'NONE',  ( -0.000000000000000000, -0.000000000000000000, -1.000000000000000000 ) ) ;
#4054=VERTEX_POINT ( 'NONE', #15646 ) ;
#4057=ORIENTED_EDGE ( 'NONE', *, *, #658, .T. ) ;
#4061=CYLINDRICAL_SURFACE ( 'NONE', #5208, 10.00000000000000178 ) ;
#4062=EDGE_LOOP ( 'NONE', ( #9056, #14926, #4927, #6454 ) ) ;
#4067=SURFACE_STYLE_FILL_AREA ( #5397 ) ;
#4070=CARTESIAN_POINT ( 'NONE',  ( -80.00000000000001421, 196.6227766016838245, 0.000000000000000000 ) ) ;
#4071=CARTESIAN_POINT ( 'NONE',  ( -27.98221281347032274, 30.00000000000000000, 4.999999999999996447 ) ) ;
#4072=ORIENTED_EDGE ( 'NONE', *, *, #10834, .F. ) ;
#4075=CARTESIAN_POINT ( 'NONE',  ( -18.25212770525997286, 32.30769230769230660, 4.999999999999999112 ) ) ;
#4076=CARTESIAN_POINT ( 'NONE',  ( -80.00000000000001421, 196.6227766016838245, 11.50215154306610188 ) ) ;
#4084=ADVANCED_FACE ( 'NONE', ( #9178 ), #7676, .T. ) ;
#4085=VECTOR ( 'NONE', #5468, 1000.000000000000000 ) ;
#4086=VERTEX_POINT ( 'NONE', #5025 ) ;
#4087=CARTESIAN_POINT ( 'NONE',  ( 48.00000000000000711, 159.6227766016838814, 3.071800142134975431 ) ) ;
#4090=CARTESIAN_POINT ( 'NONE',  ( -48.00000000000000000, 171.6227766016838245, 0.000000000000000000 ) ) ;
#4094=CARTESIAN_POINT ( 'NONE',  ( 14.40174056114590151, 138.5906827818587885, 4.212836247846050597 ) ) ;
#4095=ORIENTED_EDGE ( 'NONE', *, *, #2804, .T. ) ;
#4096=CARTESIAN_POINT ( 'NONE',  ( 21.98114852961611376, 19.99999999999999645, 23.72829316725777460 ) ) ;
#4097=VECTOR ( 'NONE', #11255, 1000.000000000000000 ) ;
#4100=CARTESIAN_POINT ( 'NONE',  ( 196.0000000000000000, 171.6227766016838245, 15.00000337241049131 ) ) ;
#4102=DIRECTION ( 'NONE',  ( -1.000000000000000000, -0.000000000000000000, -0.000000000000000000 ) ) ;
#4105=DIRECTION ( 'NONE',  ( -0.000000000000000000, -0.000000000000000000, -1.000000000000000000 ) ) ;
#4107=CARTESIAN_POINT ( 'NONE',  ( -34.99999999999999289, 120.0000000000000284, 15.00000000000000000 ) ) ;
#4110=CARTESIAN_POINT ( 'NONE',  ( -5.000000000000000888, 206.6227766016838245, -2.143131898507868248E-15 ) ) ;
#4112=ORIENTED_EDGE ( 'NONE', *, *, #13394, .T. ) ;
#4113=FACE_OUTER_BOUND ( 'NONE', #12666, .T. ) ;
#4114=ORIENTED_EDGE ( 'NONE', *, *, #1992, .F. ) ;
#4115=DIRECTION ( 'NONE',  ( -0.000000000000000000, -0.000000000000000000, -1.000000000000000000 ) ) ;
#4118=AXIS2_PLACEMENT_3D ( 'NONE', #13527, #3070, #9617 ) ;
#4119=DIRECTION ( 'NONE',  ( -0.000000000000000000, -0.000000000000000000, -1.000000000000000000 ) ) ;
#4120=CARTESIAN_POINT ( 'NONE',  ( -100.0000000000000000, 136.6227766016838245, 0.000000000000000000 ) ) ;
#4121=CARTESIAN_POINT ( 'NONE',  ( -75.16806474348092593, 147.9395323639053856, 22.98372036160737153 ) ) ;
#4123=ORIENTED_EDGE ( 'NONE', *, *, #1819, .T. ) ;
#4125=CARTESIAN_POINT ( 'NONE',  ( 16.03791926353974162, 127.7299327228906520, 9.742640703122631862 ) ) ;
#4126=FACE_OUTER_BOUND ( 'NONE', #10455, .T. ) ;
#4131=AXIS2_PLACEMENT_3D ( 'NONE', #11182, #2063, #12864 ) ;
#4145=ORIENTED_EDGE ( 'NONE', *, *, #13237, .T. ) ;
#4148=DIRECTION ( 'NONE',  ( -1.000000000000000000, 0.000000000000000000, 0.000000000000000000 ) ) ;
#4149=PLANE ( 'NONE',  #4813 ) ;
#4155=DIRECTION ( 'NONE',  ( -0.000000000000000000, -0.000000000000000000, -1.000000000000000000 ) ) ;
#4157=VECTOR ( 'NONE', #1503, 1000.000000000000000 ) ;
#4163=CARTESIAN_POINT ( 'NONE',  ( 40.00000000000000000, 20.00000000000000000, 0.000000000000000000 ) ) ;
#4164=CARTESIAN_POINT ( 'NONE',  ( 29.81269655378473971, 191.6224348813835263, 26.24906986711105716 ) ) ;
#4168=CARTESIAN_POINT ( 'NONE',  ( -22.99999999999998224, 10.00000000000000000, 35.00200000000000244 ) ) ;
#4171=ORIENTED_EDGE ( 'NONE', *, *, #2170, .F. ) ;
#4177=ORIENTED_EDGE ( 'NONE', *, *, #8736, .F. ) ;
#4178=CARTESIAN_POINT ( 'NONE',  ( -14.24512928960374225, 20.00000000000229505, 9.752520130898352235 ) ) ;
#4186=EDGE_LOOP ( 'NONE', ( #13901, #2845, #9933, #6077, #11937, #10823 ) ) ;
#4190=CARTESIAN_POINT ( 'NONE',  ( 40.00000000000000711, 138.6227766016838245, 6.062001655779397722E-15 ) ) ;
#4194=CARTESIAN_POINT ( 'NONE',  ( 27.58881406714485252, 151.0069623973649584, 25.76819119792229174 ) ) ;
#4195=ORIENTED_EDGE ( 'NONE', *, *, #15421, .F. ) ;
#4196=LINE ( 'NONE', #14987, #7598 ) ;
#4197=FACE_OUTER_BOUND ( 'NONE', #7749, .T. ) ;
#4206=CARTESIAN_POINT ( 'NONE',  ( 49.99999999999998579, 191.6227766016837677, 5.571800142134975431 ) ) ;
#4211=DIRECTION ( 'NONE',  ( 0.000000000000000000, 0.000000000000000000, -1.000000000000000000 ) ) ;
#4217=FACE_OUTER_BOUND ( 'NONE', #1033, .T. ) ;
#4218=CARTESIAN_POINT ( 'NONE',  ( 9.103003883573421717, 133.2684780490642709, 14.60854014130129030 ) ) ;
#4221=PLANE ( 'NONE',  #5823 ) ;
#4222=ORIENTED_EDGE ( 'NONE', *, *, #13115, .T. ) ;
#4224=CIRCLE ( 'NONE', #1391, 33.00000000000000000 ) ;
#4230=EDGE_LOOP ( 'NONE', ( #15653, #6412, #3849, #13385 ) ) ;
#4231=DIRECTION ( 'NONE',  ( 0.000000000000000000, -1.000000000000000000, -0.000000000000000000 ) ) ;
#4236=VECTOR ( 'NONE', #1407, 1000.000000000000000 ) ;
#4244=FACE_OUTER_BOUND ( 'NONE', #12879, .T. ) ;
#4245=CARTESIAN_POINT ( 'NONE',  ( -68.00000000000000000, 154.3022685259950038, 9.999999999999900524 ) ) ;
#4246=AXIS2_PLACEMENT_3D ( 'NONE', #6261, #11823, #14668 ) ;
#4247=AXIS2_PLACEMENT_3D ( 'NONE', #3528, #11663, #6273 ) ;
#4248=EDGE_LOOP ( 'NONE', ( #1288, #4456, #10497, #14437 ) ) ;
#4252=EDGE_CURVE ( 'NONE', #5181, #2062, #16080, .T. ) ;
#4253=DIRECTION ( 'NONE',  ( -1.000000000000000000, 0.000000000000000000, 0.000000000000000000 ) ) ;
#4257=EDGE_CURVE ( 'NONE', #2548, #5131, #11119, .T. ) ;
#4264=ORIENTED_EDGE ( 'NONE', *, *, #14345, .F. ) ;
#4269=CARTESIAN_POINT ( 'NONE',  ( -16.77496435665412733, 32.01311153724419967, 10.06041171812362300 ) ) ;
#4275=VERTEX_POINT ( 'NONE', #5467 ) ;
#4280=CARTESIAN_POINT ( 'NONE',  ( -100.0000000000000000, 120.0000000000000284, 6.000000000000001776 ) ) ;
#4281=ORIENTED_EDGE ( 'NONE', *, *, #8513, .F. ) ;
#4286=CARTESIAN_POINT ( 'NONE',  ( -48.00000000000000000, 143.0439382767972347, 16.49999999999984368 ) ) ;
#4288=DIRECTION ( 'NONE',  ( 0.000000000000000000, 1.000000000000000000, 0.000000000000000000 ) ) ;
#4289=VERTEX_POINT ( 'NONE', #407 ) ;
#4294=CARTESIAN_POINT ( 'NONE',  ( 6.134011831684060390, 139.5514275721929209, 14.99999999999999822 ) ) ;
#4296=DIRECTION ( 'NONE',  ( -1.000000000000000000, -0.000000000000000000, -0.000000000000000000 ) ) ;
#4298=DIRECTION ( 'NONE',  ( 0.000000000000000000, 0.000000000000000000, 1.000000000000000000 ) ) ;
#4299=DIRECTION ( 'NONE',  ( -0.000000000000000000, -0.000000000000000000, 1.000000000000000000 ) ) ;
#4300=CARTESIAN_POINT ( 'NONE',  ( 19.47274266584701508, 18.00000000000000000, 24.48069943974689266 ) ) ;
#4302=FACE_OUTER_BOUND ( 'NONE', #3673, .T. ) ;
#4304=EDGE_CURVE ( 'NONE', #7251, #16894, #5628, .T. ) ;
#4307=CARTESIAN_POINT ( 'NONE',  ( -25.00000000000000000, 120.0000000000000426, 10.85786437626905077 ) ) ;
#4309=CARTESIAN_POINT ( 'NONE',  ( 35.00000000000000711, 146.6227766016838245, 21.54065922853802562 ) ) ;
#4310=PRODUCT_DEFINITION_CONTEXT ( 'detailed design', #7096, 'design' ) ;
#4311=ORIENTED_EDGE ( 'NONE', *, *, #2897, .T. ) ;
#4315=FACE_OUTER_BOUND ( 'NONE', #10906, .T. ) ;
#4317=DIRECTION ( 'NONE',  ( 1.000000000000000000, -0.000000000000000000, -0.000000000000000000 ) ) ;
#4318=CARTESIAN_POINT ( 'NONE',  ( -68.00000000000000000, 171.6227766016838245, 0.000000000000000000 ) ) ;
#4320=VERTEX_POINT ( 'NONE', #14300 ) ;
#4323=CARTESIAN_POINT ( 'NONE',  ( -22.93725393319378369, 20.00000000000004263, 5.999999999999992895 ) ) ;
#4334=CARTESIAN_POINT ( 'NONE',  ( 29.61664150470813794, 191.6335950462332107, 26.24057872661396118 ) ) ;
#4337=DIRECTION ( 'NONE',  ( -1.000000000000000000, -0.000000000000000000, -0.000000000000000000 ) ) ;
#4342=ORIENTED_EDGE ( 'NONE', *, *, #4681, .T. ) ;
#4343=DIRECTION ( 'NONE',  ( -0.000000000000000000, -0.000000000000000000, 1.000000000000000000 ) ) ;
#4350=FACE_OUTER_BOUND ( 'NONE', #2417, .T. ) ;
#4352=EDGE_CURVE ( 'NONE', #9170, #3772, #1917, .T. ) ;
#4358=DIRECTION ( 'NONE',  ( 0.000000000000000000, -1.000000000000000000, -8.673617379884035472E-17 ) ) ;
#4367=ADVANCED_FACE ( 'NONE', ( #12626 ), #11640, .T. ) ;
#4368=LINE ( 'NONE', #4110, #7791 ) ;
#4371=LINE ( 'NONE', #9851, #1577 ) ;
#4375=CARTESIAN_POINT ( 'NONE',  ( 16.34705933256455879, 136.9208395216682561, 6.505922558274784606 ) ) ;
#4377=EDGE_CURVE ( 'NONE', #3947, #15613, #9863, .T. ) ;
#4381=CARTESIAN_POINT ( 'NONE',  ( 15.58935537591275811, 125.0306660307430349, 3.338448778865417577 ) ) ;
#4383=CARTESIAN_POINT ( 'NONE',  ( 25.49876332522149625, 18.00000000000000000, 21.99427390110736624 ) ) ;
#4387=DIRECTION ( 'NONE',  ( -0.000000000000000000, -0.000000000000000000, -1.000000000000000000 ) ) ;
#4398=AXIS2_PLACEMENT_3D ( 'NONE', #6846, #12236, #106 ) ;
#4402=EDGE_CURVE ( 'NONE', #11461, #1227, #5065, .T. ) ;
#4403=DIRECTION ( 'NONE',  ( 0.000000000000000000, 0.000000000000000000, -1.000000000000000000 ) ) ;
#4407=DIRECTION ( 'NONE',  ( 0.000000000000000000, 0.000000000000000000, 1.000000000000000000 ) ) ;
#4410=ORIENTED_EDGE ( 'NONE', *, *, #11046, .T. ) ;
#4411=CARTESIAN_POINT ( 'NONE',  ( 27.04340649081008507, 142.5787592618052599, 15.67196037041395940 ) ) ;
#4412=CARTESIAN_POINT ( 'NONE',  ( 30.00000000000000355, 196.6227766016838245, 0.000000000000000000 ) ) ;
#4413=LINE ( 'NONE', #14064, #13591 ) ;
#4415=AXIS2_PLACEMENT_3D ( 'NONE', #13143, #10390, #5003 ) ;
#4420=DIRECTION ( 'NONE',  ( 1.000000000000000000, 0.000000000000000000, 0.000000000000000000 ) ) ;
#4424=VECTOR ( 'NONE', #16501, 1000.000000000000000 ) ;
#4425=VECTOR ( 'NONE', #10207, 1000.000000000000000 ) ;
#4426=DIRECTION ( 'NONE',  ( 0.000000000000000000, 0.000000000000000000, -1.000000000000000000 ) ) ;
#4427=AXIS2_PLACEMENT_3D ( 'NONE', #6238, #5893, #12968 ) ;
#4431=CARTESIAN_POINT ( 'NONE',  ( 22.88339857903067198, 29.84310082762161187, 6.047897139192784266 ) ) ;
#4432=CARTESIAN_POINT ( 'NONE',  ( -84.47031951572937203, 198.8808217108462770, 18.60648811928366442 ) ) ;
#4433=CARTESIAN_POINT ( 'NONE',  ( -80.00000000000002842, 146.6227766016838245, 11.50215154306610188 ) ) ;
#4434=VERTEX_POINT ( 'NONE', #6074 ) ;
#4435=EDGE_LOOP ( 'NONE', ( #9208, #8069, #14147, #3246, #3176, #5592, #2473, #8334, #15358 ) ) ;
#4436=LINE ( 'NONE', #8583, #2977 ) ;
#4441=EDGE_CURVE ( 'NONE', #11986, #15706, #252, .T. ) ;
#4442=CARTESIAN_POINT ( 'NONE',  ( -24.81085081035532269, 19.99999999999999645, 15.69149817756037457 ) ) ;
#4443=AXIS2_PLACEMENT_3D ( 'NONE', #7333, #10240, #7156 ) ;
#4447=CARTESIAN_POINT ( 'NONE',  ( -24.80114670877659222, 18.00000000000000000, 15.70637264050927051 ) ) ;
#4450=FACE_OUTER_BOUND ( 'NONE', #1831, .T. ) ;
#4455=DIRECTION ( 'NONE',  ( 0.000000000000000000, -1.000000000000000000, 6.123233995736762338E-17 ) ) ;
#4456=ORIENTED_EDGE ( 'NONE', *, *, #5294, .T. ) ;
#4460=CARTESIAN_POINT ( 'NONE',  ( 0.000000000000000000, 18.00000000000000355, 0.000000000000000000 ) ) ;
#4462=VERTEX_POINT ( 'NONE', #15289 ) ;
#4463=EDGE_CURVE ( 'NONE', #6774, #3061, #16668, .T. ) ;
#4464=DIRECTION ( 'NONE',  ( 1.000000000000000000, 0.000000000000000000, 0.000000000000000000 ) ) ;
#4465=CIRCLE ( 'NONE', #15476, 2.500000000000000000 ) ;
#4466=DIRECTION ( 'NONE',  ( 8.673617379884037937E-17, 0.000000000000000000, -1.000000000000000000 ) ) ;
#4467=CARTESIAN_POINT ( 'NONE',  ( 16.17648631192976794, 127.5693673001539992, 9.524520547909567370 ) ) ;
#4468=AXIS2_PLACEMENT_3D ( 'NONE', #2653, #10612, #7452 ) ;
#4473=EDGE_CURVE ( 'NONE', #3234, #17055, #6772, .T. ) ;
#4474=CARTESIAN_POINT ( 'NONE',  ( -84.53371403557255803, 194.4926179048318318, 23.79294127240568457 ) ) ;
#4476=CARTESIAN_POINT ( 'NONE',  ( 15.45450437963097912, 29.98942126207016301, 13.00000000000000178 ) ) ;
#4479=ORIENTED_EDGE ( 'NONE', *, *, #9881, .T. ) ;
#4483=DIRECTION ( 'NONE',  ( -1.156482317317868274E-16, 1.000000000000000000, 0.000000000000000000 ) ) ;
#4484=CIRCLE ( 'NONE', #12381, 5.000000000000000888 ) ;
#4487=VERTEX_POINT ( 'NONE', #1014 ) ;
#4488=CARTESIAN_POINT ( 'NONE',  ( 7.535032041484082121, 144.1839557648053187, 18.33333333253072794 ) ) ;
#4498=ORIENTED_EDGE ( 'NONE', *, *, #1705, .F. ) ;
#4501=CARTESIAN_POINT ( 'NONE',  ( -7.379000772445021283, 18.00000000000000000, 25.00000000000000355 ) ) ;
#4502=CARTESIAN_POINT ( 'NONE',  ( 25.00000000000000000, 196.6227766016838245, 35.00200000000000244 ) ) ;
#4503=TOROIDAL_SURFACE ( 'NONE', #9008, 740.0000000000000000, 10.00000000000000000 ) ;
#4506=DIRECTION ( 'NONE',  ( 0.000000000000000000, -1.000000000000000000, 6.123233995736762338E-17 ) ) ;
#4509=EDGE_LOOP ( 'NONE', ( #12223, #8545, #2346, #12909 ) ) ;
#4510=SURFACE_STYLE_FILL_AREA ( #9543 ) ;
#4511=CARTESIAN_POINT ( 'NONE',  ( 27.19159743497788284, 137.1791639268274992, 6.327035192214271575 ) ) ;
#4518=LINE ( 'NONE', #11232, #7823 ) ;
#4519=CARTESIAN_POINT ( 'NONE',  ( 18.93858299686282365, 29.91990340250987757, 11.93041869825017898 ) ) ;
#4520=LINE ( 'NONE', #7425, #10177 ) ;
#4526=EDGE_CURVE ( 'NONE', #12455, #12513, #10569, .T. ) ;
#4529=ADVANCED_FACE ( 'NONE', ( #5451 ), #11558, .F. ) ;
#4534=CIRCLE ( 'NONE', #13581, 20.00000000000000355 ) ;
#4538=CARTESIAN_POINT ( 'NONE',  ( -11.98734322101359240, 18.00000000000000355, 24.50584837321702736 ) ) ;
#4542=FACE_OUTER_BOUND ( 'NONE', #13861, .T. ) ;
#4544=ADVANCED_FACE ( 'NONE', ( #1545 ), #2793, .F. ) ;
#4547=DIRECTION ( 'NONE',  ( 0.000000000000000000, 0.000000000000000000, -1.000000000000000000 ) ) ;
#4550=CARTESIAN_POINT ( 'NONE',  ( -24.99999999999999289, 90.00000000000000000, 15.00000000000000000 ) ) ;
#4551=VERTEX_POINT ( 'NONE', #10760 ) ;
#4554=CARTESIAN_POINT ( 'NONE',  ( 27.47046887371370616, 136.6950068244141221, 2.596529902249163690 ) ) ;
#4555=CARTESIAN_POINT ( 'NONE',  ( 26.13287303778632165, 137.8093815885048627, 9.050576676228219597 ) ) ;
#4558=DIRECTION ( 'NONE',  ( 0.000000000000000000, 1.000000000000000000, 0.000000000000000000 ) ) ;
#4562=ADVANCED_FACE ( 'NONE', ( #8184 ), #4043, .T. ) ;
#4563=CARTESIAN_POINT ( 'NONE',  ( 19.16009641331746849, 29.91553747150882359, 11.79770956048753838 ) ) ;
#4567=DIRECTION ( 'NONE',  ( -0.000000000000000000, -0.000000000000000000, 1.000000000000000000 ) ) ;
#4570=ORIENTED_EDGE ( 'NONE', *, *, #14637, .F. ) ;
#4573=ORIENTED_EDGE ( 'NONE', *, *, #5497, .F. ) ;
#4577=CARTESIAN_POINT ( 'NONE',  ( 12.89436750745977989, 143.6582566230365501, 17.52127501928458031 ) ) ;
#4580=VECTOR ( 'NONE', #5769, 1000.000000000000000 ) ;
#4583=CYLINDRICAL_SURFACE ( 'NONE', #12311, 2.500000000000000444 ) ;
#4587=CARTESIAN_POINT ( 'NONE',  ( 25.98421795186086314, 143.6297497249236130, 17.48070775079459338 ) ) ;
#4589=LINE ( 'NONE', #9969, #9050 ) ;
#4591=CARTESIAN_POINT ( 'NONE',  ( 14.93242934743710393, 30.00000000000000000, 25.00000000000000000 ) ) ;
#4593=EDGE_CURVE ( 'NONE', #16788, #11875, #17511, .T. ) ;
#4603=CARTESIAN_POINT ( 'NONE',  ( 37.99999999999998579, 18.00000000000000355, 28.00000000000001066 ) ) ;
#4604=ORIENTED_EDGE ( 'NONE', *, *, #2930, .F. ) ;
#4607=CARTESIAN_POINT ( 'NONE',  ( -84.88899566805817187, 197.8164829328480891, 20.09296681051160149 ) ) ;
#4609=VERTEX_POINT ( 'NONE', #12181 ) ;
#4610=ORIENTED_EDGE ( 'NONE', *, *, #2804, .F. ) ;
#4613=ORIENTED_EDGE ( 'NONE', *, *, #12667, .F. ) ;
#4614=DIRECTION ( 'NONE',  ( -0.000000000000000000, -0.000000000000000000, -1.000000000000000000 ) ) ;
#4619=CYLINDRICAL_SURFACE ( 'NONE', #13606, 5.000000000000004441 ) ;
#4620=ADVANCED_FACE ( 'NONE', ( #13677 ), #5624, .F. ) ;
#4625=EDGE_CURVE ( 'NONE', #5289, #8027, #9946, .T. ) ;
#4626=CARTESIAN_POINT ( 'NONE',  ( -7.379000772444995526, 30.00000000000000000, 13.00000000000000178 ) ) ;
#4631=ORIENTED_EDGE ( 'NONE', *, *, #12739, .F. ) ;
#4636=CARTESIAN_POINT ( 'NONE',  ( 34.93420767782698988, 19.99999999999999645, 6.321724734770472587 ) ) ;
#4638=ORIENTED_EDGE ( 'NONE', *, *, #1257, .F. ) ;
#4642=CARTESIAN_POINT ( 'NONE',  ( -27.98221281347037959, 30.00000000000000000, 0.000000000000000000 ) ) ;
#4643=DIRECTION ( 'NONE',  ( 1.000000000000000000, 0.000000000000000000, 0.000000000000000000 ) ) ;
#4649=CARTESIAN_POINT ( 'NONE',  ( -23.00000000000000000, 120.0000000000000284, 0.000000000000000000 ) ) ;
#4657=DIRECTION ( 'NONE',  ( -0.8571673013836867971, 0.000000000000000000, -0.5150380737757237481 ) ) ;
#4658=ORIENTED_EDGE ( 'NONE', *, *, #7378, .F. ) ;
#4660=CARTESIAN_POINT ( 'NONE',  ( 15.56337975240373872, 125.2134999403456135, 4.999999999999997335 ) ) ;
#4662=CYLINDRICAL_SURFACE ( 'NONE', #4676, 248.0000000000000000 ) ;
#4665=CARTESIAN_POINT ( 'NONE',  ( 27.92535256414491585, 142.0696621759509526, 14.68466941333283238 ) ) ;
#4666=DIRECTION ( 'NONE',  ( -1.000000000000000000, 0.000000000000000000, 0.000000000000000000 ) ) ;
#4667=FACE_OUTER_BOUND ( 'NONE', #4186, .T. ) ;
#4670=CIRCLE ( 'NONE', #16831, 27.69059892324149530 ) ;
#4671=CARTESIAN_POINT ( 'NONE',  ( -68.00000000000000000, 171.6227766016838245, 0.000000000000000000 ) ) ;
#4676=AXIS2_PLACEMENT_3D ( 'NONE', #9886, #11470, #1749 ) ;
#4679=CARTESIAN_POINT ( 'NONE',  ( -95.00000000000000000, 171.6227766016838245, 27.69059892324149530 ) ) ;
#4680=CARTESIAN_POINT ( 'NONE',  ( 48.00000000000000711, 155.6227766016839098, 10.00000337241049309 ) ) ;
#4681=EDGE_CURVE ( 'NONE', #647, #8265, #12257, .T. ) ;
#4683=B_SPLINE_CURVE_WITH_KNOTS ( 'NONE', 3,
 ( #3653, #12778, #14362, #10277, #736, #11358, #4721, #565, #2231, #13040, #1976, #6131, #3304, #11527, #12949, #4809, #6298, #11687, #17099, #10365, #15775, #16768, #10203, #7379, #9043 ),
 .UNSPECIFIED., .F., .F.,
 ( 4, 2, 2, 1, 2, 2, 2, 2, 2, 2, 2, 2, 4 ),
 ( 0.000000000000000000, 0.003937549356687076833, 0.005906324035030613949, 0.007875098713374151932, 0.009843873391717689048, 0.01181264807006122616, 0.01575019742674830733, 0.01771897210509184445, 0.01968774678343538503, 0.02362529614012245927, 0.02559407081846599985, 0.02756284549680953697, 0.03150039485349661467 ),
 .UNSPECIFIED. ) ;
#4685=EDGE_CURVE ( 'NONE', #14680, #13439, #11972, .T. ) ;
#4689=VECTOR ( 'NONE', #7580, 1000.000000000000000 ) ;
#4690=CARTESIAN_POINT ( 'NONE',  ( -84.18228968272714496, 199.3779494270211785, 17.85644994789933904 ) ) ;
#4694=ORIENTED_EDGE ( 'NONE', *, *, #2875, .F. ) ;
#4700=AXIS2_PLACEMENT_3D ( 'NONE', #7037, #2701, #11016 ) ;
#4707=CARTESIAN_POINT ( 'NONE',  ( -25.81900932159184592, 18.00000000000000000, 13.95463872937486194 ) ) ;
#4708=CARTESIAN_POINT ( 'NONE',  ( 25.49999999999998579, 9.999999999999998224, 0.000000000000000000 ) ) ;
#4711=VECTOR ( 'NONE', #9483, 1000.000000000000000 ) ;
#4712=ORIENTED_EDGE ( 'NONE', *, *, #8388, .T. ) ;
#4715=ORIENTED_EDGE ( 'NONE', *, *, #16713, .F. ) ;
#4716=LINE ( 'NONE', #6042, #11280 ) ;
#4721=CARTESIAN_POINT ( 'NONE',  ( 22.61491075001043782, 19.99999999999999645, 23.50024419593056635 ) ) ;
#4722=CARTESIAN_POINT ( 'NONE',  ( 19.93228116232496205, 29.93335004877557282, 13.66730128329526650 ) ) ;
#4724=B_SPLINE_CURVE_WITH_KNOTS ( 'NONE', 3,
 ( #6529, #2274, #17234, #17140, #869, #5109, #13346, #15820, #15991, #3606, #10315, #17054, #4923, #13078, #3695, #2547, #9169, #10238, #1207, #15724, #3876, #16982, #945, #10407, #7581, #2183, #13255, #7669, #6334, #15637, #3515, #9260, #2447, #8903, #11727, #6433, #5016, #6611, #3774, #17320, #9083, #14489 ),
 .UNSPECIFIED., .F., .F.,
 ( 4, 2, 2, 2, 2, 2, 2, 2, 2, 2, 2, 2, 2, 2, 2, 2, 2, 2, 2, 2, 4 ),
 ( 0.000000000000000000, 0.002803867404946438179, 0.004205801107419684590, 0.005607734809892931001, 0.007009668512366177412, 0.008411602214839424690, 0.009112569066076062207, 0.009813535917312697990, 0.01051450276854933551, 0.01086498619416765427, 0.01121546961978597302, 0.01156595304540429005, 0.01191643647102261228, 0.01261740332225922898, 0.01331837017349584741, 0.01401933702473246238, 0.01542127072720567843, 0.01682320442967889448, 0.01822513813215211401, 0.01962707183462532659, 0.02243093923957175523 ),
 .UNSPECIFIED. ) ;
#4725=EDGE_LOOP ( 'NONE', ( #8914, #2238, #16714, #1120 ) ) ;
#4726=DIRECTION ( 'NONE',  ( 0.000000000000000000, 0.000000000000000000, 1.000000000000000000 ) ) ;
#4737=ORIENTED_EDGE ( 'NONE', *, *, #13973, .F. ) ;
#4738=DIRECTION ( 'NONE',  ( 0.000000000000000000, 1.000000000000000000, 0.000000000000000000 ) ) ;
#4740=EDGE_CURVE ( 'NONE', #15841, #13489, #3661, .T. ) ;
#4741=EDGE_LOOP ( 'NONE', ( #2250, #16892, #13997, #7120 ) ) ;
#4742=ADVANCED_FACE ( 'NONE', ( #6303 ), #12958, .F. ) ;
#4744=EDGE_CURVE ( 'NONE', #3385, #15774, #9293, .T. ) ;
#4748=VERTEX_POINT ( 'NONE', #13046 ) ;
#4749=CARTESIAN_POINT ( 'NONE',  ( 27.50000000000001066, 146.6227766016838245, 10.00000000000000178 ) ) ;
#4751=CARTESIAN_POINT ( 'NONE',  ( 15.00000000000000000, 171.6227766016838245, 0.000000000000000000 ) ) ;
#4752=CARTESIAN_POINT ( 'NONE',  ( 8.630636718464335999, 133.1548047818457690, 12.68018750699619268 ) ) ;
#4753=DIRECTION ( 'NONE',  ( 1.000000000000000000, 0.000000000000000000, 0.000000000000000000 ) ) ;
#4754=CARTESIAN_POINT ( 'NONE',  ( 13.66341101666136382, 138.6227766017534293, 1.153153160045991887 ) ) ;
#4755=AXIS2_PLACEMENT_3D ( 'NONE', #8455, #12443, #481 ) ;
#4759=CARTESIAN_POINT ( 'NONE',  ( 25.00000000000000711, 146.6227766016838245, 21.54065922853802562 ) ) ;
#4760=DIRECTION ( 'NONE',  ( 0.000000000000000000, -1.000000000000000000, 6.123233995736762338E-17 ) ) ;
#4761=CYLINDRICAL_SURFACE ( 'NONE', #15843, 10.00000000000000178 ) ;
#4764=CARTESIAN_POINT ( 'NONE',  ( -100.0000000000000000, 100.0000000000000142, 6.000000000000000000 ) ) ;
#4771=ORIENTED_EDGE ( 'NONE', *, *, #7430, .T. ) ;
#4776=EDGE_LOOP ( 'NONE', ( #8635, #4095, #9894, #14047 ) ) ;
#4780=AXIS2_PLACEMENT_3D ( 'NONE', #6954, #13422, #9605 ) ;
#4783=ORIENTED_EDGE ( 'NONE', *, *, #12472, .F. ) ;
#4787=ORIENTED_EDGE ( 'NONE', *, *, #7866, .F. ) ;
#4788=EDGE_CURVE ( 'NONE', #13275, #15996, #1521, .T. ) ;
#4791=CYLINDRICAL_SURFACE ( 'NONE', #10620, 10.00000000000000178 ) ;
#4798=CARTESIAN_POINT ( 'NONE',  ( -12.73428483635922426, 18.00000000000460787, 6.504128904294631752 ) ) ;
#4802=CARTESIAN_POINT ( 'NONE',  ( 196.0000000000000000, 155.6227766016839098, 15.00000337241049486 ) ) ;
#4804=ORIENTED_EDGE ( 'NONE', *, *, #9391, .F. ) ;
#4809=CARTESIAN_POINT ( 'NONE',  ( 31.20890926080315353, 19.99999999999999289, 16.64259892333393154 ) ) ;
#4811=FACE_OUTER_BOUND ( 'NONE', #15003, .T. ) ;
#4813=AXIS2_PLACEMENT_3D ( 'NONE', #12279, #17336, #2645 ) ;
#4818=CARTESIAN_POINT ( 'NONE',  ( -75.00000000000001421, 196.3674529106260422, 21.83698684826043390 ) ) ;
#4820=EDGE_CURVE ( 'NONE', #15013, #12351, #17394, .T. ) ;
#4821=DIRECTION ( 'NONE',  ( 0.000000000000000000, 0.000000000000000000, 1.000000000000000000 ) ) ;
#4842=CARTESIAN_POINT ( 'NONE',  ( 22.73076297281406255, 29.84603606043824442, 6.815711530131156159 ) ) ;
#4843=EDGE_CURVE ( 'NONE', #978, #13751, #9458, .T. ) ;
#4844=DIRECTION ( 'NONE',  ( -1.000000000000000000, -0.000000000000000000, -0.000000000000000000 ) ) ;
#4846=ORIENTED_EDGE ( 'NONE', *, *, #11525, .F. ) ;
#4855=VERTEX_POINT ( 'NONE', #10898 ) ;
#4856=LINE ( 'NONE', #16731, #5377 ) ;
#4862=CARTESIAN_POINT ( 'NONE',  ( 30.00000000000001066, 146.6227766016838245, 10.00000000000000178 ) ) ;
#4864=VERTEX_POINT ( 'NONE', #7988 ) ;
#4865=ORIENTED_EDGE ( 'NONE', *, *, #8845, .F. ) ;
#4867=CARTESIAN_POINT ( 'NONE',  ( -725.0000000000000000, 19.99999999999995737, 15.00000000000000000 ) ) ;
#4868=EDGE_LOOP ( 'NONE', ( #11683, #4281 ) ) ;
#4876=CARTESIAN_POINT ( 'NONE',  ( -725.0000000000000000, 19.99999999999995737, 4.999999999999997335 ) ) ;
#4877=CARTESIAN_POINT ( 'NONE',  ( -14.94236098988382722, 32.37030496448370798, 9.276599271047366813 ) ) ;
#4878=FACE_OUTER_BOUND ( 'NONE', #292, .T. ) ;
#4881=LINE ( 'NONE', #4802, #14940 ) ;
#4884=DIRECTION ( 'NONE',  ( -0.000000000000000000, -0.000000000000000000, -1.000000000000000000 ) ) ;
#4887=CARTESIAN_POINT ( 'NONE',  ( 24.99836435517920918, 19.99999999999999289, 6.327826241642252825 ) ) ;
#4891=DIRECTION ( 'NONE',  ( 1.000000000000000000, 0.000000000000000000, -0.000000000000000000 ) ) ;
#4892=ADVANCED_FACE ( 'NONE', ( #3114 ), #14187, .T. ) ;
#4897=EDGE_LOOP ( 'NONE', ( #7562, #7940 ) ) ;
#4900=ORIENTED_EDGE ( 'NONE', *, *, #144, .T. ) ;
#4908=VERTEX_POINT ( 'NONE', #16576 ) ;
#4910=LINE ( 'NONE', #14652, #3981 ) ;
#4917=CYLINDRICAL_SURFACE ( 'NONE', #17179, 2.500000000000002220 ) ;
#4920=CARTESIAN_POINT ( 'NONE',  ( 19.94005785806629660, 29.93324777864367192, 13.66280195656096907 ) ) ;
#4922=LINE ( 'NONE', #7489, #4689 ) ;
#4923=CARTESIAN_POINT ( 'NONE',  ( 27.91212228340977930, 201.1698135001049650, 14.69689982759755154 ) ) ;
#4926=EDGE_CURVE ( 'NONE', #14446, #17286, #16671, .T. ) ;
#4927=ORIENTED_EDGE ( 'NONE', *, *, #12092, .F. ) ;
#4929=AXIS2_PLACEMENT_3D ( 'NONE', #14613, #7883, #13292 ) ;
#4932=VECTOR ( 'NONE', #10398, 1000.000000000000000 ) ;
#4935=CARTESIAN_POINT ( 'NONE',  ( 196.0000000000000000, 175.6227766016838245, 5.571800142134975431 ) ) ;
#4936=ORIENTED_EDGE ( 'NONE', *, *, #10276, .F. ) ;
#4937=DIRECTION ( 'NONE',  ( 1.000000000000000000, 0.000000000000000000, 0.000000000000000000 ) ) ;
#4940=CARTESIAN_POINT ( 'NONE',  ( 30.00000000000001066, 146.6227766016838245, 0.000000000000000000 ) ) ;
#4942=EDGE_LOOP ( 'NONE', ( #15594, #14816, #10409, #11286, #225, #12496 ) ) ;
#4943=MECHANICAL_DESIGN_GEOMETRIC_PRESENTATION_REPRESENTATION('',(#3829),#16558);
#4949=EDGE_LOOP ( 'NONE', ( #8589, #3192, #17048, #757 ) ) ;
#4952=ORIENTED_EDGE ( 'NONE', *, *, #790, .T. ) ;
#4956=CIRCLE ( 'NONE', #5808, 2.500000000000002220 ) ;
#4957=DIRECTION ( 'NONE',  ( -0.000000000000000000, -0.000000000000000000, -1.000000000000000000 ) ) ;
#4959=CARTESIAN_POINT ( 'NONE',  ( -12.51506868919167026, 17.99999999999883826, 7.695309128566540480 ) ) ;
#4960=CARTESIAN_POINT ( 'NONE',  ( -19.68629150101526903, 125.3137084989847807, 12.99999999999998401 ) ) ;
#4962=ORIENTED_EDGE ( 'NONE', *, *, #14013, .F. ) ;
#4965=EDGE_CURVE ( 'NONE', #2336, #8681, #13924, .T. ) ;
#4967=AXIS2_PLACEMENT_3D ( 'NONE', #15434, #7200, #8797 ) ;
#4973=VECTOR ( 'NONE', #13632, 1000.000000000000000 ) ;
#4974=CARTESIAN_POINT ( 'NONE',  ( 24.67949051125555826, 29.87169671703155771, 7.269639412668861489 ) ) ;
#4991=ORIENTED_EDGE ( 'NONE', *, *, #2990, .T. ) ;
#4993=VECTOR ( 'NONE', #11858, 1000.000000000000000 ) ;
#5003=DIRECTION ( 'NONE',  ( 0.000000000000000000, 1.000000000000000000, 0.000000000000000000 ) ) ;
#5005=CARTESIAN_POINT ( 'NONE',  ( 22.66736643345232949, 29.84725565559530480, 7.069278529401977984 ) ) ;
#5006=CARTESIAN_POINT ( 'NONE',  ( -85.00000000000000000, 147.1386660375792417, 22.13939837391654208 ) ) ;
#5008=DIRECTION ( 'NONE',  ( -0.000000000000000000, -0.000000000000000000, -1.000000000000000000 ) ) ;
#5011=DIRECTION ( 'NONE',  ( -1.000000000000000000, 0.000000000000000000, 0.000000000000000000 ) ) ;
#5012=CARTESIAN_POINT ( 'NONE',  ( 18.16062352778163813, 29.95676120085481386, 14.47054584901207619 ) ) ;
#5014=CIRCLE ( 'NONE', #14910, 33.00000000000000000 ) ;
#5015=EDGE_CURVE ( 'NONE', #11548, #11927, #10874, .T. ) ;
#5016=CARTESIAN_POINT ( 'NONE',  ( 34.17818013757652551, 199.3841150854655382, 17.84683500849086712 ) ) ;
#5017=VERTEX_POINT ( 'NONE', #2217 ) ;
#5021=AXIS2_PLACEMENT_3D ( 'NONE', #333, #3345, #14148 ) ;
#5023=CONICAL_SURFACE ( 'NONE', #13799, 2.499999999999998668, 1.029744260000002187 ) ;
#5025=CARTESIAN_POINT ( 'NONE',  ( -15.00000000000001421, 90.00000000000000000, 13.00000000000000000 ) ) ;
#5030=EDGE_CURVE ( 'NONE', #4908, #4748, #984, .T. ) ;
#5035=VERTEX_POINT ( 'NONE', #10265 ) ;
#5037=ORIENTED_EDGE ( 'NONE', *, *, #2622, .T. ) ;
#5044=CARTESIAN_POINT ( 'NONE',  ( -15.00000000000002665, 130.0000000000000000, 15.00000000000000000 ) ) ;
#5045=CARTESIAN_POINT ( 'NONE',  ( 30.00000000000001066, 146.6227766016838245, 0.000000000000000000 ) ) ;
#5047=CARTESIAN_POINT ( 'NONE',  ( -96.00000000000001421, 171.6227766016838245, 30.00000000000000000 ) ) ;
#5048=DIRECTION ( 'NONE',  ( 0.000000000000000000, -1.000000000000000000, 0.000000000000000000 ) ) ;
#5049=DIRECTION ( 'NONE',  ( -1.000000000000000000, -0.000000000000000000, -0.000000000000000000 ) ) ;
#5050=CARTESIAN_POINT ( 'NONE',  ( -9.925381735234770630, 18.00000000000231992, 11.63955885304398130 ) ) ;
#5051=EDGE_CURVE ( 'NONE', #11003, #13316, #7698, .T. ) ;
#5054=EDGE_CURVE ( 'NONE', #2062, #6313, #2388, .T. ) ;
#5055=DIRECTION ( 'NONE',  ( -1.000000000000000000, 0.000000000000000000, -5.782411586589356653E-16 ) ) ;
#5062=VECTOR ( 'NONE', #10747, 1000.000000000000000 ) ;
#5063=ORIENTED_EDGE ( 'NONE', *, *, #4402, .F. ) ;
#5064=CARTESIAN_POINT ( 'NONE',  ( -20.86241502029082184, 19.99999999999999645, 20.14618526196967352 ) ) ;
#5065=CIRCLE ( 'NONE', #1109, 2.499999999999998668 ) ;
#5066=CARTESIAN_POINT ( 'NONE',  ( 27.25143353317894324, 139.0964629073462220, 5.659441210211040740 ) ) ;
#5067=CARTESIAN_POINT ( 'NONE',  ( 18.16394926501914497, 19.99999999999886313, 14.51477632729204537 ) ) ;
#5068=ORIENTED_EDGE ( 'NONE', *, *, #15325, .F. ) ;
#5072=CARTESIAN_POINT ( 'NONE',  ( -80.00000000000002842, 146.6227766016838245, 0.000000000000000000 ) ) ;
#5074=CIRCLE ( 'NONE', #14971, 5.000000000000004441 ) ;
#5075=VERTEX_POINT ( 'NONE', #6560 ) ;
#5080=ORIENTED_EDGE ( 'NONE', *, *, #4257, .F. ) ;
#5083=AXIS2_PLACEMENT_3D ( 'NONE', #16709, #5724, #7628 ) ;
#5085=DIRECTION ( 'NONE',  ( -1.000000000000000000, -0.000000000000000000, -0.000000000000000000 ) ) ;
#5091=DIRECTION ( 'NONE',  ( -1.000000000000000000, 0.000000000000000000, 0.000000000000000000 ) ) ;
#5095=CARTESIAN_POINT ( 'NONE',  ( 21.87797949700605926, 29.86248177612424115, 9.008363892349379398 ) ) ;
#5096=CARTESIAN_POINT ( 'NONE',  ( 15.60228996707308191, 124.9392590765123998, 1.671679228207827439 ) ) ;
#5098=CARTESIAN_POINT ( 'NONE',  ( 27.42718951882975631, 138.9142741377072525, 4.446260193316556197 ) ) ;
#5099=AXIS2_PLACEMENT_3D ( 'NONE', #3741, #14531, #189 ) ;
#5100=AXIS2_PLACEMENT_3D ( 'NONE', #6256, #12898, #8823 ) ;
#5104=CIRCLE ( 'NONE', #6225, 2.500000000000002220 ) ;
#5106=ORIENTED_EDGE ( 'NONE', *, *, #15224, .T. ) ;
#5107=LINE ( 'NONE', #10581, #6098 ) ;
#5109=CARTESIAN_POINT ( 'NONE',  ( 25.81771031727288346, 199.3779494270211785, 17.85644994789938167 ) ) ;
#5111=DIRECTION ( 'NONE',  ( -1.000000000000000000, -0.000000000000000000, -0.000000000000000000 ) ) ;
#5114=ORIENTED_EDGE ( 'NONE', *, *, #2989, .F. ) ;
#5116=CARTESIAN_POINT ( 'NONE',  ( -77.93691419132714771, 142.0644190903623212, 14.67410160148079967 ) ) ;
#5117=CARTESIAN_POINT ( 'NONE',  ( 25.49999999999998579, 9.999999999999998224, 10.00000000000000178 ) ) ;
#5123=EDGE_CURVE ( 'NONE', #10007, #8974, #2403, .T. ) ;
#5128=EDGE_CURVE ( 'NONE', #9979, #11801, #4670, .T. ) ;
#5130=ORIENTED_EDGE ( 'NONE', *, *, #2938, .F. ) ;
#5131=VERTEX_POINT ( 'NONE', #8852 ) ;
#5133=ORIENTED_EDGE ( 'NONE', *, *, #7920, .F. ) ;
#5141=CARTESIAN_POINT ( 'NONE',  ( 32.87600950244731735, 192.5178712342568019, 25.54362227291153786 ) ) ;
#5148=CARTESIAN_POINT ( 'NONE',  ( -725.0000000000001137, 129.9999999999995453, 4.999999999999999112 ) ) ;
#5149=ORIENTED_EDGE ( 'NONE', *, *, #14530, .T. ) ;
#5151=DIRECTION ( 'NONE',  ( -1.000000000000000000, 0.000000000000000000, 0.000000000000000000 ) ) ;
#5154=CARTESIAN_POINT ( 'NONE',  ( 24.34257225596280350, 140.5456842492515932, 11.13195485280035513 ) ) ;
#5156=EDGE_LOOP ( 'NONE', ( #15530, #2469 ) ) ;
#5159=EDGE_CURVE ( 'NONE', #7694, #10746, #11450, .T. ) ;
#5162=DIRECTION ( 'NONE',  ( 1.000000000000000000, 0.000000000000000000, 0.000000000000000000 ) ) ;
#5176=CARTESIAN_POINT ( 'NONE',  ( -16.30611068361785954, 32.76923076923075939, 5.287877769756280877 ) ) ;
#5177=CARTESIAN_POINT ( 'NONE',  ( -13.77790586189935951, 31.39781009804136502, 13.10675149387370197 ) ) ;
#5179=CARTESIAN_POINT ( 'NONE',  ( 22.51491806150639974, 29.85019096660411364, 7.572044396946283840 ) ) ;
#5180=CARTESIAN_POINT ( 'NONE',  ( 39.99999999999998579, 4.000000000000000000, 33.00000000000000711 ) ) ;
#5181=VERTEX_POINT ( 'NONE', #11832 ) ;
#5183=CARTESIAN_POINT ( 'NONE',  ( 50.00000000000000000, 146.6227766016838245, 0.000000000000000000 ) ) ;
#5184=CARTESIAN_POINT ( 'NONE',  ( 8.750829511962136209, 133.4309389808502715, 14.69696305399116198 ) ) ;
#5188=DIRECTION ( 'NONE',  ( 0.000000000000000000, 0.000000000000000000, -1.000000000000000000 ) ) ;
#5195=DIRECTION ( 'NONE',  ( -1.000000000000000000, 0.000000000000000000, 0.000000000000000000 ) ) ;
#5203=UNCERTAINTY_MEASURE_WITH_UNIT (LENGTH_MEASURE( 1.000000000000000082E-05 ), #2996, 'distance_accuracy_value', 'NONE');
#5204=SURFACE_STYLE_USAGE ( .BOTH. , #14851 ) ;
#5206=EDGE_CURVE ( 'NONE', #6576, #10977, #13435, .T. ) ;
#5208=AXIS2_PLACEMENT_3D ( 'NONE', #1136, #12525, #1402 ) ;
#5209=FACE_OUTER_BOUND ( 'NONE', #14991, .T. ) ;
#5214=ORIENTED_EDGE ( 'NONE', *, *, #13567, .T. ) ;
#5215=DIRECTION ( 'NONE',  ( -0.000000000000000000, -0.000000000000000000, -1.000000000000000000 ) ) ;
#5216=CARTESIAN_POINT ( 'NONE',  ( -3.000000000000002665, 171.6227766016838245, 0.000000000000000000 ) ) ;
#5226=VECTOR ( 'NONE', #15146, 1000.000000000000000 ) ;
#5228=PLANE ( 'NONE',  #10865 ) ;
#5232=ORIENTED_EDGE ( 'NONE', *, *, #1257, .T. ) ;
#5236=FACE_OUTER_BOUND ( 'NONE', #1864, .T. ) ;
#5237=CARTESIAN_POINT ( 'NONE',  ( 15.12922779335904977, 126.1891464972476911, 7.145555214655046505 ) ) ;
#5239=CARTESIAN_POINT ( 'NONE',  ( 14.93242934743711814, 30.00000000000000000, 15.00000000000000000 ) ) ;
#5247=CARTESIAN_POINT ( 'NONE',  ( 34.06272495246724930, 149.5415222133261466, 24.52446659945426433 ) ) ;
#5249=EDGE_CURVE ( 'NONE', #12504, #5356, #17328, .T. ) ;
#5251=VERTEX_POINT ( 'NONE', #3882 ) ;
#5253=DIRECTION ( 'NONE',  ( -0.000000000000000000, -0.000000000000000000, -1.000000000000000000 ) ) ;
#5254=VECTOR ( 'NONE', #3543, 1000.000000000000000 ) ;
#5255=VERTEX_POINT ( 'NONE', #14677 ) ;
#5262=CARTESIAN_POINT ( 'NONE',  ( -15.77503540472913457, 32.61497647743762229, 7.787339510197840653 ) ) ;
#5263=VECTOR ( 'NONE', #15882, 1000.000000000000000 ) ;
#5266=CARTESIAN_POINT ( 'NONE',  ( 32.50000000000000000, 196.6227766016838245, 0.000000000000000000 ) ) ;
#5268=VERTEX_POINT ( 'NONE', #13352 ) ;
#5269=CARTESIAN_POINT ( 'NONE',  ( 27.99999999999998224, 9.999999999999998224, 10.00000000000000178 ) ) ;
#5276=CARTESIAN_POINT ( 'NONE',  ( 21.54624641763228254, 29.91220938647573391, 12.53033468027509478 ) ) ;
#5284=CARTESIAN_POINT ( 'NONE',  ( 15.00000000000000000, 143.0344144757318929, 16.50549856913627877 ) ) ;
#5287=EDGE_LOOP ( 'NONE', ( #7055, #14522, #9950, #15928 ) ) ;
#5289=VERTEX_POINT ( 'NONE', #9436 ) ;
#5293=VECTOR ( 'NONE', #15572, 1000.000000000000000 ) ;
#5294=EDGE_CURVE ( 'NONE', #11801, #1199, #2702, .T. ) ;
#5296=CIRCLE ( 'NONE', #3315, 5.000000000000004441 ) ;
#5299=DIRECTION ( 'NONE',  ( -0.000000000000000000, -0.000000000000000000, -1.000000000000000000 ) ) ;
#5301=B_SPLINE_CURVE_WITH_KNOTS ( 'NONE', 3,
 ( #10250, #16005, #17069, #7856 ),
 .UNSPECIFIED., .F., .F.,
 ( 4, 4 ),
 ( 0.000000000000000000, 0.001170341053039947524 ),
 .UNSPECIFIED. ) ;
#5305=CARTESIAN_POINT ( 'NONE',  ( 0.000000000000000000, 18.00000000000000355, 25.00000000000000000 ) ) ;
#5309=VECTOR ( 'NONE', #17172, 1000.000000000000000 ) ;
#5311=ORIENTED_EDGE ( 'NONE', *, *, #6514, .T. ) ;
#5312=FACE_OUTER_BOUND ( 'NONE', #10473, .T. ) ;
#5317=DIRECTION ( 'NONE',  ( 1.000000000000000000, 0.000000000000000000, 0.000000000000000000 ) ) ;
#5318=ADVANCED_FACE ( 'NONE', ( #405 ), #7059, .F. ) ;
#5321=CARTESIAN_POINT ( 'NONE',  ( -91.33974596215564645, 171.6227766016838245, 0.000000000000000000 ) ) ;
#5322=FACE_OUTER_BOUND ( 'NONE', #1370, .T. ) ;
#5323=CIRCLE ( 'NONE', #7012, 2.500000000000002220 ) ;
#5326=CARTESIAN_POINT ( 'NONE',  ( 32.50000000000000711, 146.6227766016838245, 0.000000000000000000 ) ) ;
#5328=CARTESIAN_POINT ( 'NONE',  ( -25.00000000000002132, 130.0000000000000000, 15.00000000000000000 ) ) ;
#5329=ORIENTED_EDGE ( 'NONE', *, *, #4352, .F. ) ;
#5330=LINE ( 'NONE', #7979, #8466 ) ;
#5333=ORIENTED_EDGE ( 'NONE', *, *, #9719, .T. ) ;
#5334=CARTESIAN_POINT ( 'NONE',  ( -10.59078875499043981, 20.00000000000000000, 13.69642986623834702 ) ) ;
#5336=EDGE_LOOP ( 'NONE', ( #5648, #9144, #4783, #8908, #1418, #4694 ) ) ;
#5340=CARTESIAN_POINT ( 'NONE',  ( -34.99999999999999289, 122.0000000000000284, 4.999999999999999112 ) ) ;
#5344=ORIENTED_EDGE ( 'NONE', *, *, #13274, .T. ) ;
#5346=CARTESIAN_POINT ( 'NONE',  ( 34.89689726072227671, 147.6679082027615948, 22.70058015389365735 ) ) ;
#5348=VECTOR ( 'NONE', #4483, 1000.000000000000000 ) ;
#5349=ORIENTED_EDGE ( 'NONE', *, *, #3481, .F. ) ;
#5356=VERTEX_POINT ( 'NONE', #14842 ) ;
#5358=CARTESIAN_POINT ( 'NONE',  ( 7.559396570614633326, 133.9010074147453508, 14.92908841323498770 ) ) ;
#5359=CIRCLE ( 'NONE', #11011, 30.00000000000000000 ) ;
#5363=CARTESIAN_POINT ( 'NONE',  ( -725.0000000000000000, 30.00000000000000000, 15.00000000000000000 ) ) ;
#5368=CARTESIAN_POINT ( 'NONE',  ( -77.93529739263047418, 151.1803749979462737, 25.90597399044991889 ) ) ;
#5370=DIRECTION ( 'NONE',  ( -1.000000000000000000, -6.938893903907228378E-16, 0.000000000000000000 ) ) ;
#5371=CARTESIAN_POINT ( 'NONE',  ( -15.00000000000001421, 130.0000000000000000, 13.00000000000000000 ) ) ;
#5375=DIRECTION ( 'NONE',  ( 1.156482317317868274E-16, -1.000000000000000000, 0.000000000000000000 ) ) ;
#5377=VECTOR ( 'NONE', #12648, 1000.000000000000000 ) ;
#5380=DIRECTION ( 'NONE',  ( -0.000000000000000000, -0.000000000000000000, -1.000000000000000000 ) ) ;
#5381=VERTEX_POINT ( 'NONE', #9792 ) ;
#5386=ADVANCED_FACE ( 'NONE', ( #14934 ), #16716, .T. ) ;
#5391=VECTOR ( 'NONE', #676, 1000.000000000000000 ) ;
#5392=CARTESIAN_POINT ( 'NONE',  ( -26.89314795393037016, 19.99999999999999289, 11.55702759004480207 ) ) ;
#5393=EDGE_LOOP ( 'NONE', ( #17208, #9508, #4771, #9871, #5684, #8280, #3828, #13692, #589, #11880, #15351, #5311, #9119, #2947, #981, #12948, #13355, #5817, #13278, #11381, #8133, #11283, #8888, #2327, #9325, #9006, #9539, #8043, #11084, #9300, #14532, #6854, #6817, #2408, #7392, #2230, #7306, #2576, #7520, #15188, #9135, #16467, #12753, #10723, #16786, #14080, #3945, #8722, #4952, #1267, #9956, #7867, #5950, #14714, #9375 ) ) ;
#5395=DIRECTION ( 'NONE',  ( -1.000000000000000000, 0.000000000000000000, 0.000000000000000000 ) ) ;
#5397=FILL_AREA_STYLE ('',( #7763 ) ) ;
#5398=ORIENTED_EDGE ( 'NONE', *, *, #3658, .F. ) ;
#5401=FACE_BOUND ( 'NONE', #7848, .T. ) ;
#5404=VERTEX_POINT ( 'NONE', #5907 ) ;
#5405=DIRECTION ( 'NONE',  ( 1.000000000000000000, 0.000000000000000000, 0.000000000000000000 ) ) ;
#5409=DIRECTION ( 'NONE',  ( -0.000000000000000000, -0.000000000000000000, -1.000000000000000000 ) ) ;
#5417=VERTEX_POINT ( 'NONE', #7227 ) ;
#5421=CARTESIAN_POINT ( 'NONE',  ( -48.00000000000000000, 171.6227766016838245, 0.000000000000000000 ) ) ;
#5422=ORIENTED_EDGE ( 'NONE', *, *, #10511, .T. ) ;
#5424=CARTESIAN_POINT ( 'NONE',  ( -10.16681828783789143, 30.62365918355438055, 14.67566226953583985 ) ) ;
#5425=CARTESIAN_POINT ( 'NONE',  ( 22.72753210816364700, 141.1551838527312555, 12.68377836492884470 ) ) ;
#5426=AXIS2_PLACEMENT_3D ( 'NONE', #1787, #2934, #7102 ) ;
#5427=VERTEX_POINT ( 'NONE', #501 ) ;
#5428=CARTESIAN_POINT ( 'NONE',  ( 16.23725950538873164, 20.00000000000000000, 24.99999999984155252 ) ) ;
#5436=ORIENTED_EDGE ( 'NONE', *, *, #7524, .T. ) ;
#5443=CARTESIAN_POINT ( 'NONE',  ( -68.00000000000000000, 143.0439382767972347, 16.49999999999984368 ) ) ;
#5445=EDGE_CURVE ( 'NONE', #8820, #12504, #12807, .T. ) ;
#5446=VERTEX_POINT ( 'NONE', #15365 ) ;
#5448=ADVANCED_FACE ( 'NONE', ( #15626 ), #4583, .F. ) ;
#5450=EDGE_CURVE ( 'NONE', #11548, #2095, #8428, .T. ) ;
#5451=FACE_OUTER_BOUND ( 'NONE', #14740, .T. ) ;
#5453=CARTESIAN_POINT ( 'NONE',  ( -83.42148544384103559, 150.2853719096988812, 25.17531865327014629 ) ) ;
#5456=CARTESIAN_POINT ( 'NONE',  ( 11.07991637643875116, 132.1496266960828336, 13.91448104906911709 ) ) ;
#5459=DIRECTION ( 'NONE',  ( -0.000000000000000000, -0.000000000000000000, -1.000000000000000000 ) ) ;
#5461=CARTESIAN_POINT ( 'NONE',  ( -90.80384757729339640, 138.6227766016838245, 0.000000000000000000 ) ) ;
#5463=DIRECTION ( 'NONE',  ( 1.000000000000000000, 0.000000000000000000, 0.000000000000000000 ) ) ;
#5467=CARTESIAN_POINT ( 'NONE',  ( -82.50000000000002842, 146.6227766016838245, 0.000000000000000000 ) ) ;
#5468=DIRECTION ( 'NONE',  ( -1.000000000000000000, -0.000000000000000000, -0.000000000000000000 ) ) ;
#5472=FACE_OUTER_BOUND ( 'NONE', #10269, .T. ) ;
#5473=CARTESIAN_POINT ( 'NONE',  ( 49.99999999999998579, 175.6227766016838245, 8.071800142134975431 ) ) ;
#5474=EDGE_CURVE ( 'NONE', #7978, #14499, #14574, .T. ) ;
#5478=ORIENTED_EDGE ( 'NONE', *, *, #16537, .F. ) ;
#5481=VERTEX_POINT ( 'NONE', #6321 ) ;
#5482=CARTESIAN_POINT ( 'NONE',  ( 0.000000000000000000, 0.000000000000000000, 0.000000000000000000 ) ) ;
#5483=CARTESIAN_POINT ( 'NONE',  ( -25.00000000000002132, 120.0000000000000284, 5.000000000000023093 ) ) ;
#5486=CARTESIAN_POINT ( 'NONE',  ( 24.99999999999999645, 196.1091490972146403, 22.13677318565946095 ) ) ;
#5490=DIRECTION ( 'NONE',  ( 1.000000000000000000, 0.000000000000000000, -0.000000000000000000 ) ) ;
#5491=CARTESIAN_POINT ( 'NONE',  ( 49.99999999999998579, 179.6227766016838245, 10.00000337241049309 ) ) ;
#5492=DIRECTION ( 'NONE',  ( 0.000000000000000000, 0.000000000000000000, 1.000000000000000000 ) ) ;
#5494=ORIENTED_EDGE ( 'NONE', *, *, #14985, .T. ) ;
#5497=EDGE_CURVE ( 'NONE', #1301, #3629, #6525, .T. ) ;
#5499=EDGE_LOOP ( 'NONE', ( #13309, #15018, #1023, #14183, #15285, #17226, #15514, #143, #12322, #5349 ) ) ;
#5503=CARTESIAN_POINT ( 'NONE',  ( -13.98869899561406882, 20.00000000000231637, 10.23150106588177621 ) ) ;
#5508=ORIENTED_EDGE ( 'NONE', *, *, #7160, .T. ) ;
#5516=CARTESIAN_POINT ( 'NONE',  ( 25.00000000000001421, 147.1386660375792417, 22.13939837391653853 ) ) ;
#5526=CARTESIAN_POINT ( 'NONE',  ( 9.647168043681871197, 132.9898913927504225, 14.44632387683999575 ) ) ;
#5534=AXIS2_PLACEMENT_3D ( 'NONE', #15903, #15815, #13156 ) ;
#5535=EDGE_CURVE ( 'NONE', #13709, #5614, #2955, .T. ) ;
#5537=ORIENTED_EDGE ( 'NONE', *, *, #9179, .T. ) ;
#5540=LINE ( 'NONE', #9604, #1271 ) ;
#5541=CYLINDRICAL_SURFACE ( 'NONE', #4780, 12.00000000000000000 ) ;
#5546=AXIS2_PLACEMENT_3D ( 'NONE', #12520, #6140, #16599 ) ;
#5547=CARTESIAN_POINT ( 'NONE',  ( -90.80384757729339640, 204.6227766016838245, 0.000000000000000000 ) ) ;
#5557=VECTOR ( 'NONE', #16924, 1000.000000000000000 ) ;
#5561=CIRCLE ( 'NONE', #16872, 2.499999999999998668 ) ;
#5564=AXIS2_PLACEMENT_3D ( 'NONE', #12929, #5947, #15660 ) ;
#5571=PRESENTATION_STYLE_ASSIGNMENT (( #9899 ) ) ;
#5574=DIRECTION ( 'NONE',  ( -1.000000000000000000, -0.000000000000000000, -0.000000000000000000 ) ) ;
#5576=CARTESIAN_POINT ( 'NONE',  ( 30.98806968877808998, 191.7175861903016596, 26.17636150746909607 ) ) ;
#5579=DIRECTION ( 'NONE',  ( 1.000000000000000000, 0.000000000000000000, -0.000000000000000000 ) ) ;
#5583=DIRECTION ( 'NONE',  ( 0.000000000000000000, -0.8660254037844413721, 0.4999999999999953371 ) ) ;
#5585=ORIENTED_EDGE ( 'NONE', *, *, #4681, .F. ) ;
#5587=VECTOR ( 'NONE', #7566, 1000.000000000000000 ) ;
#5590=CARTESIAN_POINT ( 'NONE',  ( -15.30535435590778448, 19.99999999999999645, 5.925683940270866756 ) ) ;
#5591=CARTESIAN_POINT ( 'NONE',  ( -25.49999999999998579, 10.00000000000000000, 0.000000000000000000 ) ) ;
#5592=ORIENTED_EDGE ( 'NONE', *, *, #9213, .T. ) ;
#5596=EDGE_CURVE ( 'NONE', #6523, #6919, #10314, .T. ) ;
#5597=ADVANCED_FACE ( 'NONE', ( #10921 ), #1282, .F. ) ;
#5598=AXIS2_PLACEMENT_3D ( 'NONE', #2881, #5370, #16176 ) ;
#5600=VECTOR ( 'NONE', #5746, 1000.000000000000000 ) ;
#5614=VERTEX_POINT ( 'NONE', #16249 ) ;
#5618=CARTESIAN_POINT ( 'NONE',  ( 27.48361012698968864, 136.6227766016838245, 4.651049393634109604E-13 ) ) ;
#5623=CARTESIAN_POINT ( 'NONE',  ( -70.00000000000000000, 154.3022685259950038, 9.999999999999900524 ) ) ;
#5624=CYLINDRICAL_SURFACE ( 'NONE', #3943, 2.500000000000000444 ) ;
#5625=DIRECTION ( 'NONE',  ( -0.000000000000000000, -0.000000000000000000, -1.000000000000000000 ) ) ;
#5626=CARTESIAN_POINT ( 'NONE',  ( 18.50138388889793362, 17.99999999999999289, 12.24385303908842637 ) ) ;
#5627=CIRCLE ( 'NONE', #545, 2.499999999999998668 ) ;
#5628=CIRCLE ( 'NONE', #1381, 2.500000000000000444 ) ;
#5629=ORIENTED_EDGE ( 'NONE', *, *, #81, .T. ) ;
#5632=CYLINDRICAL_SURFACE ( 'NONE', #11272, 747.9999999999998863 ) ;
#5634=DIRECTION ( 'NONE',  ( -6.938893903907228378E-16, 1.000000000000000000, 0.000000000000000000 ) ) ;
#5636=VECTOR ( 'NONE', #429, 1000.000000000000000 ) ;
#5641=CARTESIAN_POINT ( 'NONE',  ( 196.0000000000000000, 175.6227766016838245, 3.071800142134975431 ) ) ;
#5643=ORIENTED_EDGE ( 'NONE', *, *, #9290, .F. ) ;
#5647=ADVANCED_FACE ( 'NONE', ( #12345 ), #6864, .T. ) ;
#5648=ORIENTED_EDGE ( 'NONE', *, *, #4820, .T. ) ;
#5651=DIRECTION ( 'NONE',  ( -1.000000000000000000, 0.000000000000000000, 0.000000000000000000 ) ) ;
#5652=PLANE ( 'NONE',  #2000 ) ;
#5655=VERTEX_POINT ( 'NONE', #5623 ) ;
#5657=PLANE ( 'NONE',  #5849 ) ;
#5658=CARTESIAN_POINT ( 'NONE',  ( -75.00000000000000000, 196.6227766016838245, 35.00200000000000244 ) ) ;
#5664=AXIS2_PLACEMENT_3D ( 'NONE', #7589, #9978, #875 ) ;
#5666=ADVANCED_FACE ( 'NONE', ( #2792 ), #11742, .F. ) ;
#5672=CARTESIAN_POINT ( 'NONE',  ( 19.16569565073602277, 29.91542719746881929, 11.79421528189872070 ) ) ;
#5678=VECTOR ( 'NONE', #8641, 1000.000000000000000 ) ;
#5679=DIRECTION ( 'NONE',  ( -1.000000000000000000, 0.000000000000000000, 0.000000000000000000 ) ) ;
#5684=ORIENTED_EDGE ( 'NONE', *, *, #11201, .F. ) ;
#5687=CARTESIAN_POINT ( 'NONE',  ( -20.85266279178582138, 18.00000000000000000, 20.15433268689461954 ) ) ;
#5690=PLANE ( 'NONE',  #12208 ) ;
#5696=DIRECTION ( 'NONE',  ( -0.000000000000000000, -0.000000000000000000, -1.000000000000000000 ) ) ;
#5697=FACE_BOUND ( 'NONE', #15771, .T. ) ;
#5699=EDGE_CURVE ( 'NONE', #8489, #12692, #6958, .T. ) ;
#5700=VERTEX_POINT ( 'NONE', #15521 ) ;
#5701=ADVANCED_FACE ( 'NONE', ( #14119 ), #16775, .F. ) ;
#5707=CARTESIAN_POINT ( 'NONE',  ( 17.42040306417330342, 125.8667821340875577, 6.358709916038607801 ) ) ;
#5714=CARTESIAN_POINT ( 'NONE',  ( 17.77234289100806564, 17.99999999999999289, 12.54415977683811256 ) ) ;
#5715=ORIENTED_EDGE ( 'NONE', *, *, #8285, .F. ) ;
#5716=FACE_OUTER_BOUND ( 'NONE', #9232, .T. ) ;
#5719=CARTESIAN_POINT ( 'NONE',  ( 225.0000000000000000, 89.99999999999997158, 15.00000000000000000 ) ) ;
#5724=DIRECTION ( 'NONE',  ( 0.000000000000000000, -1.000000000000000000, 0.000000000000000000 ) ) ;
#5726=CARTESIAN_POINT ( 'NONE',  ( 196.0000000000000000, 167.6227766016838530, 5.571800142134975431 ) ) ;
#5730=ADVANCED_BREP_SHAPE_REPRESENTATION ( '', ( #11216, #3583 ), #11517 ) ;
#5734=CARTESIAN_POINT ( 'NONE',  ( 35.00000000000000711, 146.6227766016838245, 21.54065922853802562 ) ) ;
#5736=LINE ( 'NONE', #4323, #5956 ) ;
#5742=FACE_BOUND ( 'NONE', #10427, .T. ) ;
#5746=DIRECTION ( 'NONE',  ( 1.000000000000000000, 0.000000000000000000, 0.000000000000000000 ) ) ;
#5751=CARTESIAN_POINT ( 'NONE',  ( -75.10997073956447423, 197.8146641845672491, 20.09570409464925334 ) ) ;
#5756=CARTESIAN_POINT ( 'NONE',  ( 22.99999999999997868, 9.999999999999998224, 28.00000000000001066 ) ) ;
#5757=DIRECTION ( 'NONE',  ( -1.000000000000000000, -0.000000000000000000, -0.000000000000000000 ) ) ;
#5761=ADVANCED_FACE ( 'NONE', ( #7291 ), #10114, .F. ) ;
#5762=DIRECTION ( 'NONE',  ( -1.000000000000000000, -0.000000000000000000, -0.000000000000000000 ) ) ;
#5763=ORIENTED_EDGE ( 'NONE', *, *, #9719, .F. ) ;
#5769=DIRECTION ( 'NONE',  ( 1.000000000000000000, 0.000000000000000000, 0.000000000000000000 ) ) ;
#5771=LINE ( 'NONE', #11429, #5226 ) ;
#5773=CARTESIAN_POINT ( 'NONE',  ( -100.0000000000000000, 171.6227766016838245, 0.000000000000000000 ) ) ;
#5775=CARTESIAN_POINT ( 'NONE',  ( -85.00000000000002842, 146.6227766016838245, 21.54065922853802562 ) ) ;
#5777=ORIENTED_EDGE ( 'NONE', *, *, #8575, .T. ) ;
#5781=CARTESIAN_POINT ( 'NONE',  ( -5.000000000000000888, 171.6227766016838245, 0.000000000000000000 ) ) ;
#5787=FACE_OUTER_BOUND ( 'NONE', #2224, .T. ) ;
#5789=CARTESIAN_POINT ( 'NONE',  ( 16.74904763372935790, 29.96341334642810139, 12.79227977592015897 ) ) ;
#5794=AXIS2_PLACEMENT_3D ( 'NONE', #17182, #15593, #5055 ) ;
#5797=DIRECTION ( 'NONE',  ( 1.000000000000000000, 0.000000000000000000, 0.000000000000000000 ) ) ;
#5799=ORIENTED_EDGE ( 'NONE', *, *, #5535, .F. ) ;
#5801=CARTESIAN_POINT ( 'NONE',  ( 196.0000000000000000, 159.6227766016838814, 8.071800142134975431 ) ) ;
#5806=LINE ( 'NONE', #8818, #5678 ) ;
#5808=AXIS2_PLACEMENT_3D ( 'NONE', #13914, #6022, #16563 ) ;
#5812=ADVANCED_FACE ( 'NONE', ( #7123 ), #10021, .F. ) ;
#5814=CARTESIAN_POINT ( 'NONE',  ( -147.9615242270661213, 171.6227766016838245, 0.000000000000000000 ) ) ;
#5815=EDGE_CURVE ( 'NONE', #5255, #3947, #7455, .T. ) ;
#5817=ORIENTED_EDGE ( 'NONE', *, *, #11933, .T. ) ;
#5818=DIRECTION ( 'NONE',  ( -0.8571673013836867971, 0.000000000000000000, -0.5150380737757237481 ) ) ;
#5820=FACE_OUTER_BOUND ( 'NONE', #8272, .T. ) ;
#5823=AXIS2_PLACEMENT_3D ( 'NONE', #231, #5634, #16520 ) ;
#5825=VERTEX_POINT ( 'NONE', #15604 ) ;
#5830=EDGE_CURVE ( 'NONE', #3629, #2336, #12903, .T. ) ;
#5835=DIRECTION ( 'NONE',  ( -1.000000000000000000, 0.000000000000000000, 0.000000000000000000 ) ) ;
#5838=CARTESIAN_POINT ( 'NONE',  ( -77.05368524155726107, 200.6745000914694401, 15.65774685523815890 ) ) ;
#5847=ORIENTED_EDGE ( 'NONE', *, *, #15621, .F. ) ;
#5848=CARTESIAN_POINT ( 'NONE',  ( -14.77653433949313744, 31.60550367499664759, 12.35354907637233701 ) ) ;
#5849=AXIS2_PLACEMENT_3D ( 'NONE', #1414, #4420, #161 ) ;
#5862=ADVANCED_FACE ( 'NONE', ( #8867 ), #3744, .F. ) ;
#5865=ORIENTED_EDGE ( 'NONE', *, *, #917, .F. ) ;
#5866=CARTESIAN_POINT ( 'NONE',  ( 49.99999999999998579, 151.6227766016839098, 5.571800142134973655 ) ) ;
#5874=CARTESIAN_POINT ( 'NONE',  ( 15.95013150516294154, 137.1612117474554111, 8.111885438162648398 ) ) ;
#5875=CIRCLE ( 'NONE', #10100, 2.499999999999998668 ) ;
#5880=CARTESIAN_POINT ( 'NONE',  ( -78.44971993548843159, 191.8535701216948155, 26.07159546787934445 ) ) ;
#5881=CARTESIAN_POINT ( 'NONE',  ( 196.0000000000000000, 167.6227766016838530, 8.071800142134975431 ) ) ;
#5882=CARTESIAN_POINT ( 'NONE',  ( 19.20424459521615290, 18.00000000000228439, 11.86908137778077688 ) ) ;
#5884=DIRECTION ( 'NONE',  ( -1.000000000000000000, 0.000000000000000000, 0.000000000000000000 ) ) ;
#5888=AXIS2_PLACEMENT_3D ( 'NONE', #14919, #9344, #8009 ) ;
#5891=DIRECTION ( 'NONE',  ( 0.000000000000000000, 0.000000000000000000, -1.000000000000000000 ) ) ;
#5893=DIRECTION ( 'NONE',  ( 0.000000000000000000, 0.000000000000000000, 1.000000000000000000 ) ) ;
#5896=VERTEX_POINT ( 'NONE', #14633 ) ;
#5899=EDGE_CURVE ( 'NONE', #2134, #13670, #1870, .T. ) ;
#5904=AXIS2_PLACEMENT_3D ( 'NONE', #5148, #10536, #2490 ) ;
#5905=DIRECTION ( 'NONE',  ( 0.000000000000000000, -1.000000000000000000, 6.123233995736762338E-17 ) ) ;
#5907=CARTESIAN_POINT ( 'NONE',  ( -100.0000000000000000, 199.3133755249253056, 1.695560166891042033E-15 ) ) ;
#5911=CARTESIAN_POINT ( 'NONE',  ( 29.06781294723401388, 141.7051482704754335, 13.92628470286629927 ) ) ;
#5918=VECTOR ( 'NONE', #10283, 1000.000000000000000 ) ;
#5921=EDGE_CURVE ( 'NONE', #5131, #8580, #13746, .T. ) ;
#5922=EDGE_CURVE ( 'NONE', #12616, #16088, #10084, .T. ) ;
#5923=EDGE_LOOP ( 'NONE', ( #14385, #5344, #781, #13180 ) ) ;
#5925=ORIENTED_EDGE ( 'NONE', *, *, #17461, .F. ) ;
#5927=CARTESIAN_POINT ( 'NONE',  ( 23.67803828928656884, 138.9414820825090544, 12.55787835418278675 ) ) ;
#5934=FACE_OUTER_BOUND ( 'NONE', #10749, .T. ) ;
#5935=ORIENTED_EDGE ( 'NONE', *, *, #1819, .F. ) ;
#5936=DIRECTION ( 'NONE',  ( -1.000000000000000000, 0.000000000000000000, 0.000000000000000000 ) ) ;
#5937=CARTESIAN_POINT ( 'NONE',  ( 22.93524650466160963, 29.84210526315773748, 4.999999999999999112 ) ) ;
#5938=CARTESIAN_POINT ( 'NONE',  ( -75.00000000000000000, 196.6227766016838245, 21.54065922853802206 ) ) ;
#5944=CIRCLE ( 'NONE', #14417, 2.499999999999998668 ) ;
#5945=CARTESIAN_POINT ( 'NONE',  ( 35.00000000000000000, 196.6227766016838245, 21.54065922853802206 ) ) ;
#5947=DIRECTION ( 'NONE',  ( -0.000000000000000000, -0.000000000000000000, -1.000000000000000000 ) ) ;
#5949=DIRECTION ( 'NONE',  ( -0.000000000000000000, -0.000000000000000000, -1.000000000000000000 ) ) ;
#5950=ORIENTED_EDGE ( 'NONE', *, *, #6173, .F. ) ;
#5953=CARTESIAN_POINT ( 'NONE',  ( -100.0000000000000000, 171.6227766016838245, 0.000000000000000000 ) ) ;
#5954=DIRECTION ( 'NONE',  ( -0.000000000000000000, -0.000000000000000000, -1.000000000000000000 ) ) ;
#5956=VECTOR ( 'NONE', #1754, 1000.000000000000000 ) ;
#5959=VECTOR ( 'NONE', #5905, 1000.000000000000000 ) ;
#5965=DIRECTION ( 'NONE',  ( 0.000000000000000000, 2.775557561562891351E-15, 1.000000000000000000 ) ) ;
#5967=ORIENTED_EDGE ( 'NONE', *, *, #11776, .F. ) ;
#5969=CIRCLE ( 'NONE', #9912, 249.9999999999999716 ) ;
#5971=CARTESIAN_POINT ( 'NONE',  ( 16.24385689529520604, 136.8350826111700655, 4.682368943704262598 ) ) ;
#5977=CARTESIAN_POINT ( 'NONE',  ( 17.00458606767794834, 29.95830270928036398, 12.72829919683579902 ) ) ;
#5978=DIRECTION ( 'NONE',  ( 0.000000000000000000, 0.000000000000000000, 1.000000000000000000 ) ) ;
#5979=ORIENTED_EDGE ( 'NONE', *, *, #1438, .T. ) ;
#5989=CARTESIAN_POINT ( 'NONE',  ( 10.09659264799822331, 132.0789811519323962, 12.16719622200489681 ) ) ;
#6000=CARTESIAN_POINT ( 'NONE',  ( 31.71694765202421351, 141.9230918234059402, 14.38591257614910823 ) ) ;
#6004=CARTESIAN_POINT ( 'NONE',  ( -22.99999999999998224, 10.00000000000000000, 0.000000000000000000 ) ) ;
#6005=DIRECTION ( 'NONE',  ( -1.000000000000000000, 0.000000000000000000, 0.000000000000000000 ) ) ;
#6013=EDGE_LOOP ( 'NONE', ( #16866, #9174, #3361, #11111 ) ) ;
#6014=FACE_OUTER_BOUND ( 'NONE', #10183, .T. ) ;
#6018=CARTESIAN_POINT ( 'NONE',  ( -75.82181986242348160, 199.3841150854655666, 17.84683500849085647 ) ) ;
#6020=ORIENTED_EDGE ( 'NONE', *, *, #2781, .T. ) ;
#6022=DIRECTION ( 'NONE',  ( -1.000000000000000000, -0.000000000000000000, -0.000000000000000000 ) ) ;
#6023=CARTESIAN_POINT ( 'NONE',  ( 49.99999999999998579, 159.6227766016838814, 3.071800142134975431 ) ) ;
#6029=CARTESIAN_POINT ( 'NONE',  ( -14.99999999999998579, 90.00000000000000000, 4.999999999999999112 ) ) ;
#6032=CARTESIAN_POINT ( 'NONE',  ( -16.41264213764166513, 18.00000000000000000, 23.02790928165778794 ) ) ;
#6036=ADVANCED_FACE ( 'NONE', ( #16230 ), #1356, .F. ) ;
#6038=DIRECTION ( 'NONE',  ( -1.000000000000000000, 0.000000000000000000, 0.000000000000000000 ) ) ;
#6039=EDGE_LOOP ( 'NONE', ( #5149, #6252, #16658, #4787 ) ) ;
#6042=CARTESIAN_POINT ( 'NONE',  ( 22.99999999999997868, 9.999999999999998224, 35.00200000000000244 ) ) ;
#6046=CARTESIAN_POINT ( 'NONE',  ( 24.41196201396447663, 20.00000000000113687, 8.570466955472159754 ) ) ;
#6047=CARTESIAN_POINT ( 'NONE',  ( 27.44407568426053246, 136.8394969516870958, 3.888888888888893725 ) ) ;
#6051=CARTESIAN_POINT ( 'NONE',  ( 17.00000000000000000, 171.6227766016838245, 0.000000000000000000 ) ) ;
#6052=CARTESIAN_POINT ( 'NONE',  ( -80.77514562707608547, 191.6792914357319262, 26.20566807848922863 ) ) ;
#6058=CARTESIAN_POINT ( 'NONE',  ( 39.99999999999998579, 0.000000000000000000, 33.00000000000000711 ) ) ;
#6059=ORIENTED_EDGE ( 'NONE', *, *, #15800, .F. ) ;
#6061=CARTESIAN_POINT ( 'NONE',  ( -22.93725393319379791, 120.0000000000000284, 6.000000000000001776 ) ) ;
#6068=DIRECTION ( 'NONE',  ( 0.000000000000000000, 0.000000000000000000, 1.000000000000000000 ) ) ;
#6074=CARTESIAN_POINT ( 'NONE',  ( -25.49999999999998579, 10.00000000000000000, 10.00000000000000178 ) ) ;
#6076=CIRCLE ( 'NONE', #2390, 20.00000000000000355 ) ;
#6077=ORIENTED_EDGE ( 'NONE', *, *, #8189, .F. ) ;
#6078=CARTESIAN_POINT ( 'NONE',  ( 35.00000000000000711, 146.3163998792643667, 21.18507967179266416 ) ) ;
#6086=VECTOR ( 'NONE', #17251, 1000.000000000000000 ) ;
#6088=DIRECTION ( 'NONE',  ( 0.000000000000000000, 1.000000000000000000, 0.000000000000000000 ) ) ;
#6089=VECTOR ( 'NONE', #10231, 1000.000000000000000 ) ;
#6091=CARTESIAN_POINT ( 'NONE',  ( 19.49215236471922807, 140.4173771131980857, 15.85404464849102268 ) ) ;
#6096=VERTEX_POINT ( 'NONE', #5340 ) ;
#6098=VECTOR ( 'NONE', #9428, 1000.000000000000000 ) ;
#6099=CARTESIAN_POINT ( 'NONE',  ( -75.53359938325087342, 198.8884873102157940, 18.59522663992144231 ) ) ;
#6103=ORIENTED_EDGE ( 'NONE', *, *, #16073, .T. ) ;
#6106=ORIENTED_EDGE ( 'NONE', *, *, #11641, .F. ) ;
#6107=DIRECTION ( 'NONE',  ( 0.000000000000000000, 0.000000000000000000, -1.000000000000000000 ) ) ;
#6109=DIRECTION ( 'NONE',  ( -1.000000000000000000, -0.000000000000000000, -0.000000000000000000 ) ) ;
#6110=AXIS2_PLACEMENT_3D ( 'NONE', #1638, #9418, #1377 ) ;
#6112=EDGE_CURVE ( 'NONE', #5181, #10830, #10736, .T. ) ;
#6118=CARTESIAN_POINT ( 'NONE',  ( -16.30611068361414695, 32.76923076921517008, 5.528684565802741702 ) ) ;
#6120=CIRCLE ( 'NONE', #758, 35.00000000000000000 ) ;
#6128=VECTOR ( 'NONE', #10343, 1000.000000000000000 ) ;
#6131=CARTESIAN_POINT ( 'NONE',  ( 28.15871609335591685, 19.99999999999999289, 20.05978710182010971 ) ) ;
#6134=CARTESIAN_POINT ( 'NONE',  ( 23.18512258076559007, 19.99999999999999645, 23.22991426836919260 ) ) ;
#6136=CARTESIAN_POINT ( 'NONE',  ( 49.99999999999998579, 175.6227766016838530, 19.42820660268601074 ) ) ;
#6137=ORIENTED_EDGE ( 'NONE', *, *, #5699, .T. ) ;
#6140=DIRECTION ( 'NONE',  ( 0.000000000000000000, -0.000000000000000000, -1.000000000000000000 ) ) ;
#6143=CARTESIAN_POINT ( 'NONE',  ( 196.0000000000000000, 167.6227766016838814, 19.42820660268601074 ) ) ;
#6147=CARTESIAN_POINT ( 'NONE',  ( -77.50000000000002842, 146.6227766016838245, 10.00000000000000178 ) ) ;
#6151=VECTOR ( 'NONE', #1144, 1000.000000000000000 ) ;
#6155=ORIENTED_EDGE ( 'NONE', *, *, #4526, .F. ) ;
#6156=VECTOR ( 'NONE', #5085, 1000.000000000000000 ) ;
#6157=ORIENTED_EDGE ( 'NONE', *, *, #9081, .F. ) ;
#6158=FACE_OUTER_BOUND ( 'NONE', #2536, .T. ) ;
#6159=EDGE_CURVE ( 'NONE', #14798, #16088, #1520, .T. ) ;
#6163=CARTESIAN_POINT ( 'NONE',  ( 6.134011831684049731, 134.2062027339443944, 13.00000000000000000 ) ) ;
#6164=CARTESIAN_POINT ( 'NONE',  ( -100.0000000000000000, 142.8100939375178200, 16.63501009223129756 ) ) ;
#6165=AXIS2_PLACEMENT_3D ( 'NONE', #11721, #5008, #17131 ) ;
#6166=CIRCLE ( 'NONE', #3055, 2.500000000000002220 ) ;
#6167=ORIENTED_EDGE ( 'NONE', *, *, #572, .F. ) ;
#6168=CARTESIAN_POINT ( 'NONE',  ( 25.63134405897505985, 139.9845197017440057, 9.403501633128708903 ) ) ;
#6169=DIRECTION ( 'NONE',  ( 1.000000000000000000, 0.000000000000000000, 0.000000000000000000 ) ) ;
#6173=EDGE_CURVE ( 'NONE', #6571, #4289, #12319, .T. ) ;
#6174=DIRECTION ( 'NONE',  ( -1.000000000000000000, -0.000000000000000000, -0.000000000000000000 ) ) ;
#6175=VECTOR ( 'NONE', #13034, 1000.000000000000000 ) ;
#6183=EDGE_LOOP ( 'NONE', ( #17030, #16710, #7087, #1508 ) ) ;
#6188=DIRECTION ( 'NONE',  ( -0.000000000000000000, 1.000000000000000000, 0.000000000000000000 ) ) ;
#6190=ORIENTED_EDGE ( 'NONE', *, *, #13391, .F. ) ;
#6194=CARTESIAN_POINT ( 'NONE',  ( -30.49999999999998224, 10.00000000000000000, 10.00000000000000178 ) ) ;
#6201=CIRCLE ( 'NONE', #12717, 2.500000000000002220 ) ;
#6204=AXIS2_PLACEMENT_3D ( 'NONE', #6575, #17368, #2406 ) ;
#6206=CARTESIAN_POINT ( 'NONE',  ( 30.00000000000000355, 196.6227766016838245, 0.000000000000000000 ) ) ;
#6208=CARTESIAN_POINT ( 'NONE',  ( -14.07899634757819385, 32.11373924370096233, 10.33209047619764753 ) ) ;
#6212=DIRECTION ( 'NONE',  ( -1.000000000000000000, -0.000000000000000000, -0.000000000000000000 ) ) ;
#6215=ORIENTED_EDGE ( 'NONE', *, *, #10468, .T. ) ;
#6220=LINE ( 'NONE', #1888, #13124 ) ;
#6221=CARTESIAN_POINT ( 'NONE',  ( 22.30340133326367180, 20.00000000000000000, 11.90876978475634651 ) ) ;
#6222=VECTOR ( 'NONE', #9785, 1000.000000000000000 ) ;
#6225=AXIS2_PLACEMENT_3D ( 'NONE', #13596, #4296, #8182 ) ;
#6229=LINE ( 'NONE', #7204, #2097 ) ;
#6230=VERTEX_POINT ( 'NONE', #1961 ) ;
#6232=EDGE_CURVE ( 'NONE', #216, #4054, #9998, .T. ) ;
#6234=DIRECTION ( 'NONE',  ( 0.000000000000000000, 0.000000000000000000, 1.000000000000000000 ) ) ;
#6238=CARTESIAN_POINT ( 'NONE',  ( 30.00000000000001066, 146.6227766016838245, 0.000000000000000000 ) ) ;
#6240=ORIENTED_EDGE ( 'NONE', *, *, #14369, .F. ) ;
#6241=ORIENTED_EDGE ( 'NONE', *, *, #10061, .F. ) ;
#6242=AXIS2_PLACEMENT_3D ( 'NONE', #12694, #8710, #4558 ) ;
#6244=ORIENTED_EDGE ( 'NONE', *, *, #9944, .F. ) ;
#6246=CARTESIAN_POINT ( 'NONE',  ( -16.17053951239850207, 32.72994544565565889, 6.425226171708652956 ) ) ;
#6248=DIRECTION ( 'NONE',  ( 0.000000000000000000, 0.000000000000000000, -1.000000000000000000 ) ) ;
#6250=CARTESIAN_POINT ( 'NONE',  ( 22.93524650466160253, 29.84210526315789025, 5.000000000000003553 ) ) ;
#6251=CARTESIAN_POINT ( 'NONE',  ( 15.56337975240373162, 125.2134999403455851, 5.000000000000083489 ) ) ;
#6252=ORIENTED_EDGE ( 'NONE', *, *, #719, .T. ) ;
#6253=CARTESIAN_POINT ( 'NONE',  ( 18.93231600135347392, 142.3609111598534298, 15.26062816855829851 ) ) ;
#6256=CARTESIAN_POINT ( 'NONE',  ( 34.93420767853316988, 30.00000000000000000, 15.00000000000000000 ) ) ;
#6259=CARTESIAN_POINT ( 'NONE',  ( 14.93242934743711992, 18.00000000000000355, 25.00000000000000000 ) ) ;
#6261=CARTESIAN_POINT ( 'NONE',  ( -80.00000000000001421, 196.6227766016838245, 0.000000000000000000 ) ) ;
#6267=CARTESIAN_POINT ( 'NONE',  ( -27.98221281347037603, 18.00000000000000000, 0.000000000000000000 ) ) ;
#6273=DIRECTION ( 'NONE',  ( 0.000000000000000000, 1.000000000000000000, 0.000000000000000000 ) ) ;
#6276=ORIENTED_EDGE ( 'NONE', *, *, #1796, .F. ) ;
#6281=DIRECTION ( 'NONE',  ( 1.000000000000000000, 0.000000000000000000, 0.000000000000000000 ) ) ;
#6282=VERTEX_POINT ( 'NONE', #8690 ) ;
#6284=ADVANCED_FACE ( 'NONE', ( #1875 ), #549, .T. ) ;
#6286=DIRECTION ( 'NONE',  ( -1.000000000000000000, -0.000000000000000000, -0.000000000000000000 ) ) ;
#6287=CARTESIAN_POINT ( 'NONE',  ( -9.245637070518823109, 17.99999999999769074, 12.12237611798427572 ) ) ;
#6288=DIRECTION ( 'NONE',  ( -0.000000000000000000, -0.000000000000000000, -1.000000000000000000 ) ) ;
#6291=CARTESIAN_POINT ( 'NONE',  ( -80.00000000000002842, 146.6227766016838245, 10.00000000000000178 ) ) ;
#6294=DIRECTION ( 'NONE',  ( 1.000000000000000000, 0.000000000000000000, 0.000000000000000000 ) ) ;
#6298=CARTESIAN_POINT ( 'NONE',  ( 32.29638371061065527, 20.00000000000000355, 15.01265034258821096 ) ) ;
#6299=CARTESIAN_POINT ( 'NONE',  ( 10.22516481506617581, 140.0471213951830407, 11.75777818883246617 ) ) ;
#6300=CARTESIAN_POINT ( 'NONE',  ( 27.13959012325755538, 19.99999999999999645, 20.89788123228700556 ) ) ;
#6302=CARTESIAN_POINT ( 'NONE',  ( 15.00000000000000000, 143.0344144757318929, 16.50549856913627877 ) ) ;
#6303=FACE_OUTER_BOUND ( 'NONE', #7453, .T. ) ;
#6308=DIRECTION ( 'NONE',  ( 0.000000000000000000, 1.000000000000000000, 0.000000000000000000 ) ) ;
#6309=ORIENTED_EDGE ( 'NONE', *, *, #9874, .F. ) ;
#6313=VERTEX_POINT ( 'NONE', #723 ) ;
#6321=CARTESIAN_POINT ( 'NONE',  ( -3.000000000000002665, 144.1839557653416080, 18.33333333333336057 ) ) ;
#6323=CARTESIAN_POINT ( 'NONE',  ( 34.80444759354871564, 18.00000000000000000, 7.621511755358874929 ) ) ;
#6330=CYLINDRICAL_SURFACE ( 'NONE', #5100, 12.00000000000000000 ) ;
#6332=ORIENTED_EDGE ( 'NONE', *, *, #455, .T. ) ;
#6334=CARTESIAN_POINT ( 'NONE',  ( 31.70991205391183954, 201.3251192758334298, 14.38044245167808022 ) ) ;
#6339=ORIENTED_EDGE ( 'NONE', *, *, #17017, .T. ) ;
#6341=EDGE_CURVE ( 'NONE', #9911, #16300, #17268, .T. ) ;
#6363=EDGE_LOOP ( 'NONE', ( #16224, #6631, #11896, #16748 ) ) ;
#6366=DIRECTION ( 'NONE',  ( -1.000000000000000000, 0.000000000000000000, 0.000000000000000000 ) ) ;
#6367=VECTOR ( 'NONE', #5188, 1000.000000000000000 ) ;
#6368=CARTESIAN_POINT ( 'NONE',  ( 34.07008595419463148, 193.7005638513908536, 24.52922227238014941 ) ) ;
#6369=VECTOR ( 'NONE', #4844, 1000.000000000000000 ) ;
#6370=CARTESIAN_POINT ( 'NONE',  ( 196.0000000000000000, 151.6227766016839098, 5.571800142134973655 ) ) ;
#6371=DIRECTION ( 'NONE',  ( 0.000000000000000000, 0.000000000000000000, -1.000000000000000000 ) ) ;
#6372=VECTOR ( 'NONE', #13421, 1000.000000000000000 ) ;
#6373=CARTESIAN_POINT ( 'NONE',  ( -19.80886414215282798, 18.00000000000000000, 20.97268729564153489 ) ) ;
#6374=FACE_OUTER_BOUND ( 'NONE', #11913, .T. ) ;
#6377=CARTESIAN_POINT ( 'NONE',  ( 39.99999999999998579, 20.00000000000000000, 30.00000000000001066 ) ) ;
#6383=AXIS2_PLACEMENT_3D ( 'NONE', #16611, #9870, #8195 ) ;
#6384=ORIENTED_EDGE ( 'NONE', *, *, #13556, .F. ) ;
#6386=CARTESIAN_POINT ( 'NONE',  ( -19.80886414215398261, 19.99999999999999645, 20.97268729564270728 ) ) ;
#6387=CARTESIAN_POINT ( 'NONE',  ( 21.38051303318334462, 141.6185065902053282, 13.74313897096208414 ) ) ;
#6388=CARTESIAN_POINT ( 'NONE',  ( -48.00000000000000000, 204.6227766016838245, 0.000000000000000000 ) ) ;
#6391=ADVANCED_FACE ( 'NONE', ( #2481 ), #7526, .F. ) ;
#6398=AXIS2_PLACEMENT_3D ( 'NONE', #4070, #4155, #16547 ) ;
#6399=EDGE_LOOP ( 'NONE', ( #10043, #11550, #8221, #1513 ) ) ;
#6404=EDGE_LOOP ( 'NONE', ( #11432, #16201, #1369, #695 ) ) ;
#6409=AXIS2_PLACEMENT_3D ( 'NONE', #2465, #1045, #15832 ) ;
#6412=ORIENTED_EDGE ( 'NONE', *, *, #12482, .T. ) ;
#6414=CARTESIAN_POINT ( 'NONE',  ( -11.59473107857741425, 31.35552539902487723, 12.08231249604354574 ) ) ;
#6415=EDGE_CURVE ( 'NONE', #9250, #6665, #2386, .T. ) ;
#6417=EDGE_CURVE ( 'NONE', #938, #7945, #17176, .T. ) ;
#6419=CARTESIAN_POINT ( 'NONE',  ( 22.12396056536369215, 29.85772992373802026, 8.548742771607255264 ) ) ;
#6423=LINE ( 'NONE', #2268, #8895 ) ;
#6427=DIRECTION ( 'NONE',  ( 1.000000000000000000, 0.000000000000000000, 0.000000000000000000 ) ) ;
#6433=CARTESIAN_POINT ( 'NONE',  ( 34.01316144709517886, 199.6193856840139063, 17.47499078086477553 ) ) ;
#6436=DIRECTION ( 'NONE',  ( 1.000000000000000000, 0.000000000000000000, 0.000000000000000000 ) ) ;
#6437=ORIENTED_EDGE ( 'NONE', *, *, #14467, .F. ) ;
#6438=CARTESIAN_POINT ( 'NONE',  ( -83.43212945347822540, 142.9736659102426870, 16.38272693053711393 ) ) ;
#6439=CIRCLE ( 'NONE', #3333, 2.499999999999998668 ) ;
#6440=DIRECTION ( 'NONE',  ( 0.000000000000000000, 0.000000000000000000, -1.000000000000000000 ) ) ;
#6442=DIRECTION ( 'NONE',  ( -1.000000000000000000, -0.000000000000000000, -0.000000000000000000 ) ) ;
#6444=CARTESIAN_POINT ( 'NONE',  ( -5.000000000000000888, 171.6227766016838245, 0.000000000000000000 ) ) ;
#6448=EDGE_CURVE ( 'NONE', #4054, #12800, #1603, .T. ) ;
#6449=ADVANCED_FACE ( 'NONE', ( #9030 ), #15758, .F. ) ;
#6453=AXIS2_PLACEMENT_3D ( 'NONE', #2306, #14118, #6366 ) ;
#6454=ORIENTED_EDGE ( 'NONE', *, *, #17382, .F. ) ;
#6456=ORIENTED_EDGE ( 'NONE', *, *, #4843, .F. ) ;
#6457=CARTESIAN_POINT ( 'NONE',  ( 196.0000000000000000, 159.6227766016838814, 3.071800142134975431 ) ) ;
#6463=CIRCLE ( 'NONE', #7315, 10.00000000000000178 ) ;
#6464=CARTESIAN_POINT ( 'NONE',  ( 35.00000000000000000, 196.6227766016838245, 21.54065922853802206 ) ) ;
#6470=DIRECTION ( 'NONE',  ( 0.000000000000000000, 0.000000000000000000, 1.000000000000000000 ) ) ;
#6478=VECTOR ( 'NONE', #1337, 1000.000000000000000 ) ;
#6479=LINE ( 'NONE', #10726, #3581 ) ;
#6483=CARTESIAN_POINT ( 'NONE',  ( 13.00433657606611604, 139.2454419355441928, 9.442801289196161463 ) ) ;
#6485=CARTESIAN_POINT ( 'NONE',  ( 14.93242934743711814, 20.00000000000000000, 24.99999999999999645 ) ) ;
#6492=EDGE_CURVE ( 'NONE', #11986, #16166, #812, .T. ) ;
#6510=CARTESIAN_POINT ( 'NONE',  ( -8.058782516633090864, 30.15486961025272450, 15.00000000000000178 ) ) ;
#6512=CARTESIAN_POINT ( 'NONE',  ( 29.53214135918722505, 18.00000000000000000, 18.68621337607990185 ) ) ;
#6514=EDGE_CURVE ( 'NONE', #3772, #13139, #17009, .T. ) ;
#6518=PLANE ( 'NONE',  #13707 ) ;
#6519=CARTESIAN_POINT ( 'NONE',  ( 16.97539380423070909, 126.5649914159620266, 7.928130581088665529 ) ) ;
#6523=VERTEX_POINT ( 'NONE', #10446 ) ;
#6524=CARTESIAN_POINT ( 'NONE',  ( 30.00000000000001066, 146.6227766016838245, 0.000000000000000000 ) ) ;
#6525=B_SPLINE_CURVE_WITH_KNOTS ( 'NONE', 3,
 ( #17309, #6510, #9151, #2342, #17125, #14557, #16075, #7732, #2430, #11901, #5177, #14394, #14746, #3955, #10568, #3589, #8004, #3858, #6598, #7655, #9246, #13411, #14653, #10300, #13065, #2531 ),
 .UNSPECIFIED., .F., .F.,
 ( 4, 2, 2, 2, 2, 2, 2, 2, 2, 2, 2, 2, 4 ),
 ( 0.000000000000000000, 0.002066677509289960735, 0.003100016263934941754, 0.004133355018579923205, 0.006200032527869886109, 0.007233371282514866260, 0.008266710037159848146, 0.01033338754644981018, 0.01136672630109478513, 0.01240006505573976354, 0.01446674256502970997, 0.01550008131967467971, 0.01653342007431965119 ),
 .UNSPECIFIED. ) ;
#6529=CARTESIAN_POINT ( 'NONE',  ( 25.00000000000000000, 196.6227766016838245, 21.54065922853802562 ) ) ;
#6539=CARTESIAN_POINT ( 'NONE',  ( -7.379000772444994638, 20.00000000000000000, 25.00000000000000000 ) ) ;
#6540=EDGE_LOOP ( 'NONE', ( #819, #14646 ) ) ;
#6541=CARTESIAN_POINT ( 'NONE',  ( 37.99999999999999289, 2.000000000000000000, 0.000000000000000000 ) ) ;
#6544=AXIS2_PLACEMENT_3D ( 'NONE', #4642, #4299, #577 ) ;
#6551=ORIENTED_EDGE ( 'NONE', *, *, #9166, .T. ) ;
#6552=DIRECTION ( 'NONE',  ( -0.000000000000000000, -0.000000000000000000, -1.000000000000000000 ) ) ;
#6556=EDGE_CURVE ( 'NONE', #2637, #13756, #1238, .T. ) ;
#6559=CARTESIAN_POINT ( 'NONE',  ( -40.00000000000000000, 4.000000000000000000, 33.00000000000000711 ) ) ;
#6560=CARTESIAN_POINT ( 'NONE',  ( 49.99999999999998579, 175.6227766016838530, 16.92820660268601429 ) ) ;
#6561=CYLINDRICAL_SURFACE ( 'NONE', #9516, 30.00000000000000000 ) ;
#6568=ORIENTED_EDGE ( 'NONE', *, *, #9372, .T. ) ;
#6569=DIRECTION ( 'NONE',  ( -1.000000000000000000, -0.000000000000000000, -0.000000000000000000 ) ) ;
#6571=VERTEX_POINT ( 'NONE', #9383 ) ;
#6573=CARTESIAN_POINT ( 'NONE',  ( 13.64704021889961361, 139.0043329719002259, 8.527746218697362934 ) ) ;
#6575=CARTESIAN_POINT ( 'NONE',  ( -48.00000000000000000, 171.6227766016838245, 0.000000000000000000 ) ) ;
#6576=VERTEX_POINT ( 'NONE', #13551 ) ;
#6578=ADVANCED_FACE ( 'NONE', ( #14957 ), #10618, .T. ) ;
#6579=EDGE_CURVE ( 'NONE', #2548, #14798, #6897, .T. ) ;
#6584=ORIENTED_EDGE ( 'NONE', *, *, #15063, .F. ) ;
#6593=ADVANCED_FACE ( 'NONE', ( #8303 ), #13717, .F. ) ;
#6598=CARTESIAN_POINT ( 'NONE',  ( -17.19488518268993715, 32.09742631896689602, 9.330173263366075886 ) ) ;
#6605=CARTESIAN_POINT ( 'NONE',  ( 7.674484246658608733, 133.8653086123773903, 14.91481465347803415 ) ) ;
#6606=CARTESIAN_POINT ( 'NONE',  ( 34.80468147095351128, 17.99999999999999645, 7.619145204522578041 ) ) ;
#6608=EDGE_LOOP ( 'NONE', ( #17484, #4057, #15015 ) ) ;
#6611=CARTESIAN_POINT ( 'NONE',  ( 34.46640061674913369, 198.8884873102157655, 18.59522663992144942 ) ) ;
#6617=ORIENTED_EDGE ( 'NONE', *, *, #14467, .T. ) ;
#6619=CARTESIAN_POINT ( 'NONE',  ( -80.00000000000001421, 196.6227766016838245, 10.00000000000000178 ) ) ;
#6620=CARTESIAN_POINT ( 'NONE',  ( 50.00000000000000000, 171.6227766016838245, 0.000000000000000000 ) ) ;
#6624=CARTESIAN_POINT ( 'NONE',  ( -25.81010901361623056, 20.00000000000000000, 13.97188021846430850 ) ) ;
#6626=ORIENTED_EDGE ( 'NONE', *, *, #14861, .T. ) ;
#6631=ORIENTED_EDGE ( 'NONE', *, *, #2081, .T. ) ;
#6633=LINE ( 'NONE', #3718, #6151 ) ;
#6635=ORIENTED_EDGE ( 'NONE', *, *, #14345, .T. ) ;
#6644=ADVANCED_FACE ( 'NONE', ( #426, #12748 ), #1939, .T. ) ;
#6645=CIRCLE ( 'NONE', #8879, 12.00000000000000000 ) ;
#6647=FACE_OUTER_BOUND ( 'NONE', #3013, .T. ) ;
#6649=VECTOR ( 'NONE', #14445, 1000.000000000000000 ) ;
#6652=ORIENTED_EDGE ( 'NONE', *, *, #15549, .F. ) ;
#6659=CARTESIAN_POINT ( 'NONE',  ( -14.55266450408011636, 19.99999999999999645, 23.76398220081675206 ) ) ;
#6660=CARTESIAN_POINT ( 'NONE',  ( 14.80221254542069076, 126.7206120434983490, 7.900896541359456293 ) ) ;
#6661=AXIS2_PLACEMENT_3D ( 'NONE', #14349, #6286, #17086 ) ;
#6663=CARTESIAN_POINT ( 'NONE',  ( 17.04141343047935564, 29.97166846511136029, 14.77658840773744409 ) ) ;
#6665=VERTEX_POINT ( 'NONE', #4603 ) ;
#6672=CARTESIAN_POINT ( 'NONE',  ( 32.56480294350151183, 150.9309764409412367, 25.70786830908634002 ) ) ;
#6674=ORIENTED_EDGE ( 'NONE', *, *, #5445, .T. ) ;
#6687=CARTESIAN_POINT ( 'NONE',  ( -40.00000000000000000, 0.000000000000000000, 33.00000000000000711 ) ) ;
#6688=AXIS2_PLACEMENT_3D ( 'NONE', #14813, #2610, #17116 ) ;
#6692=DIRECTION ( 'NONE',  ( -1.000000000000000000, 0.000000000000000000, 0.000000000000000000 ) ) ;
#6694=DIRECTION ( 'NONE',  ( 1.000000000000000000, 0.000000000000000000, -0.000000000000000000 ) ) ;
#6695=DIRECTION ( 'NONE',  ( 1.000000000000000000, 0.000000000000000000, 0.000000000000000000 ) ) ;
#6697=CARTESIAN_POINT ( 'NONE',  ( 29.98123639043839006, 18.00000000000000000, 18.19121573219640098 ) ) ;
#6698=FACE_OUTER_BOUND ( 'NONE', #11720, .T. ) ;
#6700=DIRECTION ( 'NONE',  ( 0.8660254037844378194, -0.5000000000000015543, -0.000000000000000000 ) ) ;
#6703=CIRCLE ( 'NONE', #12064, 740.0000000000000000 ) ;
#6704=VECTOR ( 'NONE', #11484, 1000.000000000000000 ) ;
#6710=DIRECTION ( 'NONE',  ( -0.000000000000000000, -1.000000000000000000, 2.312964634635742267E-15 ) ) ;
#6715=CARTESIAN_POINT ( 'NONE',  ( -21.35874126517689930, 20.00000000000000000, 19.71585776365618869 ) ) ;
#6716=VECTOR ( 'NONE', #16452, 1000.000000000000000 ) ;
#6721=EDGE_CURVE ( 'NONE', #4462, #15051, #16554, .T. ) ;
#6723=ORIENTED_EDGE ( 'NONE', *, *, #12848, .T. ) ;
#6732=DIRECTION ( 'NONE',  ( 0.000000000000000000, 0.000000000000000000, -1.000000000000000000 ) ) ;
#6733=DIRECTION ( 'NONE',  ( -1.000000000000000000, 0.000000000000000000, 0.000000000000000000 ) ) ;
#6739=AXIS2_PLACEMENT_3D ( 'NONE', #7045, #4567, #8719 ) ;
#6742=AXIS2_PLACEMENT_3D ( 'NONE', #9720, #85, #2830 ) ;
#6744=CARTESIAN_POINT ( 'NONE',  ( -48.00000000000000000, 171.6227766016838245, 0.000000000000000000 ) ) ;
#6747=VERTEX_POINT ( 'NONE', #3360 ) ;
#6748=DIRECTION ( 'NONE',  ( -1.000000000000000000, -0.000000000000000000, -0.000000000000000000 ) ) ;
#6749=ADVANCED_FACE ( 'NONE', ( #5934 ), #8756, .F. ) ;
#6753=CARTESIAN_POINT ( 'NONE',  ( -12.78554710720352894, 31.18907022382790117, 13.71297843187037202 ) ) ;
#6755=CARTESIAN_POINT ( 'NONE',  ( 18.30724418481818461, 142.5286147297794344, 15.57621362570774437 ) ) ;
#6760=ORIENTED_EDGE ( 'NONE', *, *, #14312, .T. ) ;
#6767=CARTESIAN_POINT ( 'NONE',  ( 29.59441769460779526, 151.6102025845143828, 26.23924109008940420 ) ) ;
#6769=CIRCLE ( 'NONE', #15801, 10.00000000000000000 ) ;
#6772=CIRCLE ( 'NONE', #2232, 2.499999999999998668 ) ;
#6773=CYLINDRICAL_SURFACE ( 'NONE', #2151, 2.500000000000002220 ) ;
#6774=VERTEX_POINT ( 'NONE', #15119 ) ;
#6775=VERTEX_POINT ( 'NONE', #12653 ) ;
#6777=CARTESIAN_POINT ( 'NONE',  ( 13.53786153804125725, 141.8544345782132439, 18.40805394434863018 ) ) ;
#6786=EDGE_CURVE ( 'NONE', #2211, #735, #3002, .T. ) ;
#6789=LINE ( 'NONE', #8186, #13162 ) ;
#6790=ADVANCED_FACE ( 'NONE', ( #13172 ), #12823, .F. ) ;
#6793=LINE ( 'NONE', #3868, #7077 ) ;
#6794=CARTESIAN_POINT ( 'NONE',  ( 22.61491075001043782, 18.00000000000000000, 23.50024419593056635 ) ) ;
#6795=CARTESIAN_POINT ( 'NONE',  ( 196.0000000000000000, 175.6227766016838530, 16.92820660268601429 ) ) ;
#6797=CIRCLE ( 'NONE', #3677, 10.00000000000000178 ) ;
#6798=VECTOR ( 'NONE', #8834, 1000.000000000000000 ) ;
#6803=DIRECTION ( 'NONE',  ( -1.000000000000000000, -0.000000000000000000, -0.000000000000000000 ) ) ;
#6805=DIRECTION ( 'NONE',  ( 0.000000000000000000, -0.8660254037844413721, 0.4999999999999953371 ) ) ;
#6809=CARTESIAN_POINT ( 'NONE',  ( -11.98734322101357641, 20.00000000000000000, 24.50584837321703802 ) ) ;
#6817=ORIENTED_EDGE ( 'NONE', *, *, #4625, .T. ) ;
#6819=AXIS2_PLACEMENT_3D ( 'NONE', #11362, #10349, #3042 ) ;
#6821=EDGE_LOOP ( 'NONE', ( #9192, #1496, #16498, #3716 ) ) ;
#6824=CARTESIAN_POINT ( 'NONE',  ( 27.93429729575420950, 192.0656250386302872, 25.90562197801993349 ) ) ;
#6828=CIRCLE ( 'NONE', #11344, 2.500000000000002220 ) ;
#6833=FACE_OUTER_BOUND ( 'NONE', #14839, .T. ) ;
#6835=DIRECTION ( 'NONE',  ( 0.000000000000000000, 0.000000000000000000, 1.000000000000000000 ) ) ;
#6840=VECTOR ( 'NONE', #1709, 1000.000000000000000 ) ;
#6846=CARTESIAN_POINT ( 'NONE',  ( -725.0000000000000000, 19.99999999999995737, 0.000000000000000000 ) ) ;
#6850=EDGE_CURVE ( 'NONE', #12878, #1164, #2664, .T. ) ;
#6854=ORIENTED_EDGE ( 'NONE', *, *, #10790, .T. ) ;
#6859=EDGE_LOOP ( 'NONE', ( #8165, #16787 ) ) ;
#6860=CARTESIAN_POINT ( 'NONE',  ( 13.85534145189689248, 141.7971685630157879, 18.31519266891907094 ) ) ;
#6861=VERTEX_POINT ( 'NONE', #2367 ) ;
#6864=PLANE ( 'NONE',  #3558 ) ;
#6865=CARTESIAN_POINT ( 'NONE',  ( 30.00000000000000355, 196.6227766016838245, 35.00200000000000244 ) ) ;
#6866=LINE ( 'NONE', #4120, #11604 ) ;
#6870=CARTESIAN_POINT ( 'NONE',  ( 48.00000000000000711, 155.6227766016839098, 12.50000337241049309 ) ) ;
#6871=CARTESIAN_POINT ( 'NONE',  ( -25.00000000000002132, 120.0000000000000284, 5.000000000000023093 ) ) ;
#6872=LINE ( 'NONE', #6795, #3352 ) ;
#6874=VERTEX_POINT ( 'NONE', #7592 ) ;
#6875=CARTESIAN_POINT ( 'NONE',  ( -90.80384757729339640, 138.6227766016838245, 0.000000000000000000 ) ) ;
#6877=ORIENTED_EDGE ( 'NONE', *, *, #8003, .T. ) ;
#6879=CARTESIAN_POINT ( 'NONE',  ( -84.88882470713647876, 145.4280468792801742, 20.09168135694114454 ) ) ;
#6880=DIRECTION ( 'NONE',  ( 1.000000000000000000, 0.000000000000000000, 0.000000000000000000 ) ) ;
#6882=CARTESIAN_POINT ( 'NONE',  ( -38.00000000000000000, 20.00000000000000000, 28.00000000000000355 ) ) ;
#6891=DIRECTION ( 'NONE',  ( 1.000000000000000000, 0.000000000000000000, 0.000000000000000000 ) ) ;
#6893=DIRECTION ( 'NONE',  ( 0.000000000000000000, 0.000000000000000000, 1.000000000000000000 ) ) ;
#6897=LINE ( 'NONE', #170, #2740 ) ;
#6899=CARTESIAN_POINT ( 'NONE',  ( 22.73104287435775461, 29.84603067649059227, 6.814483377121257845 ) ) ;
#6902=EDGE_LOOP ( 'NONE', ( #8997, #16012, #6723, #4114 ) ) ;
#6909=CARTESIAN_POINT ( 'NONE',  ( -14.51002702888200702, 31.55035369552022928, 12.57309263104575869 ) ) ;
#6910=CARTESIAN_POINT ( 'NONE',  ( -18.25212770525996930, 32.30769230769230660, 0.000000000000000000 ) ) ;
#6913=CIRCLE ( 'NONE', #4929, 239.9999999999999716 ) ;
#6918=LINE ( 'NONE', #11158, #16172 ) ;
#6919=VERTEX_POINT ( 'NONE', #8116 ) ;
#6921=ORIENTED_EDGE ( 'NONE', *, *, #17138, .F. ) ;
#6922=CARTESIAN_POINT ( 'NONE',  ( 29.79050797247102977, 151.6222428389254731, 26.24840280143448012 ) ) ;
#6923=EDGE_CURVE ( 'NONE', #2095, #2500, #10593, .T. ) ;
#6925=ADVANCED_FACE ( 'NONE', ( #13529 ), #4061, .T. ) ;
#6932=ORIENTED_EDGE ( 'NONE', *, *, #6556, .F. ) ;
#6935=CARTESIAN_POINT ( 'NONE',  ( 16.61152767523946139, 141.2200844281568379, 17.35152312112458972 ) ) ;
#6945=FACE_OUTER_BOUND ( 'NONE', #12922, .T. ) ;
#6948=VERTEX_POINT ( 'NONE', #17519 ) ;
#6949=CARTESIAN_POINT ( 'NONE',  ( 24.93507336697353693, 29.86842105263157876, 0.000000000000000000 ) ) ;
#6950=CIRCLE ( 'NONE', #15697, 33.00000000000000000 ) ;
#6951=CARTESIAN_POINT ( 'NONE',  ( 27.99999999999998224, 9.999999999999998224, 28.00000000000001066 ) ) ;
#6954=CARTESIAN_POINT ( 'NONE',  ( -100.0000000000000000, 134.2062027339443944, 25.00000000000000000 ) ) ;
#6955=DIRECTION ( 'NONE',  ( -1.000000000000000000, 0.000000000000000000, 0.000000000000000000 ) ) ;
#6958=CIRCLE ( 'NONE', #4967, 9.999999999999998224 ) ;
#6962=ORIENTED_EDGE ( 'NONE', *, *, #4252, .T. ) ;
#6963=EDGE_CURVE ( 'NONE', #2336, #9238, #2012, .T. ) ;
#6971=ORIENTED_EDGE ( 'NONE', *, *, #17461, .T. ) ;
#6974=EDGE_CURVE ( 'NONE', #16869, #9238, #9773, .T. ) ;
#6977=CONICAL_SURFACE ( 'NONE', #9804, 2.499999999999998668, 1.029744260000002187 ) ;
#6980=FACE_BOUND ( 'NONE', #9920, .T. ) ;
#6984=AXIS2_PLACEMENT_3D ( 'NONE', #5321, #12042, #7390 ) ;
#6986=CONICAL_SURFACE ( 'NONE', #7825, 2.499999999999998668, 1.029744260000002187 ) ;
#6987=LINE ( 'NONE', #3181, #5600 ) ;
#6989=DIRECTION ( 'NONE',  ( 0.000000000000000000, 0.000000000000000000, 1.000000000000000000 ) ) ;
#6991=LINE ( 'NONE', #12297, #5636 ) ;
#6994=DIRECTION ( 'NONE',  ( 1.000000000000000000, 0.000000000000000000, -0.000000000000000000 ) ) ;
#6995=ADVANCED_FACE ( 'NONE', ( #16604 ), #15269, .F. ) ;
#7005=CARTESIAN_POINT ( 'NONE',  ( 49.99999999999998579, 179.6227766016838245, 12.50000337241049309 ) ) ;
#7007=CARTESIAN_POINT ( 'NONE',  ( -27.30244652380281778, 19.99999999999999645, 10.27378278477019080 ) ) ;
#7012=AXIS2_PLACEMENT_3D ( 'NONE', #14377, #11540, #6308 ) ;
#7020=EDGE_LOOP ( 'NONE', ( #15492, #13757 ) ) ;
#7023=CYLINDRICAL_SURFACE ( 'NONE', #8746, 2.500000000000000444 ) ;
#7026=VECTOR ( 'NONE', #3554, 1000.000000000000000 ) ;
#7031=CARTESIAN_POINT ( 'NONE',  ( -27.99999999999998224, 10.00000000000000000, 28.00000000000000355 ) ) ;
#7032=CARTESIAN_POINT ( 'NONE',  ( 12.52734837489390785, 131.0783166553242722, 13.12014565386486176 ) ) ;
#7037=CARTESIAN_POINT ( 'NONE',  ( 0.000000000000000000, 20.00000000000000000, 0.000000000000000000 ) ) ;
#7038=DIRECTION ( 'NONE',  ( 0.000000000000000000, 0.000000000000000000, -1.000000000000000000 ) ) ;
#7041=CARTESIAN_POINT ( 'NONE',  ( 17.53546816055560953, 18.00000000000000000, 24.87355917367171187 ) ) ;
#7044=VERTEX_POINT ( 'NONE', #10120 ) ;
#7045=CARTESIAN_POINT ( 'NONE',  ( 40.00000000000000711, 196.6227766016838245, 0.000000000000000000 ) ) ;
#7047=CYLINDRICAL_SURFACE ( 'NONE', #13684, 2.499999999999998668 ) ;
#7051=ORIENTED_EDGE ( 'NONE', *, *, #10810, .T. ) ;
#7052=AXIS2_PLACEMENT_3D ( 'NONE', #2983, #9708, #4148 ) ;
#7053=CARTESIAN_POINT ( 'NONE',  ( 8.431728255697246155, 133.2562109147605156, 12.71722808757355949 ) ) ;
#7055=ORIENTED_EDGE ( 'NONE', *, *, #11643, .F. ) ;
#7059=CYLINDRICAL_SURFACE ( 'NONE', #14016, 20.00000000000000355 ) ;
#7060=CARTESIAN_POINT ( 'NONE',  ( 17.00000000000000000, 154.3022685259950038, 9.999999999999900524 ) ) ;
#7061=DIRECTION ( 'NONE',  ( 0.000000000000000000, 0.000000000000000000, -1.000000000000000000 ) ) ;
#7063=CARTESIAN_POINT ( 'NONE',  ( 6.134011831684049731, 144.1839557653416080, 18.33333333333335702 ) ) ;
#7067=DIRECTION ( 'NONE',  ( 1.000000000000000000, 0.000000000000000000, 0.000000000000000000 ) ) ;
#7071=EDGE_CURVE ( 'NONE', #1654, #4434, #12960, .T. ) ;
#7074=FACE_BOUND ( 'NONE', #3205, .T. ) ;
#7076=AXIS2_PLACEMENT_3D ( 'NONE', #12905, #9805, #16637 ) ;
#7077=VECTOR ( 'NONE', #7836, 1000.000000000000000 ) ;
#7080=VECTOR ( 'NONE', #9616, 1000.000000000000000 ) ;
#7081=DIRECTION ( 'NONE',  ( 0.000000000000000000, 0.000000000000000000, 1.000000000000000000 ) ) ;
#7084=DIRECTION ( 'NONE',  ( -1.000000000000000000, -0.000000000000000000, -0.000000000000000000 ) ) ;
#7085=CARTESIAN_POINT ( 'NONE',  ( -39.68629150101524061, 122.0000000000000000, 9.686291501015231731 ) ) ;
#7086=CARTESIAN_POINT ( 'NONE',  ( -80.94808030731641679, 201.5373699728806400, 13.93281245758934084 ) ) ;
#7087=ORIENTED_EDGE ( 'NONE', *, *, #8673, .T. ) ;
#7089=CYLINDRICAL_SURFACE ( 'NONE', #7226, 10.00000000000000178 ) ;
#7091=DIRECTION ( 'NONE',  ( -1.000000000000000000, 0.000000000000000000, 0.000000000000000000 ) ) ;
#7095=ORIENTED_EDGE ( 'NONE', *, *, #8979, .T. ) ;
#7096=APPLICATION_CONTEXT ( 'automotive_design' ) ;
#7099=CARTESIAN_POINT ( 'NONE',  ( -21.35874126517689220, 18.00000000000000355, 19.71585776365615317 ) ) ;
#7102=DIRECTION ( 'NONE',  ( -1.156482317317868274E-16, 1.000000000000000000, 0.000000000000000000 ) ) ;
#7105=ORIENTED_EDGE ( 'NONE', *, *, #1329, .T. ) ;
#7108=CARTESIAN_POINT ( 'NONE',  ( 27.44407568426044364, 136.8394969516870958, 3.888888888888887063 ) ) ;
#7114=ADVANCED_FACE ( 'NONE', ( #11369 ), #3319, .T. ) ;
#7116=CARTESIAN_POINT ( 'NONE',  ( 6.134011831684049731, 134.2062027339443944, 13.00000000000000000 ) ) ;
#7117=EDGE_CURVE ( 'NONE', #16986, #15774, #6229, .T. ) ;
#7118=CARTESIAN_POINT ( 'NONE',  ( 18.85693063296981009, 140.6075696125688239, 16.22282984566914621 ) ) ;
#7120=ORIENTED_EDGE ( 'NONE', *, *, #1919, .T. ) ;
#7123=FACE_OUTER_BOUND ( 'NONE', #11669, .T. ) ;
#7124=CARTESIAN_POINT ( 'NONE',  ( 15.56337975240373872, 125.2134999403456135, 4.999999999999997335 ) ) ;
#7125=CARTESIAN_POINT ( 'NONE',  ( 196.0000000000000000, 159.6227766016838814, 5.571800142134975431 ) ) ;
#7126=CARTESIAN_POINT ( 'NONE',  ( -27.98221281347037959, 20.00000000000000000, 4.999999999999999112 ) ) ;
#7127=VERTEX_POINT ( 'NONE', #15528 ) ;
#7132=CARTESIAN_POINT ( 'NONE',  ( 225.0000000000000000, 89.99999999999997158, 4.999999999999999112 ) ) ;
#7133=ORIENTED_EDGE ( 'NONE', *, *, #9213, .F. ) ;
#7135=ORIENTED_EDGE ( 'NONE', *, *, #4257, .T. ) ;
#7136=CARTESIAN_POINT ( 'NONE',  ( 8.856485326996372365, 132.9846638168478137, 12.59946789408625456 ) ) ;
#7147=CARTESIAN_POINT ( 'NONE',  ( 25.11117529286356742, 145.4280468792802026, 20.09168135694114099 ) ) ;
#7149=DIRECTION ( 'NONE',  ( 0.000000000000000000, 0.000000000000000000, -1.000000000000000000 ) ) ;
#7150=DIRECTION ( 'NONE',  ( -0.000000000000000000, -1.000000000000000000, -0.000000000000000000 ) ) ;
#7156=DIRECTION ( 'NONE',  ( -1.000000000000000000, 0.000000000000000000, 0.000000000000000000 ) ) ;
#7160=EDGE_CURVE ( 'NONE', #9285, #3708, #14233, .T. ) ;
#7161=DIRECTION ( 'NONE',  ( -1.000000000000000000, 0.000000000000000000, 0.000000000000000000 ) ) ;
#7162=CARTESIAN_POINT ( 'NONE',  ( 26.58318862804039640, 192.9554221994867476, 25.17938093289615509 ) ) ;
#7173=DIRECTION ( 'NONE',  ( 0.000000000000000000, 0.8660254037844413721, -0.4999999999999952816 ) ) ;
#7178=CARTESIAN_POINT ( 'NONE',  ( -17.58288004918493996, 18.00000000000000000, 22.43027208364173575 ) ) ;
#7187=ADVANCED_FACE ( 'NONE', ( #1618 ), #199, .T. ) ;
#7188=ORIENTED_EDGE ( 'NONE', *, *, #5030, .F. ) ;
#7190=LINE ( 'NONE', #4460, #4424 ) ;
#7193=CARTESIAN_POINT ( 'NONE',  ( -23.00000000000001421, 122.0000000000000284, 4.999999999999999112 ) ) ;
#7194=AXIS2_PLACEMENT_3D ( 'NONE', #12065, #15144, #3024 ) ;
#7197=CARTESIAN_POINT ( 'NONE',  ( 15.82262738632537946, 137.2266821760960340, 8.447647312139547893 ) ) ;
#7200=DIRECTION ( 'NONE',  ( 0.01578383822436034076, -0.1110972697184772484, -0.9936841888205766304 ) ) ;
#7201=CARTESIAN_POINT ( 'NONE',  ( -75.46415429630739879, 194.4969340293140476, 23.78882387388087238 ) ) ;
#7202=CARTESIAN_POINT ( 'NONE',  ( 14.93242934743711992, 30.00000000000000000, 15.00000000000000000 ) ) ;
#7203=CARTESIAN_POINT ( 'NONE',  ( 21.98114852961722576, 18.00000000000000000, 23.72829316725777815 ) ) ;
#7204=CARTESIAN_POINT ( 'NONE',  ( -45.00000000000000000, 140.0000000000000000, 0.000000000000000000 ) ) ;
#7210=CIRCLE ( 'NONE', #10893, 2.500000000000002220 ) ;
#7211=DIRECTION ( 'NONE',  ( -0.000000000000000000, -0.000000000000000000, -1.000000000000000000 ) ) ;
#7213=CARTESIAN_POINT ( 'NONE',  ( -15.00000000000002665, 130.0000000000000000, 15.00000000000000000 ) ) ;
#7220=VERTEX_POINT ( 'NONE', #8073 ) ;
#7221=DIRECTION ( 'NONE',  ( -1.000000000000000000, -0.000000000000000000, -0.000000000000000000 ) ) ;
#7223=ORIENTED_EDGE ( 'NONE', *, *, #12229, .F. ) ;
#7224=DIRECTION ( 'NONE',  ( -0.000000000000000000, -0.000000000000000000, -1.000000000000000000 ) ) ;
#7226=AXIS2_PLACEMENT_3D ( 'NONE', #8502, #3009, #15045 ) ;
#7227=CARTESIAN_POINT ( 'NONE',  ( 48.00000000000000711, 191.6227766016837677, 3.071800142134975431 ) ) ;
#7230=CARTESIAN_POINT ( 'NONE',  ( -68.00000000000000000, 171.6227766016838245, 0.000000000000000000 ) ) ;
#7231=ORIENTED_EDGE ( 'NONE', *, *, #17518, .F. ) ;
#7232=CARTESIAN_POINT ( 'NONE',  ( 33.63865905896372510, 143.1809062453614843, 16.74061342279919984 ) ) ;
#7235=AXIS2_PLACEMENT_3D ( 'NONE', #9494, #9847, #1459 ) ;
#7237=VECTOR ( 'NONE', #14758, 1000.000000000000000 ) ;
#7239=EDGE_LOOP ( 'NONE', ( #15223, #1691, #10121, #11615 ) ) ;
#7240=CARTESIAN_POINT ( 'NONE',  ( -40.00000000000000000, 20.00000000000000000, 0.000000000000000000 ) ) ;
#7243=CIRCLE ( 'NONE', #1879, 30.00000000000000000 ) ;
#7246=DIRECTION ( 'NONE',  ( 0.000000000000000000, 0.000000000000000000, -1.000000000000000000 ) ) ;
#7251=VERTEX_POINT ( 'NONE', #17475 ) ;
#7252=DIRECTION ( 'NONE',  ( 0.000000000000000000, 0.000000000000000000, 1.000000000000000000 ) ) ;
#7254=CARTESIAN_POINT ( 'NONE',  ( -79.09267923946974577, 201.5450689758321232, 13.91624649103837719 ) ) ;
#7259=AXIS2_PLACEMENT_3D ( 'NONE', #6559, #2582, #11949 ) ;
#7261=CIRCLE ( 'NONE', #7535, 8.000000000000000000 ) ;
#7265=CARTESIAN_POINT ( 'NONE',  ( -27.98221281347037959, 30.00000000000000000, 15.00000000000000000 ) ) ;
#7274=DIRECTION ( 'NONE',  ( -1.156482317317868274E-16, 1.000000000000000000, 0.000000000000000000 ) ) ;
#7278=ORIENTED_EDGE ( 'NONE', *, *, #13141, .F. ) ;
#7285=CARTESIAN_POINT ( 'NONE',  ( 27.44407568426047206, 136.8394969516870958, 3.888888888888889728 ) ) ;
#7286=CARTESIAN_POINT ( 'NONE',  ( 25.02538947967125793, 138.3580044269788800, 10.92703196337285299 ) ) ;
#7290=CARTESIAN_POINT ( 'NONE',  ( 48.00000000000000711, 187.6227766016837961, 12.50000337241049309 ) ) ;
#7291=FACE_OUTER_BOUND ( 'NONE', #4248, .T. ) ;
#7293=CARTESIAN_POINT ( 'NONE',  ( -38.00000000000000000, 18.00000000000000355, 28.00000000000000355 ) ) ;
#7294=CARTESIAN_POINT ( 'NONE',  ( 17.52334770333193248, 18.00000000000113332, 12.62810114740270606 ) ) ;
#7301=ORIENTED_EDGE ( 'NONE', *, *, #4463, .T. ) ;
#7306=ORIENTED_EDGE ( 'NONE', *, *, #11443, .T. ) ;
#7308=CARTESIAN_POINT ( 'NONE',  ( 10.76597736162413632, 139.9178931572356532, 11.43282512092270053 ) ) ;
#7309=ORIENTED_EDGE ( 'NONE', *, *, #15450, .F. ) ;
#7311=ORIENTED_EDGE ( 'NONE', *, *, #2781, .F. ) ;
#7312=ADVANCED_FACE ( 'NONE', ( #12323 ), #16416, .F. ) ;
#7315=AXIS2_PLACEMENT_3D ( 'NONE', #9301, #10808, #10722 ) ;
#7316=DIRECTION ( 'NONE',  ( -0.000000000000000000, -0.000000000000000000, -1.000000000000000000 ) ) ;
#7317=EDGE_CURVE ( 'NONE', #1461, #14379, #2960, .T. ) ;
#7319=CARTESIAN_POINT ( 'NONE',  ( 15.04007972439966956, 126.3543340278276190, 7.435061541642935978 ) ) ;
#7321=LINE ( 'NONE', #15367, #15125 ) ;
#7323=CARTESIAN_POINT ( 'NONE',  ( 25.00000000000001066, 146.0036328918050970, 20.82208359987472335 ) ) ;
#7324=DIRECTION ( 'NONE',  ( -0.000000000000000000, -0.000000000000000000, -1.000000000000000000 ) ) ;
#7329=VECTOR ( 'NONE', #3054, 1000.000000000000000 ) ;
#7333=CARTESIAN_POINT ( 'NONE',  ( -80.00000000000002842, 146.6227766016838245, 0.000000000000000000 ) ) ;
#7338=CARTESIAN_POINT ( 'NONE',  ( 24.48161681970857018, 138.6020828307752879, 11.64873334838780572 ) ) ;
#7345=DIRECTION ( 'NONE',  ( 1.000000000000000000, 0.000000000000000000, -0.000000000000000000 ) ) ;
#7347=CARTESIAN_POINT ( 'NONE',  ( -79.78392266530065058, 201.6195082837481323, 13.75486997215864093 ) ) ;
#7359=ORIENTED_EDGE ( 'NONE', *, *, #917, .T. ) ;
#7362=( BOUNDED_CURVE ( )  B_SPLINE_CURVE ( 3, ( #3551, #4960, #3643, #12939 ),
 .UNSPECIFIED., .F., .F. ) 
 B_SPLINE_CURVE_WITH_KNOTS ( ( 4, 4 ),
 ( 4.712388980384692339, 6.283185307179586232 ),
 .UNSPECIFIED. ) 
 CURVE ( )  GEOMETRIC_REPRESENTATION_ITEM ( )  RATIONAL_B_SPLINE_CURVE ( ( 1.000000000000000000, 0.8047378541243654926, 0.8047378541243654926, 1.000000000000000000 ) ) 
 REPRESENTATION_ITEM ( '' )  );
#7367=CARTESIAN_POINT ( 'NONE',  ( -27.30244652380281778, 18.00000000000000000, 10.27378278477019080 ) ) ;
#7370=DIRECTION ( 'NONE',  ( -0.000000000000000000, -0.000000000000000000, 1.000000000000000000 ) ) ;
#7378=EDGE_CURVE ( 'NONE', #9236, #15970, #15413, .T. ) ;
#7379=CARTESIAN_POINT ( 'NONE',  ( 34.93420767853314146, 20.00000000000000000, 6.320602137672510779 ) ) ;
#7381=CARTESIAN_POINT ( 'NONE',  ( 25.49876332522151401, 19.99999999999999645, 21.99427390110736624 ) ) ;
#7386=DIRECTION ( 'NONE',  ( -0.000000000000000000, -0.000000000000000000, -1.000000000000000000 ) ) ;
#7388=CARTESIAN_POINT ( 'NONE',  ( -80.18730344621531003, 191.6224348813836116, 26.24906986711107848 ) ) ;
#7390=DIRECTION ( 'NONE',  ( 0.000000000000000000, 0.000000000000000000, -1.000000000000000000 ) ) ;
#7392=ORIENTED_EDGE ( 'NONE', *, *, #12412, .F. ) ;
#7394=CIRCLE ( 'NONE', #8510, 5.000000000000004441 ) ;
#7403=PLANE ( 'NONE',  #7934 ) ;
#7404=CARTESIAN_POINT ( 'NONE',  ( 13.21952030233119046, 128.8713892059273860, 10.07325499884888664 ) ) ;
#7413=CARTESIAN_POINT ( 'NONE',  ( 49.99999999999998579, 175.6227766016838245, 3.071800142134975431 ) ) ;
#7415=CYLINDRICAL_SURFACE ( 'NONE', #7076, 5.000000000000004441 ) ;
#7417=LINE ( 'NONE', #693, #8397 ) ;
#7419=CARTESIAN_POINT ( 'NONE',  ( 27.44407568426044364, 136.8394969516870958, 3.888888888888887063 ) ) ;
#7420=DIRECTION ( 'NONE',  ( 1.000000000000000000, 0.000000000000000000, 0.000000000000000000 ) ) ;
#7424=CARTESIAN_POINT ( 'NONE',  ( 49.99999999999998579, 175.6227766016838245, 5.571800142134975431 ) ) ;
#7425=CARTESIAN_POINT ( 'NONE',  ( 196.0000000000000000, 187.6227766016837961, 15.00000337241049486 ) ) ;
#7426=LINE ( 'NONE', #706, #12022 ) ;
#7428=EDGE_CURVE ( 'NONE', #4551, #3972, #8518, .T. ) ;
#7430=EDGE_CURVE ( 'NONE', #7044, #13835, #12769, .T. ) ;
#7436=CARTESIAN_POINT ( 'NONE',  ( 49.99999999999998579, 163.6227766016838530, 10.00000337241049309 ) ) ;
#7439=CARTESIAN_POINT ( 'NONE',  ( 196.0000000000000000, 151.6227766016839098, 8.071800142134973655 ) ) ;
#7442=CARTESIAN_POINT ( 'NONE',  ( -27.98221281341758626, 18.00000000000000000, 6.321711414556880904 ) ) ;
#7446=FACE_OUTER_BOUND ( 'NONE', #4776, .T. ) ;
#7447=VERTEX_POINT ( 'NONE', #4708 ) ;
#7448=DIRECTION ( 'NONE',  ( 0.000000000000000000, 0.000000000000000000, -1.000000000000000000 ) ) ;
#7452=DIRECTION ( 'NONE',  ( 0.000000000000000000, 0.000000000000000000, 1.000000000000000000 ) ) ;
#7453=EDGE_LOOP ( 'NONE', ( #3337, #14814, #7950, #1742 ) ) ;
#7455=LINE ( 'NONE', #742, #4425 ) ;
#7456=CARTESIAN_POINT ( 'NONE',  ( -83.65340775248648697, 193.1938012187559366, 24.97603563008316385 ) ) ;
#7457=FACE_OUTER_BOUND ( 'NONE', #4509, .T. ) ;
#7458=EDGE_CURVE ( 'NONE', #5446, #16788, #640, .T. ) ;
#7459=DIRECTION ( 'NONE',  ( 0.000000000000000000, -0.8660254037844413721, 0.4999999999999953371 ) ) ;
#7460=DIRECTION ( 'NONE',  ( 0.000000000000000000, 0.000000000000000000, 1.000000000000000000 ) ) ;
#7462=ORIENTED_EDGE ( 'NONE', *, *, #4402, .T. ) ;
#7466=CARTESIAN_POINT ( 'NONE',  ( -90.33974596215564645, 171.6227766016838245, 0.000000000000000000 ) ) ;
#7481=LINE ( 'NONE', #6164, #6369 ) ;
#7487=LINE ( 'NONE', #10149, #8209 ) ;
#7489=CARTESIAN_POINT ( 'NONE',  ( 17.00000000000000000, 191.6227766016837961, -1.224646799147353454E-15 ) ) ;
#7495=ORIENTED_EDGE ( 'NONE', *, *, #8629, .T. ) ;
#7502=ADVANCED_FACE ( 'NONE', ( #13107 ), #13197, .F. ) ;
#7507=DIRECTION ( 'NONE',  ( 0.000000000000000000, 0.000000000000000000, 1.000000000000000000 ) ) ;
#7512=ORIENTED_EDGE ( 'NONE', *, *, #2532, .F. ) ;
#7516=CYLINDRICAL_SURFACE ( 'NONE', #5564, 5.000000000000000888 ) ;
#7517=VECTOR ( 'NONE', #4884, 1000.000000000000000 ) ;
#7520=ORIENTED_EDGE ( 'NONE', *, *, #1052, .F. ) ;
#7524=EDGE_CURVE ( 'NONE', #10721, #15996, #7362, .T. ) ;
#7526=CYLINDRICAL_SURFACE ( 'NONE', #7805, 2.499999999999998668 ) ;
#7528=CARTESIAN_POINT ( 'NONE',  ( -13.45813206906208848, 31.92660440999782523, 10.88283926110020516 ) ) ;
#7529=DIRECTION ( 'NONE',  ( -1.000000000000000000, 0.000000000000000000, 0.000000000000000000 ) ) ;
#7535=AXIS2_PLACEMENT_3D ( 'NONE', #10445, #3906, #9292 ) ;
#7536=ORIENTED_EDGE ( 'NONE', *, *, #2566, .T. ) ;
#7541=ORIENTED_EDGE ( 'NONE', *, *, #6579, .F. ) ;
#7543=CARTESIAN_POINT ( 'NONE',  ( 22.52789404479186786, 20.00000000000113687, 11.66574595783169954 ) ) ;
#7548=CARTESIAN_POINT ( 'NONE',  ( 15.00000000000000000, 143.1210915093834330, 16.64102305613075572 ) ) ;
#7554=LINE ( 'NONE', #10287, #1082 ) ;
#7556=ORIENTED_EDGE ( 'NONE', *, *, #2108, .T. ) ;
#7560=CIRCLE ( 'NONE', #15764, 740.0000000000000000 ) ;
#7561=ORIENTED_EDGE ( 'NONE', *, *, #15602, .T. ) ;
#7562=ORIENTED_EDGE ( 'NONE', *, *, #14110, .F. ) ;
#7564=CIRCLE ( 'NONE', #15478, 2.500000000000000000 ) ;
#7565=EDGE_CURVE ( 'NONE', #3708, #10702, #6645, .T. ) ;
#7566=DIRECTION ( 'NONE',  ( -1.000000000000000000, -0.000000000000000000, -0.000000000000000000 ) ) ;
#7569=DIRECTION ( 'NONE',  ( 1.000000000000000000, 0.000000000000000000, 0.000000000000000000 ) ) ;
#7570=CARTESIAN_POINT ( 'NONE',  ( 22.88332935572807969, 29.84310215611307271, 6.048604702147989620 ) ) ;
#7571=CARTESIAN_POINT ( 'NONE',  ( -43.00000000000000000, 140.0000000000000000, 0.000000000000000000 ) ) ;
#7572=CIRCLE ( 'NONE', #4755, 2.500000000000002220 ) ;
#7573=AXIS2_PLACEMENT_3D ( 'NONE', #14782, #1152, #14866 ) ;
#7574=COLOUR_RGB ( '', 0.09019608, 0.27058824, 0.51372549) ;
#7577=DIRECTION ( 'NONE',  ( 0.000000000000000000, 0.000000000000000000, -1.000000000000000000 ) ) ;
#7580=DIRECTION ( 'NONE',  ( -1.000000000000000000, -0.000000000000000000, -0.000000000000000000 ) ) ;
#7581=CARTESIAN_POINT ( 'NONE',  ( 30.56782666082448330, 201.5917424073649613, 13.81529814621278085 ) ) ;
#7582=AXIS2_PLACEMENT_3D ( 'NONE', #8857, #16839, #15770 ) ;
#7584=EDGE_CURVE ( 'NONE', #3061, #6774, #133, .T. ) ;
#7589=CARTESIAN_POINT ( 'NONE',  ( 27.44407568426044008, 126.9014170516880284, 4.999999999999997335 ) ) ;
#7590=DIRECTION ( 'NONE',  ( 1.000000000000000000, 0.000000000000000000, -0.000000000000000000 ) ) ;
#7592=CARTESIAN_POINT ( 'NONE',  ( -24.99999999999999289, 90.00000000000000000, 4.999999999999999112 ) ) ;
#7593=ADVANCED_FACE ( 'NONE', ( #6374 ), #15666, .F. ) ;
#7595=DIRECTION ( 'NONE',  ( -0.000000000000000000, -0.000000000000000000, 1.000000000000000000 ) ) ;
#7597=FACE_OUTER_BOUND ( 'NONE', #13495, .T. ) ;
#7598=VECTOR ( 'NONE', #12071, 1000.000000000000000 ) ;
#7605=ORIENTED_EDGE ( 'NONE', *, *, #10394, .F. ) ;
#7608=AXIS2_PLACEMENT_3D ( 'NONE', #4412, #1753, #5651 ) ;
#7610=CIRCLE ( 'NONE', #15249, 248.0000000000000000 ) ;
#7615=CARTESIAN_POINT ( 'NONE',  ( -12.63609539511579527, 18.00000000000000000, 24.35132453916584794 ) ) ;
#7618=ORIENTED_EDGE ( 'NONE', *, *, #250, .T. ) ;
#7623=AXIS2_PLACEMENT_3D ( 'NONE', #3780, #15824, #3611 ) ;
#7625=ADVANCED_FACE ( 'NONE', ( #17012 ), #2220, .T. ) ;
#7627=CARTESIAN_POINT ( 'NONE',  ( 48.00000000000000711, 183.6227766016837961, 8.071800142134975431 ) ) ;
#7628=DIRECTION ( 'NONE',  ( 0.000000000000000000, -0.000000000000000000, -1.000000000000000000 ) ) ;
#7629=CARTESIAN_POINT ( 'NONE',  ( 22.45383620668762248, 29.90040889522806111, 11.60055593449971845 ) ) ;
#7630=VECTOR ( 'NONE', #4506, 1000.000000000000000 ) ;
#7632=EDGE_LOOP ( 'NONE', ( #6921, #10128, #16246 ) ) ;
#7635=CARTESIAN_POINT ( 'NONE',  ( -100.0000000000000000, 171.6227766016838245, 0.000000000000000000 ) ) ;
#7642=DIRECTION ( 'NONE',  ( 0.000000000000000000, 0.000000000000000000, 1.000000000000000000 ) ) ;
#7645=ORIENTED_EDGE ( 'NONE', *, *, #4820, .F. ) ;
#7646=ADVANCED_FACE ( 'NONE', ( #4878 ), #15765, .F. ) ;
#7648=EDGE_CURVE ( 'NONE', #4086, #15544, #6913, .T. ) ;
#7649=ORIENTED_EDGE ( 'NONE', *, *, #2366, .T. ) ;
#7654=CARTESIAN_POINT ( 'NONE',  ( -8.461393309425545795, 30.35704578695612099, 12.95687587100684368 ) ) ;
#7655=CARTESIAN_POINT ( 'NONE',  ( -17.63576980228536328, 32.18555361985414720, 8.400096275226864861 ) ) ;
#7658=CARTESIAN_POINT ( 'NONE',  ( 34.93420767782698988, 18.00000000000000000, 6.321724734778991106 ) ) ;
#7659=DIRECTION ( 'NONE',  ( -1.000000000000000000, -0.000000000000000000, -0.000000000000000000 ) ) ;
#7661=DIRECTION ( 'NONE',  ( -0.000000000000000000, -0.000000000000000000, -1.000000000000000000 ) ) ;
#7665=CARTESIAN_POINT ( 'NONE',  ( 24.93507336697353338, 29.86842105263157521, 5.660390792616599498 ) ) ;
#7669=CARTESIAN_POINT ( 'NONE',  ( 31.52313204192882523, 201.3896308033654634, 14.24607874381217520 ) ) ;
#7674=CARTESIAN_POINT ( 'NONE',  ( -77.05212259621265503, 142.5723011982437072, 15.66001370690270633 ) ) ;
#7676=PLANE ( 'NONE',  #10699 ) ;
#7678=EDGE_LOOP ( 'NONE', ( #5537, #10886, #3508, #4604 ) ) ;
#7680=DIRECTION ( 'NONE',  ( -1.000000000000000000, -0.000000000000000000, -0.000000000000000000 ) ) ;
#7694=VERTEX_POINT ( 'NONE', #13555 ) ;
#7696=LINE ( 'NONE', #15262, #16149 ) ;
#7697=CARTESIAN_POINT ( 'NONE',  ( 39.99999999999999289, 20.00000000000000000, 0.000000000000000000 ) ) ;
#7698=LINE ( 'NONE', #15937, #2691 ) ;
#7699=CARTESIAN_POINT ( 'NONE',  ( -11.31385407355777950, 31.26810920821015216, 12.21116371260378308 ) ) ;
#7701=DIRECTION ( 'NONE',  ( -1.000000000000000000, 0.000000000000000000, 0.000000000000000000 ) ) ;
#7702=CARTESIAN_POINT ( 'NONE',  ( -151.9615242270660929, 171.6227766016838245, 0.000000000000000000 ) ) ;
#7704=CARTESIAN_POINT ( 'NONE',  ( 196.0000000000000000, 151.6227766016839098, 5.571800142134973655 ) ) ;
#7705=ORIENTED_EDGE ( 'NONE', *, *, #5497, .T. ) ;
#7707=PLANE ( 'NONE',  #8663 ) ;
#7708=ORIENTED_EDGE ( 'NONE', *, *, #3478, .F. ) ;
#7711=CARTESIAN_POINT ( 'NONE',  ( 15.22098041563561388, 126.0279773824920824, 6.884464680362713196 ) ) ;
#7712=CARTESIAN_POINT ( 'NONE',  ( 22.95484754400920124, 19.99999999999884537, 11.15425480658508306 ) ) ;
#7727=B_SPLINE_CURVE_WITH_KNOTS ( 'NONE', 3,
 ( #11899, #3953, #7654, #3856, #9245, #3588, #6414, #1108, #13064, #2169, #14297, #855, #2341, #9068, #17308, #5262, #15891, #6246, #3682, #2259, #5176, #10567 ),
 .UNSPECIFIED., .F., .F.,
 ( 4, 2, 2, 2, 2, 2, 2, 2, 2, 2, 4 ),
 ( 0.000000000000000000, 0.001700754388868652408, 0.003401508777737304815, 0.005102263166605957440, 0.005952640361040282234, 0.006803017555474607028, 0.008503771944343253147, 0.01020452633321189927, 0.01190528072208054712, 0.01275565791651486931, 0.01360603511094918977 ),
 .UNSPECIFIED. ) ;
#7732=CARTESIAN_POINT ( 'NONE',  ( -11.99846793330598693, 31.02137248309377071, 14.08482506821421509 ) ) ;
#7735=CARTESIAN_POINT ( 'NONE',  ( 22.93524650466135739, 29.84210526317653489, 5.528689893908154573 ) ) ;
#7737=CARTESIAN_POINT ( 'NONE',  ( 40.00000000000000711, 196.6227766016838245, 0.000000000000000000 ) ) ;
#7740=CARTESIAN_POINT ( 'NONE',  ( 19.59022622986824302, 142.1737554346910599, 14.89790021284453303 ) ) ;
#7742=AXIS2_PLACEMENT_3D ( 'NONE', #10109, #14198, #826 ) ;
#7745=CARTESIAN_POINT ( 'NONE',  ( 23.61565302391275267, 29.88537503463918554, 10.00682404417760551 ) ) ;
#7749=EDGE_LOOP ( 'NONE', ( #7984, #9500, #15376, #14398 ) ) ;
#7754=CARTESIAN_POINT ( 'NONE',  ( -82.07464743585514100, 142.0696621759509810, 14.68466941333284126 ) ) ;
#7760=FACE_OUTER_BOUND ( 'NONE', #14481, .T. ) ;
#7763=FILL_AREA_STYLE_COLOUR ( '', #2706 ) ;
#7771=LINE ( 'NONE', #6457, #6128 ) ;
#7773=EDGE_LOOP ( 'NONE', ( #6309, #6635, #12971, #13650 ) ) ;
#7774=DIRECTION ( 'NONE',  ( 1.000000000000000000, 0.000000000000000000, 0.000000000000000000 ) ) ;
#7776=ADVANCED_FACE ( 'NONE', ( #10805 ), #4008, .F. ) ;
#7780=CARTESIAN_POINT ( 'NONE',  ( 33.65098944192141772, 193.2024116766813222, 24.96685975555417514 ) ) ;
#7781=DIRECTION ( 'NONE',  ( 0.000000000000000000, 0.000000000000000000, -1.000000000000000000 ) ) ;
#7782=CARTESIAN_POINT ( 'NONE',  ( 196.0000000000000000, 171.6227766016838245, 10.00000337241048953 ) ) ;
#7785=DIRECTION ( 'NONE',  ( -1.000000000000000000, 0.000000000000000000, 0.000000000000000000 ) ) ;
#7787=ORIENTED_EDGE ( 'NONE', *, *, #11965, .T. ) ;
#7788=CYLINDRICAL_SURFACE ( 'NONE', #531, 2.500000000000000444 ) ;
#7790=CARTESIAN_POINT ( 'NONE',  ( 37.99999999999999289, 2.000000000000000000, 8.789265611615818404E-15 ) ) ;
#7791=VECTOR ( 'NONE', #12592, 1000.000000000000000 ) ;
#7796=VERTEX_POINT ( 'NONE', #5491 ) ;
#7798=CARTESIAN_POINT ( 'NONE',  ( 14.44088586081352688, 138.6571688462224472, 6.678806037552732278 ) ) ;
#7801=EDGE_CURVE ( 'NONE', #4462, #3385, #9037, .T. ) ;
#7805=AXIS2_PLACEMENT_3D ( 'NONE', #6206, #13027, #3806 ) ;
#7808=DIRECTION ( 'NONE',  ( -1.000000000000000000, -0.000000000000000000, -0.000000000000000000 ) ) ;
#7818=DIRECTION ( 'NONE',  ( -1.000000000000000000, 0.000000000000000000, 0.000000000000000000 ) ) ;
#7823=VECTOR ( 'NONE', #12916, 1000.000000000000000 ) ;
#7825=AXIS2_PLACEMENT_3D ( 'NONE', #10850, #5380, #8202 ) ;
#7830=CARTESIAN_POINT ( 'NONE',  ( 21.28500206399612438, 29.87397908709612082, 9.872681979495178339 ) ) ;
#7832=ORIENTED_EDGE ( 'NONE', *, *, #8067, .F. ) ;
#7833=CARTESIAN_POINT ( 'NONE',  ( -40.00000000000000000, 20.00000000000000000, 30.00000000000000355 ) ) ;
#7836=DIRECTION ( 'NONE',  ( -0.000000000000000000, -0.000000000000000000, -1.000000000000000000 ) ) ;
#7838=CARTESIAN_POINT ( 'NONE',  ( 15.00000000000000000, 171.6227766016838245, 0.000000000000000000 ) ) ;
#7839=CARTESIAN_POINT ( 'NONE',  ( 16.24588547270996131, 29.98230316816100327, 14.93526533897157726 ) ) ;
#7841=LINE ( 'NONE', #13253, #3842 ) ;
#7842=CARTESIAN_POINT ( 'NONE',  ( -32.99999999999998579, 10.00000000000000000, 28.00000000000000355 ) ) ;
#7845=ORIENTED_EDGE ( 'NONE', *, *, #5596, .T. ) ;
#7847=B_SPLINE_CURVE_WITH_KNOTS ( 'NONE', 3,
 ( #1388, #10768, #1118, #14831, #9426, #2711, #6794, #3963, #1293, #9256, #10495, #4050, #12188, #6697, #9077, #15900, #7933, #2439, #14485, #3770, #9164, #11819, #6606, #2352, #12097 ),
 .UNSPECIFIED., .F., .F.,
 ( 4, 2, 2, 1, 2, 2, 2, 2, 2, 2, 2, 2, 4 ),
 ( 0.000000000000000000, 0.003937549356687076833, 0.005906324035030613949, 0.007875098713374151932, 0.009843873391717689048, 0.01181264807006122616, 0.01575019742674830733, 0.01771897210509184445, 0.01968774678343538503, 0.02362529614012245927, 0.02559407081846599985, 0.02756284549680953697, 0.03150039485349661467 ),
 .UNSPECIFIED. ) ;
#7848=EDGE_LOOP ( 'NONE', ( #1382, #15338 ) ) ;
#7851=CARTESIAN_POINT ( 'NONE',  ( -84.18069928808040459, 143.8651737624333862, 17.85267748742823457 ) ) ;
#7856=CARTESIAN_POINT ( 'NONE',  ( 15.00000000000000000, 143.0344144757318929, 16.50549856913627877 ) ) ;
#7859=PRESENTATION_STYLE_ASSIGNMENT (( #5204 ) ) ;
#7862=ORIENTED_EDGE ( 'NONE', *, *, #10597, .T. ) ;
#7864=EDGE_CURVE ( 'NONE', #8265, #647, #10428, .T. ) ;
#7866=EDGE_CURVE ( 'NONE', #13670, #12384, #4520, .T. ) ;
#7867=ORIENTED_EDGE ( 'NONE', *, *, #11333, .T. ) ;
#7873=DIRECTION ( 'NONE',  ( 0.000000000000000000, -0.000000000000000000, 1.000000000000000000 ) ) ;
#7876=CONICAL_SURFACE ( 'NONE', #2806, 33.26794919243112503, 0.5235987755983005920 ) ;
#7879=CARTESIAN_POINT ( 'NONE',  ( -32.99999999999998579, 10.00000000000000000, 35.00200000000000244 ) ) ;
#7881=LINE ( 'NONE', #8801, #11762 ) ;
#7882=DIRECTION ( 'NONE',  ( -0.000000000000000000, -0.000000000000000000, -1.000000000000000000 ) ) ;
#7883=DIRECTION ( 'NONE',  ( 0.000000000000000000, 0.000000000000000000, 1.000000000000000000 ) ) ;
#7885=EDGE_LOOP ( 'NONE', ( #9051, #7921 ) ) ;
#7890=LINE ( 'NONE', #12144, #16678 ) ;
#7891=AXIS2_PLACEMENT_3D ( 'NONE', #14328, #7680, #11585 ) ;
#7895=CARTESIAN_POINT ( 'NONE',  ( 27.50000000000000355, 196.6227766016838245, 10.00000000000000178 ) ) ;
#7897=CARTESIAN_POINT ( 'NONE',  ( 20.41303537789175948, 141.9260521957599508, 14.39564681615556907 ) ) ;
#7903=CIRCLE ( 'NONE', #3090, 12.00000000000000000 ) ;
#7908=FACE_OUTER_BOUND ( 'NONE', #4725, .T. ) ;
#7913=ORIENTED_EDGE ( 'NONE', *, *, #5054, .T. ) ;
#7914=ORIENTED_EDGE ( 'NONE', *, *, #9808, .T. ) ;
#7918=CARTESIAN_POINT ( 'NONE',  ( 27.99999999999998224, 9.999999999999998224, 28.00000000000001066 ) ) ;
#7919=AXIS2_PLACEMENT_3D ( 'NONE', #6619, #3976, #5195 ) ;
#7920=EDGE_CURVE ( 'NONE', #8790, #3840, #15260, .T. ) ;
#7921=ORIENTED_EDGE ( 'NONE', *, *, #15361, .F. ) ;
#7925=DIRECTION ( 'NONE',  ( -1.000000000000000000, 0.000000000000000000, 0.000000000000000000 ) ) ;
#7926=DIRECTION ( 'NONE',  ( -1.000000000000000000, -0.000000000000000000, -0.000000000000000000 ) ) ;
#7932=CARTESIAN_POINT ( 'NONE',  ( 11.67974368446408384, 131.7296502858855547, 13.62018484423547804 ) ) ;
#7933=CARTESIAN_POINT ( 'NONE',  ( 32.29638371061065527, 18.00000000000000000, 15.01265034258821096 ) ) ;
#7934=AXIS2_PLACEMENT_3D ( 'NONE', #4751, #596, #13964 ) ;
#7935=CARTESIAN_POINT ( 'NONE',  ( 14.93242934743711992, 30.00000000000000000, 15.00000000000000000 ) ) ;
#7937=FACE_OUTER_BOUND ( 'NONE', #1892, .T. ) ;
#7940=ORIENTED_EDGE ( 'NONE', *, *, #13564, .F. ) ;
#7945=VERTEX_POINT ( 'NONE', #13009 ) ;
#7946=CARTESIAN_POINT ( 'NONE',  ( -80.24502126479927711, 141.6230733471410304, 13.74837463607935284 ) ) ;
#7949=CARTESIAN_POINT ( 'NONE',  ( -23.65835920965562877, 20.00000000000000000, 17.33937328557894020 ) ) ;
#7950=ORIENTED_EDGE ( 'NONE', *, *, #8067, .T. ) ;
#7962=ORIENTED_EDGE ( 'NONE', *, *, #2836, .T. ) ;
#7963=DIRECTION ( 'NONE',  ( -0.000000000000000000, -0.000000000000000000, -1.000000000000000000 ) ) ;
#7964=CARTESIAN_POINT ( 'NONE',  ( -43.00000000000003553, 134.2062027339443944, 13.00000000000000000 ) ) ;
#7971=ADVANCED_FACE ( 'NONE', ( #9184 ), #10515, .F. ) ;
#7978=VERTEX_POINT ( 'NONE', #3621 ) ;
#7979=CARTESIAN_POINT ( 'NONE',  ( -23.00000000000000000, 120.0000000000000284, 4.999999999999999112 ) ) ;
#7981=VERTEX_POINT ( 'NONE', #15918 ) ;
#7982=CARTESIAN_POINT ( 'NONE',  ( -9.825395436088792067, 30.54854208321445341, 14.75250191942001088 ) ) ;
#7983=CARTESIAN_POINT ( 'NONE',  ( 13.73607130285257227, 138.7967234794239459, 3.453855393586055200 ) ) ;
#7984=ORIENTED_EDGE ( 'NONE', *, *, #2896, .F. ) ;
#7988=CARTESIAN_POINT ( 'NONE',  ( 48.00000000000000711, 187.6227766016837961, 10.00000337241049309 ) ) ;
#7991=ORIENTED_EDGE ( 'NONE', *, *, #4685, .T. ) ;
#7992=CARTESIAN_POINT ( 'NONE',  ( 26.57851455615899994, 150.2853719096988812, 25.17531865327014629 ) ) ;
#7997=ORIENTED_EDGE ( 'NONE', *, *, #1438, .F. ) ;
#8003=EDGE_CURVE ( 'NONE', #17055, #3234, #5944, .T. ) ;
#8004=CARTESIAN_POINT ( 'NONE',  ( -16.66926302330761800, 31.99181794709938487, 10.22419352058821396 ) ) ;
#8007=CARTESIAN_POINT ( 'NONE',  ( -80.99255306636646878, 151.5270838226223873, 26.17568438743892045 ) ) ;
#8009=DIRECTION ( 'NONE',  ( 0.000000000000000000, 1.000000000000000000, 0.000000000000000000 ) ) ;
#8011=CARTESIAN_POINT ( 'NONE',  ( 196.0000000000000000, 183.6227766016837961, 3.071800142134975431 ) ) ;
#8012=CARTESIAN_POINT ( 'NONE',  ( 48.00000000000000711, 171.6227766016838245, 0.000000000000000000 ) ) ;
#8013=CARTESIAN_POINT ( 'NONE',  ( -48.00000000000000000, 171.6227766016838245, 20.00000000000000355 ) ) ;
#8015=DIRECTION ( 'NONE',  ( -1.000000000000000000, 0.000000000000000000, -0.000000000000000000 ) ) ;
#8016=LINE ( 'NONE', #1630, #8039 ) ;
#8017=CARTESIAN_POINT ( 'NONE',  ( 32.50000000000000711, 146.6227766016838245, 10.00000000000000178 ) ) ;
#8021=CARTESIAN_POINT ( 'NONE',  ( -75.13467353717234687, 145.4324535730256969, 20.08206597984644048 ) ) ;
#8027=VERTEX_POINT ( 'NONE', #956 ) ;
#8028=DIRECTION ( 'NONE',  ( -1.000000000000000000, 0.000000000000000000, -2.312964634635742464E-16 ) ) ;
#8039=VECTOR ( 'NONE', #4464, 1000.000000000000000 ) ;
#8040=ORIENTED_EDGE ( 'NONE', *, *, #13824, .F. ) ;
#8043=ORIENTED_EDGE ( 'NONE', *, *, #2843, .F. ) ;
#8048=DIRECTION ( 'NONE',  ( -1.000000000000000000, -0.000000000000000000, -0.000000000000000000 ) ) ;
#8053=LINE ( 'NONE', #13463, #6478 ) ;
#8061=CARTESIAN_POINT ( 'NONE',  ( -12.16365208422963740, 31.05675767351161909, 14.01395464075509878 ) ) ;
#8062=CARTESIAN_POINT ( 'NONE',  ( 27.44407568426053246, 138.8271129316868837, 3.666666666666671404 ) ) ;
#8064=ORIENTED_EDGE ( 'NONE', *, *, #5830, .F. ) ;
#8067=EDGE_CURVE ( 'NONE', #16869, #9322, #6797, .T. ) ;
#8069=ORIENTED_EDGE ( 'NONE', *, *, #7430, .F. ) ;
#8073=CARTESIAN_POINT ( 'NONE',  ( 32.99999999999998579, 9.999999999999998224, 0.000000000000000000 ) ) ;
#8076=VECTOR ( 'NONE', #11025, 1000.000000000000000 ) ;
#8083=ORIENTED_EDGE ( 'NONE', *, *, #790, .F. ) ;
#8086=CYLINDRICAL_SURFACE ( 'NONE', #3343, 5.000000000000018652 ) ;
#8088=ORIENTED_EDGE ( 'NONE', *, *, #14110, .T. ) ;
#8089=CARTESIAN_POINT ( 'NONE',  ( -80.00000000000002842, 146.6227766016838245, 0.000000000000000000 ) ) ;
#8090=AXIS2_PLACEMENT_3D ( 'NONE', #11704, #13133, #1002 ) ;
#8091=CARTESIAN_POINT ( 'NONE',  ( -95.00000000000000000, 141.6227766016838245, -5.510910596163088767E-15 ) ) ;
#8093=CARTESIAN_POINT ( 'NONE',  ( 15.00000000000000000, 171.6227766016838245, 0.000000000000000000 ) ) ;
#8094=CARTESIAN_POINT ( 'NONE',  ( -75.34926945688242483, 148.4807726931354068, 23.52860204907123887 ) ) ;
#8100=DIRECTION ( 'NONE',  ( 1.000000000000000000, 0.000000000000000000, 0.000000000000000000 ) ) ;
#8106=AXIS2_PLACEMENT_3D ( 'NONE', #806, #4614, #8769 ) ;
#8107=DIRECTION ( 'NONE',  ( 1.000000000000000000, 0.000000000000000000, 0.000000000000000000 ) ) ;
#8109=DIRECTION ( 'NONE',  ( 0.000000000000000000, 0.000000000000000000, -1.000000000000000000 ) ) ;
#8116=CARTESIAN_POINT ( 'NONE',  ( 24.93507336697352628, 29.86842105263157876, 4.999999999999999112 ) ) ;
#8129=PRODUCT_DEFINITION_FORMATION_WITH_SPECIFIED_SOURCE ( 'ANY', '', #1782, .NOT_KNOWN. ) ;
#8133=ORIENTED_EDGE ( 'NONE', *, *, #15224, .F. ) ;
#8136=ADVANCED_FACE ( 'NONE', ( #1492 ), #4149, .F. ) ;
#8137=CYLINDRICAL_SURFACE ( 'NONE', #7573, 2.500000000000000444 ) ;
#8138=CARTESIAN_POINT ( 'NONE',  ( 34.65161675558235999, 194.7673412502506665, 23.52603474534220140 ) ) ;
#8143=AXIS2_PLACEMENT_3D ( 'NONE', #4047, #13605, #6694 ) ;
#8150=ORIENTED_EDGE ( 'NONE', *, *, #15327, .F. ) ;
#8154=CARTESIAN_POINT ( 'NONE',  ( -18.25212770525392614, 32.30769230766699707, 5.660855707253096725 ) ) ;
#8155=DIRECTION ( 'NONE',  ( 0.000000000000000000, 0.000000000000000000, 1.000000000000000000 ) ) ;
#8160=ORIENTED_EDGE ( 'NONE', *, *, #174, .F. ) ;
#8162=DIRECTION ( 'NONE',  ( 0.000000000000000000, 0.000000000000000000, -1.000000000000000000 ) ) ;
#8165=ORIENTED_EDGE ( 'NONE', *, *, #14180, .F. ) ;
#8175=ORIENTED_EDGE ( 'NONE', *, *, #7524, .F. ) ;
#8177=CARTESIAN_POINT ( 'NONE',  ( 7.098239199201186622, 139.5131674267937569, 14.94273745766416184 ) ) ;
#8179=ORIENTED_EDGE ( 'NONE', *, *, #13973, .T. ) ;
#8182=DIRECTION ( 'NONE',  ( 0.000000000000000000, 1.000000000000000000, 0.000000000000000000 ) ) ;
#8183=VECTOR ( 'NONE', #8263, 1000.000000000000000 ) ;
#8184=FACE_OUTER_BOUND ( 'NONE', #14980, .T. ) ;
#8186=CARTESIAN_POINT ( 'NONE',  ( 125.0000000000000000, 0.000000000000000000, 0.000000000000000000 ) ) ;
#8187=EDGE_LOOP ( 'NONE', ( #10679, #4012 ) ) ;
#8189=EDGE_CURVE ( 'NONE', #10010, #2606, #10738, .T. ) ;
#8192=ADVANCED_FACE ( 'NONE', ( #5472 ), #2733, .T. ) ;
#8195=DIRECTION ( 'NONE',  ( 0.000000000000000000, 0.000000000000000000, 1.000000000000000000 ) ) ;
#8201=EDGE_LOOP ( 'NONE', ( #6384, #670, #2827, #14075, #17040 ) ) ;
#8202=DIRECTION ( 'NONE',  ( -1.000000000000000000, 0.000000000000000000, 0.000000000000000000 ) ) ;
#8203=EDGE_LOOP ( 'NONE', ( #11353, #837, #4036, #13276 ) ) ;
#8209=VECTOR ( 'NONE', #1020, 1000.000000000000000 ) ;
#8213=DIRECTION ( 'NONE',  ( -1.000000000000000000, -0.000000000000000000, -0.000000000000000000 ) ) ;
#8218=ORIENTED_EDGE ( 'NONE', *, *, #7565, .T. ) ;
#8221=ORIENTED_EDGE ( 'NONE', *, *, #10404, .T. ) ;
#8222=DIRECTION ( 'NONE',  ( 1.000000000000000000, 0.000000000000000000, 0.000000000000000000 ) ) ;
#8229=DIRECTION ( 'NONE',  ( -1.000000000000000000, 0.000000000000000000, -0.000000000000000000 ) ) ;
#8234=DIRECTION ( 'NONE',  ( 0.000000000000000000, 0.000000000000000000, -1.000000000000000000 ) ) ;
#8240=DIRECTION ( 'NONE',  ( -0.000000000000000000, -0.000000000000000000, 1.000000000000000000 ) ) ;
#8242=FACE_OUTER_BOUND ( 'NONE', #2003, .T. ) ;
#8251=ORIENTED_EDGE ( 'NONE', *, *, #17473, .F. ) ;
#8253=ORIENTED_EDGE ( 'NONE', *, *, #14772, .F. ) ;
#8254=CARTESIAN_POINT ( 'NONE',  ( 25.53453899454350307, 148.8772865214096441, 23.90975478891752815 ) ) ;
#8255=ORIENTED_EDGE ( 'NONE', *, *, #9290, .T. ) ;
#8258=FACE_BOUND ( 'NONE', #3775, .T. ) ;
#8259=ADVANCED_FACE ( 'NONE', ( #9367 ), #11392, .F. ) ;
#8260=FACE_OUTER_BOUND ( 'NONE', #5336, .T. ) ;
#8263=DIRECTION ( 'NONE',  ( -1.000000000000000000, -0.000000000000000000, -0.000000000000000000 ) ) ;
#8264=CARTESIAN_POINT ( 'NONE',  ( 6.134011831684059501, 134.2062027339443944, 14.99999999999999822 ) ) ;
#8265=VERTEX_POINT ( 'NONE', #12468 ) ;
#8266=ADVANCED_FACE ( 'NONE', ( #335, #16800, #15105, #12374, #247, #8560, #3170, #3079, #2017, #3249, #8480, #414, #16460, #5820 ), #5652, .T. ) ;
#8270=DIRECTION ( 'NONE',  ( -1.000000000000000000, 0.000000000000000000, 0.000000000000000000 ) ) ;
#8271=CARTESIAN_POINT ( 'NONE',  ( -75.00000000000002842, 146.6227766016838245, 21.54065922853802562 ) ) ;
#8272=EDGE_LOOP ( 'NONE', ( #10430, #13179 ) ) ;
#8274=CARTESIAN_POINT ( 'NONE',  ( 15.00000000000000000, 171.6227766016838245, 20.00000000000000355 ) ) ;
#8280=ORIENTED_EDGE ( 'NONE', *, *, #3790, .F. ) ;
#8283=EDGE_CURVE ( 'NONE', #11917, #11907, #5736, .T. ) ;
#8285=EDGE_CURVE ( 'NONE', #1227, #10007, #4413, .T. ) ;
#8287=ADVANCED_FACE ( 'NONE', ( #4667 ), #605, .T. ) ;
#8302=CARTESIAN_POINT ( 'NONE',  ( 26.34659224751355211, 193.1938012187558797, 24.97603563008314254 ) ) ;
#8303=FACE_OUTER_BOUND ( 'NONE', #15199, .T. ) ;
#8305=CARTESIAN_POINT ( 'NONE',  ( 21.87945022329474298, 29.86245334106958538, 9.005757899690800983 ) ) ;
#8306=DIRECTION ( 'NONE',  ( 0.000000000000000000, 0.000000000000000000, -1.000000000000000000 ) ) ;
#8313=CARTESIAN_POINT ( 'NONE',  ( -7.379000772445021283, 30.00000000000000000, 13.00000000000000000 ) ) ;
#8314=CARTESIAN_POINT ( 'NONE',  ( -95.00000000000000000, 171.6227766016838245, 0.000000000000000000 ) ) ;
#8317=CARTESIAN_POINT ( 'NONE',  ( -21.36854569161992856, 19.99999999999999645, 19.70709815271291632 ) ) ;
#8318=FACE_OUTER_BOUND ( 'NONE', #674, .T. ) ;
#8319=ORIENTED_EDGE ( 'NONE', *, *, #11083, .T. ) ;
#8323=CARTESIAN_POINT ( 'NONE',  ( -25.81010901361623056, 18.00000000000000000, 13.97188021846430139 ) ) ;
#8325=CIRCLE ( 'NONE', #16821, 20.00000000000000355 ) ;
#8327=DIRECTION ( 'NONE',  ( -1.156482317317868274E-16, 1.000000000000000000, 0.000000000000000000 ) ) ;
#8328=CARTESIAN_POINT ( 'NONE',  ( -70.00000000000000000, 143.0439382767972631, 16.49999999999984013 ) ) ;
#8329=ORIENTED_EDGE ( 'NONE', *, *, #5051, .T. ) ;
#8332=ORIENTED_EDGE ( 'NONE', *, *, #8571, .T. ) ;
#8334=ORIENTED_EDGE ( 'NONE', *, *, #15065, .T. ) ;
#8337=VECTOR ( 'NONE', #9177, 1000.000000000000000 ) ;
#8340=VERTEX_POINT ( 'NONE', #4501 ) ;
#8342=CYLINDRICAL_SURFACE ( 'NONE', #16847, 5.000000000000018652 ) ;
#8345=CARTESIAN_POINT ( 'NONE',  ( 11.61835878478676598, 131.7755375868723320, 13.65455057792075877 ) ) ;
#8354=CARTESIAN_POINT ( 'NONE',  ( 34.93420767853316988, 19.99999999999999645, 0.000000000000000000 ) ) ;
#8355=CARTESIAN_POINT ( 'NONE',  ( -725.0000000000000000, 19.99999999999995737, 15.00000000000000000 ) ) ;
#8356=VECTOR ( 'NONE', #5375, 1000.000000000000000 ) ;
#8357=EDGE_LOOP ( 'NONE', ( #9219, #8485 ) ) ;
#8363=LINE ( 'NONE', #1650, #14311 ) ;
#8369=AXIS2_PLACEMENT_3D ( 'NONE', #3944, #2334, #923 ) ;
#8372=VERTEX_POINT ( 'NONE', #11124 ) ;
#8383=AXIS2_PLACEMENT_3D ( 'NONE', #10528, #8048, #13287 ) ;
#8384=CARTESIAN_POINT ( 'NONE',  ( -3.000000000000000888, 171.6227766016838245, 0.000000000000000000 ) ) ;
#8386=AXIS2_PLACEMENT_3D ( 'NONE', #2825, #6891, #11050 ) ;
#8388=EDGE_CURVE ( 'NONE', #2665, #12251, #4589, .T. ) ;
#8391=FACE_BOUND ( 'NONE', #3531, .T. ) ;
#8397=VECTOR ( 'NONE', #12995, 1000.000000000000000 ) ;
#8398=CYLINDRICAL_SURFACE ( 'NONE', #6742, 2.500000000000000444 ) ;
#8400=CARTESIAN_POINT ( 'NONE',  ( -90.80384757729339640, 204.6227766016838245, 0.000000000000000000 ) ) ;
#8401=LINE ( 'NONE', #12483, #12358 ) ;
#8402=CARTESIAN_POINT ( 'NONE',  ( 16.75836516268004317, 29.96322345091821049, 12.79344305462037035 ) ) ;
#8403=CARTESIAN_POINT ( 'NONE',  ( -84.59204834251386274, 198.6215000397446886, 18.98099903503496577 ) ) ;
#8407=VECTOR ( 'NONE', #10950, 1000.000000000000000 ) ;
#8408=ADVANCED_FACE ( 'NONE', ( #17051 ), #13074, .F. ) ;
#8411=CARTESIAN_POINT ( 'NONE',  ( -40.00000000000000000, 4.000000000000000000, 33.00000000000000711 ) ) ;
#8424=CYLINDRICAL_SURFACE ( 'NONE', #15797, 20.00000000000000355 ) ;
#8426=ADVANCED_FACE ( 'NONE', ( #11474 ), #4761, .T. ) ;
#8428=B_SPLINE_CURVE_WITH_KNOTS ( 'NONE', 3,
 ( #4660, #1916, #16970, #7319, #3502, #12725, #597, #7404, #11386, #15459, #677, #11467, #11559, #16879, #4752, #10142, #15547, #2084, #767, #6163 ),
 .UNSPECIFIED., .F., .F.,
 ( 4, 2, 2, 2, 2, 2, 2, 2, 2, 4 ),
 ( 0.000000000000000000, 0.002053780611527093129, 0.004107561223054186257, 0.006161341834581279819, 0.008215122446108372514, 0.01026890305763546694, 0.01232268366916255964, 0.01437646428068965233, 0.01540335458645322037, 0.01643024489221679013 ),
 .UNSPECIFIED. ) ;
#8435=AXIS2_PLACEMENT_3D ( 'NONE', #12328, #4105, #9489 ) ;
#8438=FACE_OUTER_BOUND ( 'NONE', #10075, .T. ) ;
#8439=VECTOR ( 'NONE', #6805, 1000.000000000000114 ) ;
#8447=VECTOR ( 'NONE', #5299, 1000.000000000000000 ) ;
#8448=CARTESIAN_POINT ( 'NONE',  ( -100.0000000000000000, 171.6227766016838245, 0.000000000000000000 ) ) ;
#8451=CIRCLE ( 'NONE', #10712, 239.9999999999999716 ) ;
#8452=CARTESIAN_POINT ( 'NONE',  ( -13.90980987654335976, 19.99999999999998934, 23.98326992096530219 ) ) ;
#8453=EDGE_CURVE ( 'NONE', #5896, #16720, #7487, .T. ) ;
#8455=CARTESIAN_POINT ( 'NONE',  ( 48.00000000000000711, 163.6227766016838530, 12.50000337241049309 ) ) ;
#8457=CARTESIAN_POINT ( 'NONE',  ( -725.0000000000000000, 19.99999999999995737, 15.00000000000000000 ) ) ;
#8458=CYLINDRICAL_SURFACE ( 'NONE', #14954, 8.000000000000000000 ) ;
#8460=ORIENTED_EDGE ( 'NONE', *, *, #2896, .T. ) ;
#8463=ADVANCED_FACE ( 'NONE', ( #14307 ), #6330, .T. ) ;
#8464=VECTOR ( 'NONE', #14062, 1000.000000000000000 ) ;
#8465=CARTESIAN_POINT ( 'NONE',  ( 10.91733900447548322, 143.9222794873857652, 17.93588862913478366 ) ) ;
#8466=VECTOR ( 'NONE', #2841, 1000.000000000000000 ) ;
#8468=CARTESIAN_POINT ( 'NONE',  ( 27.48361012698968864, 136.6227766016838245, 0.000000000000000000 ) ) ;
#8477=CARTESIAN_POINT ( 'NONE',  ( 30.91638155568829660, 141.7021811473759669, 13.91989935049638305 ) ) ;
#8480=FACE_BOUND ( 'NONE', #12643, .T. ) ;
#8481=CIRCLE ( 'NONE', #9040, 2.500000000000002220 ) ;
#8482=DIRECTION ( 'NONE',  ( -0.000000000000000000, -0.000000000000000000, -1.000000000000000000 ) ) ;
#8484=CARTESIAN_POINT ( 'NONE',  ( 48.00000000000000711, 163.6227766016838530, 10.00000337241049309 ) ) ;
#8485=ORIENTED_EDGE ( 'NONE', *, *, #5899, .F. ) ;
#8489=VERTEX_POINT ( 'NONE', #3598 ) ;
#8491=FACE_OUTER_BOUND ( 'NONE', #11757, .T. ) ;
#8493=CARTESIAN_POINT ( 'NONE',  ( 25.08013182200793878, 195.5664139939901816, 22.72185355927996042 ) ) ;
#8496=CARTESIAN_POINT ( 'NONE',  ( 22.51550247401197069, 29.85017970947654575, 7.570302168957804057 ) ) ;
#8497=CARTESIAN_POINT ( 'NONE',  ( -77.77775085091418816, 201.1051302811612231, 14.82644580554059743 ) ) ;
#8499=ORIENTED_EDGE ( 'NONE', *, *, #7801, .T. ) ;
#8502=CARTESIAN_POINT ( 'NONE',  ( 34.93420767853316988, 30.00000000000000000, 15.00000000000000000 ) ) ;
#8503=CIRCLE ( 'NONE', #6819, 20.00000000000000355 ) ;
#8507=DIRECTION ( 'NONE',  ( 0.000000000000000000, 0.000000000000000000, 1.000000000000000000 ) ) ;
#8510=AXIS2_PLACEMENT_3D ( 'NONE', #5072, #15524, #10471 ) ;
#8513=EDGE_CURVE ( 'NONE', #4855, #190, #14993, .T. ) ;
#8518=LINE ( 'NONE', #12502, #17085 ) ;
#8519=DIRECTION ( 'NONE',  ( 0.000000000000000000, 0.000000000000000000, -1.000000000000000000 ) ) ;
#8523=CARTESIAN_POINT ( 'NONE',  ( 27.47054928355543169, 136.6945666198121216, 2.592592592592591672 ) ) ;
#8529=CARTESIAN_POINT ( 'NONE',  ( 49.99999999999998579, 187.6227766016837961, 10.00000337241049309 ) ) ;
#8530=CARTESIAN_POINT ( 'NONE',  ( 16.64812168497169864, 126.9869021000460663, 8.626120676703536105 ) ) ;
#8535=CARTESIAN_POINT ( 'NONE',  ( -82.86886491573849867, 192.5125816722295724, 25.54797519334867673 ) ) ;
#8536=CARTESIAN_POINT ( 'NONE',  ( 15.60228996708978855, 124.9392590763941371, -1.387778780781445676E-14 ) ) ;
#8537=CARTESIAN_POINT ( 'NONE',  ( 17.58250999373992585, 125.2198453306090329, -1.325401613797208934E-14 ) ) ;
#8538=CARTESIAN_POINT ( 'NONE',  ( 196.0000000000000000, 191.6227766016837677, 5.571800142134975431 ) ) ;
#8544=CARTESIAN_POINT ( 'NONE',  ( 49.99999999999998579, 151.6227766016839098, 8.071800142134973655 ) ) ;
#8545=ORIENTED_EDGE ( 'NONE', *, *, #10597, .F. ) ;
#8546=ORIENTED_EDGE ( 'NONE', *, *, #5922, .F. ) ;
#8551=DIRECTION ( 'NONE',  ( -1.000000000000000000, -0.000000000000000000, -0.000000000000000000 ) ) ;
#8552=ORIENTED_EDGE ( 'NONE', *, *, #10374, .T. ) ;
#8557=ORIENTED_EDGE ( 'NONE', *, *, #719, .F. ) ;
#8558=CARTESIAN_POINT ( 'NONE',  ( 34.20572221690138548, 143.8556217771935053, 17.85322440072383543 ) ) ;
#8560=FACE_BOUND ( 'NONE', #17483, .T. ) ;
#8565=EDGE_CURVE ( 'NONE', #12513, #1130, #1117, .T. ) ;
#8569=CARTESIAN_POINT ( 'NONE',  ( 17.91514137517177474, 140.8731888928338094, 16.72020691847105667 ) ) ;
#8571=EDGE_CURVE ( 'NONE', #3946, #14086, #14431, .T. ) ;
#8572=CARTESIAN_POINT ( 'NONE',  ( 28.65205091688542893, 191.8039921295446106, 26.10980206683225902 ) ) ;
#8573=EDGE_CURVE ( 'NONE', #5381, #8372, #6793, .T. ) ;
#8575=EDGE_CURVE ( 'NONE', #8489, #9733, #1048, .T. ) ;
#8578=CARTESIAN_POINT ( 'NONE',  ( -82.70586383762018556, 200.8416626254457640, 15.34246182976911932 ) ) ;
#8580=VERTEX_POINT ( 'NONE', #2438 ) ;
#8583=CARTESIAN_POINT ( 'NONE',  ( -40.00000000000000000, 20.00000000000000000, 30.00000000000000355 ) ) ;
#8589=ORIENTED_EDGE ( 'NONE', *, *, #14106, .F. ) ;
#8591=( BOUNDED_SURFACE ( )  B_SPLINE_SURFACE ( 3, 2, ( 
 ( #16618, #13959, #1822 ),
 ( #4488, #14454, #16524 ),
 ( #12620, #16789, #9044 ),
 ( #8465, #11294, #12536 ),
 ( #13881, #14050, #7053 ),
 ( #9875, #3334, #7136 ),
 ( #4577, #6299, #401 ),
 ( #12454, #1910, #9958 ),
 ( #15282, #7308, #12715 ),
 ( #3155, #591, #5989 ),
 ( #8954, #14363, #2320 ),
 ( #6755, #6483, #14626 ),
 ( #1172, #2499, #2402 ),
 ( #16144, #6573, #13476 ),
 ( #7897, #13305, #15867 ),
 ( #6387, #10731, #3923 ),
 ( #9397, #11877, #11964 ),
 ( #5425, #7798, #15949 ),
 ( #2596, #12152, #10815 ),
 ( #5154, #22, #13119 ),
 ( #9472, #13210, #4018 ),
 ( #983, #14800, #6660 ),
 ( #17366, #4094, #17282 ),
 ( #14721, #11783, #16226 ),
 ( #1080, #3826, #5237 ),
 ( #12055, #17190, #7711 ),
 ( #10543, #9218, #9127 ),
 ( #5066, #9310, #10639 ),
 ( #16046, #7983, #2672 ),
 ( #8062, #13384, #1252 ) ),
 .UNSPECIFIED., .F., .F., .F. ) 
 B_SPLINE_SURFACE_WITH_KNOTS ( ( 4, 2, 2, 2, 2, 2, 2, 2, 2, 2, 2, 2, 2, 2, 4 ),
 ( 3, 3 ),
 ( 0.01165250788892075590, 0.01579789672993321681, 0.01787059115043944726, 0.01890693836069256423, 0.01994328557094567772, 0.02408867441195813863, 0.02616136883246436562, 0.02823406325297059608, 0.03030675767347682653, 0.03237945209398305352, 0.03652484093499551443, 0.03859753535550174142, 0.03963388256575485491, 0.04067022977600797534, 0.04481561861702043625 ),
 ( 0.000000000000000000, 1.000000000000000000 ),
 .UNSPECIFIED. ) 
 GEOMETRIC_REPRESENTATION_ITEM ( )  RATIONAL_B_SPLINE_SURFACE ( (
 ( 1.000000000000000000, 0.8819171036881968684, 1.000000000000000000),
 ( 1.000000000000000000, 0.8793942645247271317, 1.000000000000000000),
 ( 1.000000000000000000, 0.8749458316895473153, 1.000000000000000000),
 ( 1.000000000000000000, 0.8656814021268807169, 1.000000000000000000),
 ( 1.000000000000000000, 0.8621600075895787807, 1.000000000000000000),
 ( 1.000000000000000000, 0.8562492930711512740, 1.000000000000000000),
 ( 1.000000000000000000, 0.8541736901086096623, 1.000000000000000000),
 ( 1.000000000000000000, 0.8498659178638878764, 1.000000000000000000),
 ( 1.000000000000000000, 0.8476283308600994770, 1.000000000000000000),
 ( 1.000000000000000000, 0.8360458749413697266, 1.000000000000000000),
 ( 1.000000000000000000, 0.8255221978283152628, 1.000000000000000000),
 ( 1.000000000000000000, 0.8082270345000643896, 1.000000000000000000),
 ( 1.000000000000000000, 0.8022128341713220534, 1.000000000000000000),
 ( 1.000000000000000000, 0.7899684886175323273, 1.000000000000000000),
 ( 1.000000000000000000, 0.7837128169312477244, 1.000000000000000000),
 ( 1.000000000000000000, 0.7710263478628327505, 1.000000000000000000),
 ( 1.000000000000000000, 0.7645952338537677084, 1.000000000000000000),
 ( 1.000000000000000000, 0.7516613202047349729, 1.000000000000000000),
 ( 1.000000000000000000, 0.7451386183435962929, 1.000000000000000000),
 ( 1.000000000000000000, 0.7257808243687768890, 1.000000000000000000),
 ( 1.000000000000000000, 0.7133953845776382918, 1.000000000000000000),
 ( 1.000000000000000000, 0.6965170042221158209, 1.000000000000000000),
 ( 1.000000000000000000, 0.6911767420096451842, 1.000000000000000000),
 ( 1.000000000000000000, 0.6837405640632109316, 1.000000000000000000),
 ( 1.000000000000000000, 0.6813577907324296357, 1.000000000000000000),
 ( 1.000000000000000000, 0.6768117804540668692, 1.000000000000000000),
 ( 1.000000000000000000, 0.6746439590912666207, 1.000000000000000000),
 ( 1.000000000000000000, 0.6645663254999827352, 1.000000000000000000),
 ( 1.000000000000000000, 0.6588263891900785207, 1.000000000000000000),
 ( 1.000000000000000000, 0.6558243695371216431, 1.000000000000000000) ) ) 
 REPRESENTATION_ITEM ( '' )  SURFACE ( )  );
#8592=CARTESIAN_POINT ( 'NONE',  ( -8.719536044788691598, 18.00000000000000711, 25.00000000000000000 ) ) ;
#8593=DIRECTION ( 'NONE',  ( 0.000000000000000000, -1.000000000000000000, 6.123233995736762338E-17 ) ) ;
#8596=CARTESIAN_POINT ( 'NONE',  ( 0.000000000000000000, 18.00000000000000355, 0.000000000000000000 ) ) ;
#8612=CARTESIAN_POINT ( 'NONE',  ( 27.48361012695778882, 136.6227766016838530, 1.300194169143111589 ) ) ;
#8613=CARTESIAN_POINT ( 'NONE',  ( 16.31902522550215551, 136.8400131045044930, 5.103539400524462977 ) ) ;
#8616=DIRECTION ( 'NONE',  ( -1.000000000000000000, -0.000000000000000000, -0.000000000000000000 ) ) ;
#8618=CARTESIAN_POINT ( 'NONE',  ( -100.0000000000000000, 142.5209969267753820, 19.44444444444445352 ) ) ;
#8619=CARTESIAN_POINT ( 'NONE',  ( 15.45427063382542165, 18.00000000000226663, 13.01057400152831711 ) ) ;
#8626=ORIENTED_EDGE ( 'NONE', *, *, #15550, .F. ) ;
#8629=EDGE_CURVE ( 'NONE', #15706, #7981, #13515, .T. ) ;
#8630=ORIENTED_EDGE ( 'NONE', *, *, #2005, .T. ) ;
#8633=ORIENTED_EDGE ( 'NONE', *, *, #17303, .T. ) ;
#8635=ORIENTED_EDGE ( 'NONE', *, *, #4377, .T. ) ;
#8637=B_SPLINE_CURVE_WITH_KNOTS ( 'NONE', 3,
 ( #8536, #12440, #4381, #7124 ),
 .UNSPECIFIED., .F., .F.,
 ( 4, 4 ),
 ( 0.000000000000000000, 0.005007666328367723664 ),
 .UNSPECIFIED. ) ;
#8641=DIRECTION ( 'NONE',  ( -1.000000000000000000, -0.000000000000000000, -0.000000000000000000 ) ) ;
#8642=CIRCLE ( 'NONE', #16844, 750.0000000000000000 ) ;
#8643=CIRCLE ( 'NONE', #1001, 10.00000000000000178 ) ;
#8644=DIRECTION ( 'NONE',  ( 0.000000000000000000, 1.000000000000000000, 0.000000000000000000 ) ) ;
#8647=ORIENTED_EDGE ( 'NONE', *, *, #16200, .F. ) ;
#8648=CARTESIAN_POINT ( 'NONE',  ( 29.75497873520074421, 141.6230733471410304, 13.74837463607936883 ) ) ;
#8650=DIRECTION ( 'NONE',  ( 0.000000000000000000, 0.000000000000000000, -1.000000000000000000 ) ) ;
#8655=AXIS2_PLACEMENT_3D ( 'NONE', #2780, #12428, #4288 ) ;
#8657=AXIS2_PLACEMENT_3D ( 'NONE', #3752, #17205, #2419 ) ;
#8662=CARTESIAN_POINT ( 'NONE',  ( 25.83188736168996513, 137.9746650487458908, 9.688332914129558660 ) ) ;
#8663=AXIS2_PLACEMENT_3D ( 'NONE', #2495, #3650, #2593 ) ;
#8664=VERTEX_POINT ( 'NONE', #8274 ) ;
#8665=AXIS2_PLACEMENT_3D ( 'NONE', #193, #2769, #2932 ) ;
#8671=PLANE ( 'NONE',  #10137 ) ;
#8673=EDGE_CURVE ( 'NONE', #3629, #6874, #5969, .T. ) ;
#8675=ORIENTED_EDGE ( 'NONE', *, *, #12801, .T. ) ;
#8678=VECTOR ( 'NONE', #5048, 1000.000000000000000 ) ;
#8681=VERTEX_POINT ( 'NONE', #11285 ) ;
#8687=EDGE_LOOP ( 'NONE', ( #5106, #10512, #563, #4610 ) ) ;
#8689=CARTESIAN_POINT ( 'NONE',  ( -26.10410744458347665, 18.00000000000000000, 13.37721135299797304 ) ) ;
#8690=CARTESIAN_POINT ( 'NONE',  ( -43.00000000000000711, 130.0000000000000000, 12.99999999999999822 ) ) ;
#8692=DIRECTION ( 'NONE',  ( 0.000000000000000000, 0.000000000000000000, 1.000000000000000000 ) ) ;
#8697=EDGE_LOOP ( 'NONE', ( #5777, #4613, #16496, #4846 ) ) ;
#8702=ORIENTED_EDGE ( 'NONE', *, *, #364, .T. ) ;
#8706=CARTESIAN_POINT ( 'NONE',  ( 24.60025152864608700, 29.87271304632927027, 7.586598161752979408 ) ) ;
#8707=CARTESIAN_POINT ( 'NONE',  ( 26.57417986947462651, 137.5626638350942699, 8.060801806284990434 ) ) ;
#8708=CIRCLE ( 'NONE', #2192, 2.499999999999998668 ) ;
#8710=DIRECTION ( 'NONE',  ( -1.000000000000000000, -0.000000000000000000, -0.000000000000000000 ) ) ;
#8712=CARTESIAN_POINT ( 'NONE',  ( -77.12399049755265423, 192.5178712342568303, 25.54362227291155207 ) ) ;
#8715=CARTESIAN_POINT ( 'NONE',  ( 19.14963388379466736, 18.00000000000000000, 24.55317681541934149 ) ) ;
#8719=DIRECTION ( 'NONE',  ( -1.000000000000000000, 0.000000000000000000, 0.000000000000000000 ) ) ;
#8720=AXIS2_PLACEMENT_3D ( 'NONE', #11102, #4387, #9776 ) ;
#8722=ORIENTED_EDGE ( 'NONE', *, *, #6232, .T. ) ;
#8723=LINE ( 'NONE', #15181, #7329 ) ;
#8726=ORIENTED_EDGE ( 'NONE', *, *, #14951, .T. ) ;
#8728=ORIENTED_EDGE ( 'NONE', *, *, #7317, .F. ) ;
#8736=EDGE_CURVE ( 'NONE', #1044, #15578, #873, .T. ) ;
#8746=AXIS2_PLACEMENT_3D ( 'NONE', #3208, #16841, #12425 ) ;
#8747=VECTOR ( 'NONE', #4753, 1000.000000000000000 ) ;
#8749=ORIENTED_EDGE ( 'NONE', *, *, #6232, .F. ) ;
#8752=CARTESIAN_POINT ( 'NONE',  ( 10.42241938378121624, 142.2974014187406055, 19.10582184898306224 ) ) ;
#8755=AXIS2_PLACEMENT_3D ( 'NONE', #9172, #11828, #10585 ) ;
#8756=CYLINDRICAL_SURFACE ( 'NONE', #16521, 2.500000000000000444 ) ;
#8758=DIRECTION ( 'NONE',  ( 0.000000000000000000, 0.000000000000000000, -1.000000000000000000 ) ) ;
#8759=CARTESIAN_POINT ( 'NONE',  ( 0.000000000000000000, 0.000000000000000000, 0.000000000000000000 ) ) ;
#8760=CARTESIAN_POINT ( 'NONE',  ( -80.60934097988227620, 201.5868197762109162, 13.82597759728682796 ) ) ;
#8762=ORIENTED_EDGE ( 'NONE', *, *, #15065, .F. ) ;
#8763=ORIENTED_EDGE ( 'NONE', *, *, #2875, .T. ) ;
#8769=DIRECTION ( 'NONE',  ( -1.000000000000000000, 0.000000000000000000, 0.000000000000000000 ) ) ;
#8770=AXIS2_PLACEMENT_3D ( 'NONE', #11763, #10439, #16208 ) ;
#8772=ORIENTED_EDGE ( 'NONE', *, *, #15327, .T. ) ;
#8773=EDGE_CURVE ( 'NONE', #13751, #9170, #315, .T. ) ;
#8774=DIRECTION ( 'NONE',  ( 8.673617379884037937E-17, 0.000000000000000000, -1.000000000000000000 ) ) ;
#8779=VECTOR ( 'NONE', #16257, 1000.000000000000000 ) ;
#8780=CARTESIAN_POINT ( 'NONE',  ( -12.80328004468388770, 17.99999999999770850, 5.290760321145405953 ) ) ;
#8785=ORIENTED_EDGE ( 'NONE', *, *, #9166, .F. ) ;
#8789=CARTESIAN_POINT ( 'NONE',  ( -68.00000000000000000, 204.6227766016838245, 0.000000000000000000 ) ) ;
#8790=VERTEX_POINT ( 'NONE', #3051 ) ;
#8792=CIRCLE ( 'NONE', #1157, 2.500000000000000000 ) ;
#8793=CARTESIAN_POINT ( 'NONE',  ( 23.77503517897789465, 19.99999999999999645, 22.95135521423388170 ) ) ;
#8794=CARTESIAN_POINT ( 'NONE',  ( 26.46962346220079709, 137.6228726052619606, 8.310907492956932430 ) ) ;
#8797=DIRECTION ( 'NONE',  ( 0.000000000000000000, 0.9938079899999066047, -0.1111111111111111188 ) ) ;
#8798=CARTESIAN_POINT ( 'NONE',  ( -80.97044773050417632, 191.7140209832037954, 26.17909706909632561 ) ) ;
#8801=CARTESIAN_POINT ( 'NONE',  ( -85.00000000000002842, 146.6227766016838245, 35.00200000000000244 ) ) ;
#8805=ORIENTED_EDGE ( 'NONE', *, *, #1544, .F. ) ;
#8810=FACE_OUTER_BOUND ( 'NONE', #2708, .T. ) ;
#8813=VERTEX_POINT ( 'NONE', #14286 ) ;
#8815=ORIENTED_EDGE ( 'NONE', *, *, #13705, .T. ) ;
#8816=DIRECTION ( 'NONE',  ( -0.000000000000000000, -0.000000000000000000, -1.000000000000000000 ) ) ;
#8818=CARTESIAN_POINT ( 'NONE',  ( 196.0000000000000000, 191.6227766016837677, 8.071800142134975431 ) ) ;
#8819=DIRECTION ( 'NONE',  ( -0.000000000000000000, -0.000000000000000000, -1.000000000000000000 ) ) ;
#8820=VERTEX_POINT ( 'NONE', #6058 ) ;
#8823=DIRECTION ( 'NONE',  ( -1.000000000000000000, 0.000000000000000000, 0.000000000000000000 ) ) ;
#8825=CARTESIAN_POINT ( 'NONE',  ( -23.00000000000000000, 120.0000000000000284, 15.00000000000000000 ) ) ;
#8830=ORIENTED_EDGE ( 'NONE', *, *, #13216, .F. ) ;
#8831=CYLINDRICAL_SURFACE ( 'NONE', #4443, 2.500000000000002220 ) ;
#8834=DIRECTION ( 'NONE',  ( -1.000000000000000000, -0.000000000000000000, -0.000000000000000000 ) ) ;
#8835=CARTESIAN_POINT ( 'NONE',  ( -43.00000000000000000, 171.6227766016838245, 0.000000000000000000 ) ) ;
#8845=EDGE_CURVE ( 'NONE', #14384, #7220, #1444, .T. ) ;
#8846=ORIENTED_EDGE ( 'NONE', *, *, #13706, .F. ) ;
#8852=CARTESIAN_POINT ( 'NONE',  ( 17.00000000000000000, 143.0439382767972631, 16.49999999999984013 ) ) ;
#8853=CARTESIAN_POINT ( 'NONE',  ( -15.09627865792072576, 32.41573384469808161, 9.048329374498470301 ) ) ;
#8857=CARTESIAN_POINT ( 'NONE',  ( -27.98221281347037959, 30.00000000000000000, 15.00000000000000000 ) ) ;
#8860=DIRECTION ( 'NONE',  ( -1.000000000000000000, 0.000000000000000000, 0.000000000000000000 ) ) ;
#8862=ORIENTED_EDGE ( 'NONE', *, *, #15803, .F. ) ;
#8863=FACE_OUTER_BOUND ( 'NONE', #17406, .T. ) ;
#8867=FACE_OUTER_BOUND ( 'NONE', #6039, .T. ) ;
#8870=DIRECTION ( 'NONE',  ( 0.000000000000000000, 0.000000000000000000, 1.000000000000000000 ) ) ;
#8872=ORIENTED_EDGE ( 'NONE', *, *, #13599, .T. ) ;
#8875=ORIENTED_EDGE ( 'NONE', *, *, #14562, .T. ) ;
#8879=AXIS2_PLACEMENT_3D ( 'NONE', #2391, #16031, #7785 ) ;
#8884=EDGE_CURVE ( 'NONE', #11165, #12401, #16035, .T. ) ;
#8888=ORIENTED_EDGE ( 'NONE', *, *, #9681, .F. ) ;
#8893=CARTESIAN_POINT ( 'NONE',  ( 22.42543865150203075, 29.85191494357712116, 7.821916630904659939 ) ) ;
#8895=VECTOR ( 'NONE', #1201, 1000.000000000000000 ) ;
#8903=CARTESIAN_POINT ( 'NONE',  ( 33.42689610971938663, 200.2770367110203722, 16.37379161636572178 ) ) ;
#8906=AXIS2_PLACEMENT_3D ( 'NONE', #11144, #4343, #13995 ) ;
#8907=CARTESIAN_POINT ( 'NONE',  ( -5.000000000000000888, 171.6227766016838245, 0.000000000000000000 ) ) ;
#8908=ORIENTED_EDGE ( 'NONE', *, *, #11643, .T. ) ;
#8913=VECTOR ( 'NONE', #10591, 1000.000000000000000 ) ;
#8914=ORIENTED_EDGE ( 'NONE', *, *, #6341, .F. ) ;
#8916=DIRECTION ( 'NONE',  ( 0.000000000000000000, 0.000000000000000000, -1.000000000000000000 ) ) ;
#8922=ADVANCED_FACE ( 'NONE', ( #4350 ), #4619, .T. ) ;
#8924=EDGE_LOOP ( 'NONE', ( #5333, #17211, #17119, #10594 ) ) ;
#8929=CARTESIAN_POINT ( 'NONE',  ( 30.49999999999998224, 9.999999999999998224, 0.000000000000000000 ) ) ;
#8933=CARTESIAN_POINT ( 'NONE',  ( -77.50000000000001421, 196.6227766016838245, 0.000000000000000000 ) ) ;
#8935=CARTESIAN_POINT ( 'NONE',  ( -10.72783954291835151, 17.99999999999999289, 10.92811494094397951 ) ) ;
#8938=CARTESIAN_POINT ( 'NONE',  ( -27.99999999999998224, 10.00000000000000000, 10.00000000000000178 ) ) ;
#8940=EDGE_CURVE ( 'NONE', #5255, #8340, #206, .T. ) ;
#8941=AXIS2_PLACEMENT_3D ( 'NONE', #10812, #5757, #9732 ) ;
#8949=LINE ( 'NONE', #7790, #15818 ) ;
#8950=VECTOR ( 'NONE', #1056, 1000.000000000000000 ) ;
#8954=CARTESIAN_POINT ( 'NONE',  ( 16.61152767523464391, 142.9573811237880534, 16.36000751420521837 ) ) ;
#8955=CARTESIAN_POINT ( 'NONE',  ( 24.52650527911658074, 19.99999999999999645, 8.254754350129561047 ) ) ;
#8957=AXIS2_PLACEMENT_3D ( 'NONE', #529, #13988, #5936 ) ;
#8963=DIRECTION ( 'NONE',  ( -0.000000000000000000, -0.000000000000000000, 1.000000000000000000 ) ) ;
#8968=ORIENTED_EDGE ( 'NONE', *, *, #11370, .T. ) ;
#8974=VERTEX_POINT ( 'NONE', #12765 ) ;
#8976=AXIS2_PLACEMENT_3D ( 'NONE', #2478, #7963, #213 ) ;
#8979=EDGE_CURVE ( 'NONE', #4086, #5381, #2852, .T. ) ;
#8981=EDGE_CURVE ( 'NONE', #13530, #4855, #16077, .T. ) ;
#8984=DIRECTION ( 'NONE',  ( -1.000000000000000000, 0.000000000000000000, 0.000000000000000000 ) ) ;
#8989=LINE ( 'NONE', #15371, #8464 ) ;
#8991=CARTESIAN_POINT ( 'NONE',  ( 24.60077399342406679, 29.87270634359742871, 7.584611049657961068 ) ) ;
#8993=CARTESIAN_POINT ( 'NONE',  ( -725.0000000000000000, 19.99999999999995737, 4.999999999999999112 ) ) ;
#8997=ORIENTED_EDGE ( 'NONE', *, *, #12482, .F. ) ;
#9001=ORIENTED_EDGE ( 'NONE', *, *, #14791, .F. ) ;
#9006=ORIENTED_EDGE ( 'NONE', *, *, #5051, .F. ) ;
#9007=DIRECTION ( 'NONE',  ( -1.000000000000000000, -0.000000000000000000, -0.000000000000000000 ) ) ;
#9008=AXIS2_PLACEMENT_3D ( 'NONE', #2106, #7507, #13008 ) ;
#9023=AXIS2_PLACEMENT_3D ( 'NONE', #10147, #7324, #4666 ) ;
#9027=DIRECTION ( 'NONE',  ( 0.000000000000000000, 1.000000000000000000, 0.000000000000000000 ) ) ;
#9028=CIRCLE ( 'NONE', #10440, 20.00000000000000355 ) ;
#9030=FACE_OUTER_BOUND ( 'NONE', #96, .T. ) ;
#9032=CARTESIAN_POINT ( 'NONE',  ( -25.16839285024616402, 18.00000000000000000, 15.12082343620105540 ) ) ;
#9037=CIRCLE ( 'NONE', #9608, 10.00000000000000000 ) ;
#9040=AXIS2_PLACEMENT_3D ( 'NONE', #9380, #3724, #9027 ) ;
#9041=DIRECTION ( 'NONE',  ( 0.000000000000000000, -1.000000000000000000, 0.000000000000000000 ) ) ;
#9043=CARTESIAN_POINT ( 'NONE',  ( 34.93420767853316988, 20.00000000000000000, 4.999999999999999112 ) ) ;
#9044=CARTESIAN_POINT ( 'NONE',  ( 7.290380404777190293, 133.8591131982526008, 12.94327073059132971 ) ) ;
#9045=EDGE_CURVE ( 'NONE', #570, #16427, #8792, .T. ) ;
#9046=EDGE_CURVE ( 'NONE', #17091, #3368, #6866, .T. ) ;
#9047=CARTESIAN_POINT ( 'NONE',  ( 34.26467700469002864, 19.99999999999999645, 10.17319632352553427 ) ) ;
#9050=VECTOR ( 'NONE', #15372, 1000.000000000000000 ) ;
#9051=ORIENTED_EDGE ( 'NONE', *, *, #4252, .F. ) ;
#9056=ORIENTED_EDGE ( 'NONE', *, *, #364, .F. ) ;
#9068=CARTESIAN_POINT ( 'NONE',  ( -14.96200682865387854, 32.37632742624003157, 9.274234733431431010 ) ) ;
#9069=CARTESIAN_POINT ( 'NONE',  ( -27.99999999999998224, 10.00000000000000000, 0.000000000000000000 ) ) ;
#9072=CARTESIAN_POINT ( 'NONE',  ( 13.66341101665266677, 138.6227766016838245, 1.000341871676679184E-14 ) ) ;
#9077=CARTESIAN_POINT ( 'NONE',  ( 30.81698523721487604, 18.00000000000000000, 17.17210857557096659 ) ) ;
#9080=DIRECTION ( 'NONE',  ( -1.000000000000000000, 0.000000000000000000, 0.000000000000000000 ) ) ;
#9081=EDGE_CURVE ( 'NONE', #8664, #14798, #3427, .T. ) ;
#9082=AXIS2_PLACEMENT_3D ( 'NONE', #17374, #10647, #15243 ) ;
#9083=CARTESIAN_POINT ( 'NONE',  ( 34.99999999999999289, 197.2379877313571797, 20.82664773619436360 ) ) ;
#9086=DIRECTION ( 'NONE',  ( 0.000000000000000000, 0.000000000000000000, -1.000000000000000000 ) ) ;
#9087=ORIENTED_EDGE ( 'NONE', *, *, #8736, .T. ) ;
#9094=DIRECTION ( 'NONE',  ( 0.000000000000000000, 0.000000000000000000, -1.000000000000000000 ) ) ;
#9095=CARTESIAN_POINT ( 'NONE',  ( 6.134011831684049731, 144.1839557653416080, 18.33333333333335702 ) ) ;
#9098=ORIENTED_EDGE ( 'NONE', *, *, #11645, .F. ) ;
#9114=DIRECTION ( 'NONE',  ( -1.000000000000000000, -0.000000000000000000, -0.000000000000000000 ) ) ;
#9116=CARTESIAN_POINT ( 'NONE',  ( -8.509631953695096840, 18.00000000000455103, 12.55445085332768151 ) ) ;
#9119=ORIENTED_EDGE ( 'NONE', *, *, #15904, .T. ) ;
#9120=FACE_OUTER_BOUND ( 'NONE', #6013, .T. ) ;
#9125=ORIENTED_EDGE ( 'NONE', *, *, #14371, .T. ) ;
#9126=DIRECTION ( 'NONE',  ( -1.000000000000000000, 0.000000000000000000, 0.000000000000000000 ) ) ;
#9127=CARTESIAN_POINT ( 'NONE',  ( 15.26338903195270547, 125.9505563168691111, 6.751637631526196337 ) ) ;
#9135=ORIENTED_EDGE ( 'NONE', *, *, #9747, .T. ) ;
#9138=EDGE_CURVE ( 'NONE', #16166, #7981, #6828, .T. ) ;
#9140=ORIENTED_EDGE ( 'NONE', *, *, #14669, .T. ) ;
#9143=ORIENTED_EDGE ( 'NONE', *, *, #9927, .T. ) ;
#9144=ORIENTED_EDGE ( 'NONE', *, *, #11523, .T. ) ;
#9148=ORIENTED_EDGE ( 'NONE', *, *, #2990, .F. ) ;
#9150=FACE_BOUND ( 'NONE', #163, .T. ) ;
#9151=CARTESIAN_POINT ( 'NONE',  ( -8.730345434444062747, 30.30576128541687453, 14.94291915632153334 ) ) ;
#9152=( BOUNDED_SURFACE ( )  B_SPLINE_SURFACE ( 3, 2, ( 
 ( #3740, #2401, #14625 ),
 ( #17365, #10637, #16045 ),
 ( #13118, #13209, #3922 ),
 ( #2595, #14453, #7982 ),
 ( #13383, #12054, #5424 ),
 ( #17462, #5334, #1251 ),
 ( #6659, #10729, #16143 ),
 ( #4017, #14799, #8061 ),
 ( #13475, #1350, #6753 ),
 ( #12150, #21, #10814 ),
 ( #6386, #2319, #17189 ),
 ( #5064, #10460, #6909 ),
 ( #8317, #3107, #5848 ),
 ( #2926, #5503, #276 ),
 ( #9651, #4178, #15133 ),
 ( #4442, #2847, #12230 ),
 ( #187, #1697, #4269 ),
 ( #1779, #439, #13832 ),
 ( #13917, #2764, #15049 ),
 ( #16662, #12309, #14970 ),
 ( #7007, #11244, #16404 ),
 ( #1515, #5590, #9827 ),
 ( #10981, #9471, #8154 ),
 ( #359, #13731, #13568 ) ),
 .UNSPECIFIED., .F., .F., .F. ) 
 B_SPLINE_SURFACE_WITH_KNOTS ( ( 4, 2, 2, 2, 2, 2, 2, 2, 2, 2, 2, 4 ),
 ( 3, 3 ),
 ( 0.01427588378380419132, 0.01824401167166925936, 0.02022807561560179684, 0.02221213955953433086, 0.02618026744739940237, 0.02816433139133193639, 0.03014839533526447041, 0.03411652322312953844, 0.03610058716706207593, 0.03808465111099461342, 0.04205277899885968146, 0.04602090688672474950 ),
 ( 0.000000000000000000, 1.000000000000000000 ),
 .UNSPECIFIED. ) 
 GEOMETRIC_REPRESENTATION_ITEM ( )  RATIONAL_B_SPLINE_SURFACE ( (
 ( 1.000000000000000000, 0.7071067811865476838, 1.000000000000000000),
 ( 1.000000000000000000, 0.7013659285814082267, 1.000000000000000000),
 ( 1.000000000000000000, 0.6957352470443716186, 1.000000000000000000),
 ( 1.000000000000000000, 0.6874449304735253952, 1.000000000000000000),
 ( 1.000000000000000000, 0.6847075230359779274, 1.000000000000000000),
 ( 1.000000000000000000, 0.6792848743381553200, 1.000000000000000000),
 ( 1.000000000000000000, 0.6765866164121365767, 1.000000000000000000),
 ( 1.000000000000000000, 0.6687223666254397125, 1.000000000000000000),
 ( 1.000000000000000000, 0.6637534122518267132, 1.000000000000000000),
 ( 1.000000000000000000, 0.6567012635110727192, 1.000000000000000000),
 ( 1.000000000000000000, 0.6544178910915308123, 1.000000000000000000),
 ( 1.000000000000000000, 0.6499901663949341213, 1.000000000000000000),
 ( 1.000000000000000000, 0.6478648508491323676, 1.000000000000000000),
 ( 1.000000000000000000, 0.6418284244073564349, 1.000000000000000000),
 ( 1.000000000000000000, 0.6382188548936990058, 1.000000000000000000),
 ( 1.000000000000000000, 0.6334349500989927551, 1.000000000000000000),
 ( 1.000000000000000000, 0.6319385063094495880, 1.000000000000000000),
 ( 1.000000000000000000, 0.6292162870119188955, 1.000000000000000000),
 ( 1.000000000000000000, 0.6279881568154176419, 1.000000000000000000),
 ( 1.000000000000000000, 0.6246939197237179053, 1.000000000000000000),
 ( 1.000000000000000000, 0.6230139244305938906, 1.000000000000000000),
 ( 1.000000000000000000, 0.6207349535630983794, 1.000000000000000000),
 ( 1.000000000000000000, 0.6201739322037901347, 1.000000000000000000),
 ( 1.000000000000000000, 0.6201736729460421982, 1.000000000000000000) ) ) 
 REPRESENTATION_ITEM ( '' )  SURFACE ( )  );
#9154=CARTESIAN_POINT ( 'NONE',  ( 21.54590827305403877, 18.00000000000000000, 9.735228713654757726 ) ) ;
#9158=PLANE ( 'NONE',  #16895 ) ;
#9159=LINE ( 'NONE', #9662, #4932 ) ;
#9164=CARTESIAN_POINT ( 'NONE',  ( 34.26588824652853305, 18.00000000000000000, 10.16858984204336736 ) ) ;
#9166=EDGE_CURVE ( 'NONE', #4908, #13584, #14122, .T. ) ;
#9168=DIRECTION ( 'NONE',  ( -0.000000000000000000, 0.000000000000000000, -1.000000000000000000 ) ) ;
#9169=CARTESIAN_POINT ( 'NONE',  ( 29.05191969268358321, 201.5373699728807537, 13.93281245758937992 ) ) ;
#9170=VERTEX_POINT ( 'NONE', #8354 ) ;
#9172=CARTESIAN_POINT ( 'NONE',  ( -27.99999999999998224, 10.00000000000000000, 0.000000000000000000 ) ) ;
#9174=ORIENTED_EDGE ( 'NONE', *, *, #17265, .T. ) ;
#9175=CARTESIAN_POINT ( 'NONE',  ( -82.68880486155467224, 142.3932571782017646, 15.32207027268389865 ) ) ;
#9176=VECTOR ( 'NONE', #10883, 1000.000000000000000 ) ;
#9177=DIRECTION ( 'NONE',  ( -0.8571673013836867971, 0.000000000000000000, -0.5150380737757237481 ) ) ;
#9178=FACE_OUTER_BOUND ( 'NONE', #16507, .T. ) ;
#9179=EDGE_CURVE ( 'NONE', #10705, #7796, #9368, .T. ) ;
#9184=FACE_OUTER_BOUND ( 'NONE', #12526, .T. ) ;
#9192=ORIENTED_EDGE ( 'NONE', *, *, #17062, .F. ) ;
#9197=FACE_OUTER_BOUND ( 'NONE', #12851, .T. ) ;
#9205=FACE_OUTER_BOUND ( 'NONE', #3950, .T. ) ;
#9207=DIRECTION ( 'NONE',  ( 1.000000000000000000, 0.000000000000000000, -0.000000000000000000 ) ) ;
#9208=ORIENTED_EDGE ( 'NONE', *, *, #572, .T. ) ;
#9211=EDGE_CURVE ( 'NONE', #8681, #1349, #11618, .T. ) ;
#9213=EDGE_CURVE ( 'NONE', #3385, #5700, #15080, .T. ) ;
#9216=ORIENTED_EDGE ( 'NONE', *, *, #144, .F. ) ;
#9218=CARTESIAN_POINT ( 'NONE',  ( 14.12141184870282196, 138.6801925718470443, 3.743222489502259887 ) ) ;
#9219=ORIENTED_EDGE ( 'NONE', *, *, #14530, .F. ) ;
#9220=CARTESIAN_POINT ( 'NONE',  ( 17.04731744882672828, 19.99999999999885247, 14.80421929169553685 ) ) ;
#9223=AXIS2_PLACEMENT_3D ( 'NONE', #4867, #12571, #11412 ) ;
#9231=CARTESIAN_POINT ( 'NONE',  ( 33.96623626252291928, 149.6716700844112324, 24.64096846353361414 ) ) ;
#9232=EDGE_LOOP ( 'NONE', ( #808, #12771, #6877 ) ) ;
#9234=LINE ( 'NONE', #14546, #5263 ) ;
#9236=VERTEX_POINT ( 'NONE', #11099 ) ;
#9238=VERTEX_POINT ( 'NONE', #1989 ) ;
#9242=ORIENTED_EDGE ( 'NONE', *, *, #1103, .F. ) ;
#9245=CARTESIAN_POINT ( 'NONE',  ( -10.05738114656989346, 30.87167111307020306, 12.65386873594253103 ) ) ;
#9246=CARTESIAN_POINT ( 'NONE',  ( -17.86279820300995169, 32.23061541110773476, 7.751589558536285729 ) ) ;
#9249=CARTESIAN_POINT ( 'NONE',  ( -82.57145418340599008, 150.9146311475675759, 25.69413650784049707 ) ) ;
#9250=VERTEX_POINT ( 'NONE', #7293 ) ;
#9256=CARTESIAN_POINT ( 'NONE',  ( 25.51458778375578973, 18.00000000000000000, 21.98440010584615578 ) ) ;
#9258=ORIENTED_EDGE ( 'NONE', *, *, #8884, .F. ) ;
#9260=CARTESIAN_POINT ( 'NONE',  ( 32.67866620718707082, 200.8588467739806447, 15.30956876290918522 ) ) ;
#9266=CIRCLE ( 'NONE', #9834, 2.500000000000002220 ) ;
#9269=AXIS2_PLACEMENT_3D ( 'NONE', #9545, #2999, #12387 ) ;
#9272=CARTESIAN_POINT ( 'NONE',  ( -10.03891356649071653, 19.99999999999999289, 24.87483525495232328 ) ) ;
#9273=ORIENTED_EDGE ( 'NONE', *, *, #10741, .T. ) ;
#9276=DIRECTION ( 'NONE',  ( -1.000000000000000000, 0.000000000000000000, 0.000000000000000000 ) ) ;
#9278=CIRCLE ( 'NONE', #3925, 2.500000000000002220 ) ;
#9280=ORIENTED_EDGE ( 'NONE', *, *, #9973, .T. ) ;
#9285=VERTEX_POINT ( 'NONE', #16512 ) ;
#9289=CIRCLE ( 'NONE', #16664, 2.500000000000000000 ) ;
#9290=EDGE_CURVE ( 'NONE', #10702, #11548, #8637, .T. ) ;
#9291=VECTOR ( 'NONE', #4051, 1000.000000000000000 ) ;
#9292=DIRECTION ( 'NONE',  ( 0.000000000000000000, 0.000000000000000000, -1.000000000000000000 ) ) ;
#9293=CIRCLE ( 'NONE', #12703, 35.00000000000000000 ) ;
#9294=CARTESIAN_POINT ( 'NONE',  ( -45.00000000000003553, 120.0000000000000142, 4.999999999999999112 ) ) ;
#9297=DIRECTION ( 'NONE',  ( -1.000000000000000000, -0.000000000000000000, -0.000000000000000000 ) ) ;
#9298=DIRECTION ( 'NONE',  ( -0.000000000000000000, -0.000000000000000000, -1.000000000000000000 ) ) ;
#9300=ORIENTED_EDGE ( 'NONE', *, *, #7565, .F. ) ;
#9301=CARTESIAN_POINT ( 'NONE',  ( 6.134011831684053284, 134.2062027339443944, 25.00000000000000000 ) ) ;
#9308=DIRECTION ( 'NONE',  ( -0.000000000000000000, -0.000000000000000000, -1.000000000000000000 ) ) ;
#9310=CARTESIAN_POINT ( 'NONE',  ( 13.90347339350139677, 138.7488974902626069, 3.510692536284492959 ) ) ;
#9319=AXIS2_PLACEMENT_3D ( 'NONE', #10798, #967, #17346 ) ;
#9321=CARTESIAN_POINT ( 'NONE',  ( 34.53513972622751993, 148.7497411309094275, 23.78985390322973359 ) ) ;
#9322=VERTEX_POINT ( 'NONE', #7202 ) ;
#9325=ORIENTED_EDGE ( 'NONE', *, *, #3253, .F. ) ;
#9328=EDGE_CURVE ( 'NONE', #5404, #6861, #15436, .T. ) ;
#9329=VECTOR ( 'NONE', #1657, 1000.000000000000000 ) ;
#9331=CARTESIAN_POINT ( 'NONE',  ( -80.00000000000001421, 196.6227766016838245, 35.00200000000000244 ) ) ;
#9333=ADVANCED_FACE ( 'NONE', ( #5787 ), #17283, .T. ) ;
#9341=CARTESIAN_POINT ( 'NONE',  ( 49.99999999999998579, 159.6227766016838814, 5.571800142134975431 ) ) ;
#9342=CYLINDRICAL_SURFACE ( 'NONE', #15409, 33.00000000000000000 ) ;
#9344=DIRECTION ( 'NONE',  ( -1.000000000000000000, -0.000000000000000000, -0.000000000000000000 ) ) ;
#9347=CARTESIAN_POINT ( 'NONE',  ( 12.53348921593948972, 131.0729685438566605, 13.11561688552428784 ) ) ;
#9350=LINE ( 'NONE', #16180, #3364 ) ;
#9352=CARTESIAN_POINT ( 'NONE',  ( 48.00000000000000711, 151.6227766016839098, 8.071800142134973655 ) ) ;
#9354=DIRECTION ( 'NONE',  ( -1.156482317317868274E-16, 1.000000000000000000, -0.000000000000000000 ) ) ;
#9356=ORIENTED_EDGE ( 'NONE', *, *, #3253, .T. ) ;
#9360=CARTESIAN_POINT ( 'NONE',  ( -75.00000000000002842, 146.6227766016838245, 21.54065922853802562 ) ) ;
#9365=FACE_OUTER_BOUND ( 'NONE', #12442, .T. ) ;
#9367=FACE_OUTER_BOUND ( 'NONE', #10179, .T. ) ;
#9368=CIRCLE ( 'NONE', #2597, 2.500000000000000444 ) ;
#9370=EDGE_CURVE ( 'NONE', #11161, #16720, #7394, .T. ) ;
#9372=EDGE_CURVE ( 'NONE', #12169, #817, #887, .T. ) ;
#9375=ORIENTED_EDGE ( 'NONE', *, *, #14637, .T. ) ;
#9378=EDGE_LOOP ( 'NONE', ( #10295, #15333, #17499, #12104 ) ) ;
#9380=CARTESIAN_POINT ( 'NONE',  ( 48.00000000000000711, 187.6227766016837961, 12.50000337241049309 ) ) ;
#9383=CARTESIAN_POINT ( 'NONE',  ( -95.00000000000000000, 201.6227766016838245, 1.836970198721029589E-15 ) ) ;
#9389=ORIENTED_EDGE ( 'NONE', *, *, #2107, .F. ) ;
#9391=EDGE_CURVE ( 'NONE', #2665, #6230, #14185, .T. ) ;
#9393=DIRECTION ( 'NONE',  ( -2.312964634635742464E-16, 0.000000000000000000, 1.000000000000000000 ) ) ;
#9397=CARTESIAN_POINT ( 'NONE',  ( 21.84350049701177809, 141.4638053371992328, 13.40107808329819150 ) ) ;
#9398=ORIENTED_EDGE ( 'NONE', *, *, #3100, .F. ) ;
#9399=CARTESIAN_POINT ( 'NONE',  ( 18.45742352454476887, 29.95282391178955095, 14.36414658362611974 ) ) ;
#9406=ORIENTED_EDGE ( 'NONE', *, *, #3975, .T. ) ;
#9407=CARTESIAN_POINT ( 'NONE',  ( 26.33723719015080889, 150.0417915422717101, 24.96744664354709897 ) ) ;
#9408=ORIENTED_EDGE ( 'NONE', *, *, #3162, .T. ) ;
#9411=EDGE_LOOP ( 'NONE', ( #14619, #11595, #7105, #4631 ) ) ;
#9413=ORIENTED_EDGE ( 'NONE', *, *, #3078, .F. ) ;
#9417=CARTESIAN_POINT ( 'NONE',  ( 48.00000000000000711, 159.6227766016838814, 5.571800142134975431 ) ) ;
#9418=DIRECTION ( 'NONE',  ( 1.000000000000000000, 0.000000000000000000, 0.000000000000000000 ) ) ;
#9421=CARTESIAN_POINT ( 'NONE',  ( -75.10310273927775881, 147.6679082027615948, 22.70058015389365735 ) ) ;
#9425=DIRECTION ( 'NONE',  ( -1.000000000000000000, -0.000000000000000000, -0.000000000000000000 ) ) ;
#9426=CARTESIAN_POINT ( 'NONE',  ( 20.13757169487763576, 18.00000000000000000, 24.32197800972832624 ) ) ;
#9428=DIRECTION ( 'NONE',  ( -1.000000000000000000, 0.000000000000000000, 0.000000000000000000 ) ) ;
#9429=ADVANCED_FACE ( 'NONE', ( #7457 ), #745, .T. ) ;
#9436=CARTESIAN_POINT ( 'NONE',  ( 48.00000000000000711, 146.6227766016838245, 4.592425496802573578E-15 ) ) ;
#9439=ORIENTED_EDGE ( 'NONE', *, *, #1193, .F. ) ;
#9440=DIRECTION ( 'NONE',  ( 0.000000000000000000, 0.000000000000000000, -1.000000000000000000 ) ) ;
#9452=FACE_OUTER_BOUND ( 'NONE', #4230, .T. ) ;
#9458=CIRCLE ( 'NONE', #4398, 750.0000000000001137 ) ;
#9461=CARTESIAN_POINT ( 'NONE',  ( -5.000000000000004441, 171.6227766016838245, 0.000000000000000000 ) ) ;
#9463=DIRECTION ( 'NONE',  ( -1.000000000000000000, -0.000000000000000000, -0.000000000000000000 ) ) ;
#9471=CARTESIAN_POINT ( 'NONE',  ( -15.33310217281858634, 19.99999999999769784, 5.462585411291380311 ) ) ;
#9472=CARTESIAN_POINT ( 'NONE',  ( 25.02538947966649729, 140.2588485512474392, 10.30263013689336304 ) ) ;
#9474=VERTEX_POINT ( 'NONE', #13484 ) ;
#9475=CIRCLE ( 'NONE', #10331, 248.0000000000000000 ) ;
#9476=CARTESIAN_POINT ( 'NONE',  ( 17.20984524040877872, 19.99999999999999645, 14.76996962246643896 ) ) ;
#9483=DIRECTION ( 'NONE',  ( -1.000000000000000000, -0.000000000000000000, -0.000000000000000000 ) ) ;
#9485=DIRECTION ( 'NONE',  ( 0.000000000000000000, 1.000000000000000000, 0.000000000000000000 ) ) ;
#9486=DIRECTION ( 'NONE',  ( -0.000000000000000000, -0.000000000000000000, -1.000000000000000000 ) ) ;
#9487=AXIS2_PLACEMENT_3D ( 'NONE', #14823, #13507, #10838 ) ;
#9488=ORIENTED_EDGE ( 'NONE', *, *, #10638, .T. ) ;
#9489=DIRECTION ( 'NONE',  ( -1.000000000000000000, 0.000000000000000000, 0.000000000000000000 ) ) ;
#9490=CIRCLE ( 'NONE', #747, 12.00000000000000000 ) ;
#9493=LINE ( 'NONE', #1529, #9787 ) ;
#9494=CARTESIAN_POINT ( 'NONE',  ( -100.0000000000000000, 171.6227766016838245, 0.000000000000000000 ) ) ;
#9495=ORIENTED_EDGE ( 'NONE', *, *, #6514, .F. ) ;
#9496=EDGE_LOOP ( 'NONE', ( #6240, #14112, #10036 ) ) ;
#9497=CARTESIAN_POINT ( 'NONE',  ( 7.535032041485008492, 142.5209969262061804, 19.44444444359253410 ) ) ;
#9500=ORIENTED_EDGE ( 'NONE', *, *, #6341, .T. ) ;
#9507=CARTESIAN_POINT ( 'NONE',  ( -75.00000000000004263, 146.8780590376976249, 21.83693896782702026 ) ) ;
#9508=ORIENTED_EDGE ( 'NONE', *, *, #11007, .F. ) ;
#9516=AXIS2_PLACEMENT_3D ( 'NONE', #14611, #1066, #4821 ) ;
#9519=LINE ( 'NONE', #1480, #1980 ) ;
#9528=AXIS2_PLACEMENT_3D ( 'NONE', #3184, #11328, #618 ) ;
#9530=AXIS2_PLACEMENT_3D ( 'NONE', #5726, #7221, #6068 ) ;
#9536=CARTESIAN_POINT ( 'NONE',  ( -147.9615242270661213, 171.6227766016838245, 0.000000000000000000 ) ) ;
#9539=ORIENTED_EDGE ( 'NONE', *, *, #34, .F. ) ;
#9540=FACE_BOUND ( 'NONE', #7020, .T. ) ;
#9543=FILL_AREA_STYLE ('',( #343 ) ) ;
#9545=CARTESIAN_POINT ( 'NONE',  ( -100.0000000000000000, 171.6227766016838245, 0.000000000000000000 ) ) ;
#9546=CARTESIAN_POINT ( 'NONE',  ( 25.93409701014191882, 193.6946896392258282, 24.53450862945287980 ) ) ;
#9552=CARTESIAN_POINT ( 'NONE',  ( 17.51497691750854813, 29.94811823131043127, 12.57651788136221072 ) ) ;
#9553=AXIS2_PLACEMENT_3D ( 'NONE', #15786, #10376, #14640 ) ;
#9555=CIRCLE ( 'NONE', #13810, 2.499999999999998668 ) ;
#9560=CARTESIAN_POINT ( 'NONE',  ( 49.99999999999998579, 159.6227766016838814, 5.571800142134975431 ) ) ;
#9564=DIRECTION ( 'NONE',  ( 0.000000000000000000, -0.4999999999999952816, -0.8660254037844413721 ) ) ;
#9566=ORIENTED_EDGE ( 'NONE', *, *, #6492, .F. ) ;
#9567=VECTOR ( 'NONE', #17184, 1000.000000000000000 ) ;
#9570=ORIENTED_EDGE ( 'NONE', *, *, #5123, .T. ) ;
#9577=CARTESIAN_POINT ( 'NONE',  ( 32.06470260736958267, 151.1803749979462737, 25.90597399044990823 ) ) ;
#9578=CIRCLE ( 'NONE', #7891, 12.00000000000000000 ) ;
#9580=DIRECTION ( 'NONE',  ( -0.000000000000000000, -0.000000000000000000, -1.000000000000000000 ) ) ;
#9582=DIRECTION ( 'NONE',  ( 0.000000000000000000, 0.000000000000000000, -1.000000000000000000 ) ) ;
#9584=EDGE_CURVE ( 'NONE', #7981, #16166, #13051, .T. ) ;
#9589=ORIENTED_EDGE ( 'NONE', *, *, #11641, .T. ) ;
#9591=CARTESIAN_POINT ( 'NONE',  ( 8.038468667238035437, 139.4170824625289242, 14.76281475457819070 ) ) ;
#9594=VECTOR ( 'NONE', #6569, 1000.000000000000000 ) ;
#9597=DIRECTION ( 'NONE',  ( 1.000000000000000000, 1.156482317317868274E-16, -0.000000000000000000 ) ) ;
#9598=CARTESIAN_POINT ( 'NONE',  ( -725.0000000000000000, 19.99999999999995737, 4.999999999999999112 ) ) ;
#9600=CARTESIAN_POINT ( 'NONE',  ( -82.41118593285520433, 151.0069623973649868, 25.76819119792229529 ) ) ;
#9603=CARTESIAN_POINT ( 'NONE',  ( -82.50000000000001421, 196.6227766016838245, 0.000000000000000000 ) ) ;
#9604=CARTESIAN_POINT ( 'NONE',  ( 17.00000000000000000, 171.6227766016838245, 20.00000000000000355 ) ) ;
#9605=DIRECTION ( 'NONE',  ( 0.000000000000000000, 0.000000000000000000, -1.000000000000000000 ) ) ;
#9606=CARTESIAN_POINT ( 'NONE',  ( -95.00000000000000000, 171.6227766016838245, 27.69059892324149530 ) ) ;
#9608=AXIS2_PLACEMENT_3D ( 'NONE', #1593, #6994, #8306 ) ;
#9609=VERTEX_POINT ( 'NONE', #4190 ) ;
#9610=AXIS2_PLACEMENT_3D ( 'NONE', #5216, #14515, #16023 ) ;
#9616=DIRECTION ( 'NONE',  ( -1.000000000000000000, -6.938893903907228378E-16, 0.000000000000000000 ) ) ;
#9617=DIRECTION ( 'NONE',  ( 0.000000000000000000, 0.000000000000000000, 1.000000000000000000 ) ) ;
#9621=EDGE_LOOP ( 'NONE', ( #9001, #7231 ) ) ;
#9629=PLANE ( 'NONE',  #8386 ) ;
#9630=DIRECTION ( 'NONE',  ( 1.337133840571206485E-16, 0.000000000000000000, -1.000000000000000000 ) ) ;
#9631=ORIENTED_EDGE ( 'NONE', *, *, #11933, .F. ) ;
#9634=DIRECTION ( 'NONE',  ( -0.000000000000000000, -0.000000000000000000, 1.000000000000000000 ) ) ;
#9635=CARTESIAN_POINT ( 'NONE',  ( 30.20512376220668926, 191.6231342001797202, 26.24853702829030766 ) ) ;
#9641=ADVANCED_FACE ( 'NONE', ( #13313 ), #1178, .F. ) ;
#9647=ADVANCED_FACE ( 'NONE', ( #12584 ), #449, .F. ) ;
#9648=DIRECTION ( 'NONE',  ( -0.000000000000000000, -0.000000000000000000, -1.000000000000000000 ) ) ;
#9651=CARTESIAN_POINT ( 'NONE',  ( -23.66837786580496328, 19.99999999999999645, 17.32703391567687135 ) ) ;
#9654=ORIENTED_EDGE ( 'NONE', *, *, #2970, .F. ) ;
#9659=CARTESIAN_POINT ( 'NONE',  ( 17.00000000000000000, 191.6227766016837961, -1.224646799147353454E-15 ) ) ;
#9660=EDGE_LOOP ( 'NONE', ( #4264, #13055, #9143, #5629 ) ) ;
#9661=DIRECTION ( 'NONE',  ( 0.000000000000000000, -8.673617379884035472E-17, 1.000000000000000000 ) ) ;
#9662=CARTESIAN_POINT ( 'NONE',  ( -45.00000000000000000, 122.0000000000000142, 4.999999999999999112 ) ) ;
#9668=DIRECTION ( 'NONE',  ( 0.000000000000000000, -1.000000000000000000, -0.000000000000000000 ) ) ;
#9670=EDGE_LOOP ( 'NONE', ( #11220, #5037, #3344, #4498, #13303 ) ) ;
#9673=CARTESIAN_POINT ( 'NONE',  ( 6.134011831684059501, 142.5209969267753820, 19.44444444444444642 ) ) ;
#9676=CARTESIAN_POINT ( 'NONE',  ( -45.00000000000000000, 142.5209969267753820, 19.44444444444444997 ) ) ;
#9678=DIRECTION ( 'NONE',  ( -1.000000000000000000, 0.000000000000000000, 0.000000000000000000 ) ) ;
#9681=EDGE_CURVE ( 'NONE', #2477, #3947, #288, .T. ) ;
#9682=CARTESIAN_POINT ( 'NONE',  ( 19.87492423018547427, 17.99999999999543121, 11.43634947295695703 ) ) ;
#9684=ORIENTED_EDGE ( 'NONE', *, *, #1233, .F. ) ;
#9687=CARTESIAN_POINT ( 'NONE',  ( -100.0000000000000000, 171.6227766016838245, 0.000000000000000000 ) ) ;
#9690=ORIENTED_EDGE ( 'NONE', *, *, #1859, .F. ) ;
#9694=CYLINDRICAL_SURFACE ( 'NONE', #9530, 2.500000000000000444 ) ;
#9695=VERTEX_POINT ( 'NONE', #8328 ) ;
#9697=LINE ( 'NONE', #13693, #3691 ) ;
#9703=ADVANCED_FACE ( 'NONE', ( #4542 ), #5690, .T. ) ;
#9705=EDGE_CURVE ( 'NONE', #216, #6230, #15330, .T. ) ;
#9708=DIRECTION ( 'NONE',  ( -0.000000000000000000, -0.000000000000000000, -1.000000000000000000 ) ) ;
#9714=FACE_BOUND ( 'NONE', #2117, .T. ) ;
#9717=( NAMED_UNIT ( * ) SI_UNIT ( $, .STERADIAN. ) SOLID_ANGLE_UNIT ( ) );
#9719=EDGE_CURVE ( 'NONE', #12351, #5017, #15143, .T. ) ;
#9720=CARTESIAN_POINT ( 'NONE',  ( 196.0000000000000000, 179.6227766016838245, 12.50000337241049309 ) ) ;
#9721=CARTESIAN_POINT ( 'NONE',  ( 28.46817412490414512, 191.8593874686152674, 26.06696055488264108 ) ) ;
#9725=CARTESIAN_POINT ( 'NONE',  ( 18.00561851734427421, 29.93835620586352064, 12.40035566057732375 ) ) ;
#9726=CARTESIAN_POINT ( 'NONE',  ( -83.43806183198967119, 200.2660383695261714, 16.39286986631257292 ) ) ;
#9728=VECTOR ( 'NONE', #15217, 1000.000000000000000 ) ;
#9730=VERTEX_POINT ( 'NONE', #12501 ) ;
#9731=CARTESIAN_POINT ( 'NONE',  ( -75.00000000000000000, 196.6227766016838245, 0.000000000000000000 ) ) ;
#9732=DIRECTION ( 'NONE',  ( 0.000000000000000000, 0.000000000000000000, 1.000000000000000000 ) ) ;
#9733=VERTEX_POINT ( 'NONE', #10992 ) ;
#9736=VERTEX_POINT ( 'NONE', #9659 ) ;
#9739=ADVANCED_FACE ( 'NONE', ( #4450 ), #8424, .F. ) ;
#9741=DIRECTION ( 'NONE',  ( -1.000000000000000000, 0.000000000000000000, 0.000000000000000000 ) ) ;
#9742=CIRCLE ( 'NONE', #5794, 12.00000000000000000 ) ;
#9747=EDGE_CURVE ( 'NONE', #15915, #11290, #6918, .T. ) ;
#9748=ADVANCED_FACE ( 'NONE', ( #3117 ), #1366, .T. ) ;
#9751=DIRECTION ( 'NONE',  ( 0.000000000000000000, 0.000000000000000000, -1.000000000000000000 ) ) ;
#9757=CARTESIAN_POINT ( 'NONE',  ( 25.00000000000000711, 146.6227766016838245, 35.00200000000000244 ) ) ;
#9759=EDGE_LOOP ( 'NONE', ( #15463, #2464 ) ) ;
#9761=DIRECTION ( 'NONE',  ( 1.000000000000000000, 0.000000000000000000, 0.000000000000000000 ) ) ;
#9762=AXIS2_PLACEMENT_3D ( 'NONE', #4090, #6748, #12048 ) ;
#9763=CARTESIAN_POINT ( 'NONE',  ( 15.96677753506825681, 136.6227766017765930, 1.239574023933039948 ) ) ;
#9764=CARTESIAN_POINT ( 'NONE',  ( 26.76721132277178228, 137.4464968366854407, 7.553125767360616472 ) ) ;
#9768=DIRECTION ( 'NONE',  ( -1.000000000000000000, 0.000000000000000000, 0.000000000000000000 ) ) ;
#9771=CARTESIAN_POINT ( 'NONE',  ( 17.13110662433428288, 29.95577564710725227, 12.69327266642979168 ) ) ;
#9773=LINE ( 'NONE', #69, #4085 ) ;
#9776=DIRECTION ( 'NONE',  ( -1.000000000000000000, 0.000000000000000000, 0.000000000000000000 ) ) ;
#9781=EDGE_LOOP ( 'NONE', ( #9830, #5763, #7645, #16141, #17144, #3647, #4123 ) ) ;
#9784=AXIS2_PLACEMENT_3D ( 'NONE', #6051, #8616, #3482 ) ;
#9785=DIRECTION ( 'NONE',  ( -1.000000000000000000, -0.000000000000000000, -0.000000000000000000 ) ) ;
#9787=VECTOR ( 'NONE', #9582, 1000.000000000000000 ) ;
#9792=CARTESIAN_POINT ( 'NONE',  ( -22.99999999999999289, 90.00000000000000000, 4.999999999999999112 ) ) ;
#9795=VECTOR ( 'NONE', #712, 1000.000000000000000 ) ;
#9796=AXIS2_PLACEMENT_3D ( 'NONE', #12935, #1154, #7781 ) ;
#9801=CARTESIAN_POINT ( 'NONE',  ( 196.0000000000000000, 179.6227766016838245, 12.50000337241049309 ) ) ;
#9804=AXIS2_PLACEMENT_3D ( 'NONE', #9895, #11573, #1934 ) ;
#9805=DIRECTION ( 'NONE',  ( -0.000000000000000000, -0.000000000000000000, -1.000000000000000000 ) ) ;
#9808=EDGE_CURVE ( 'NONE', #13439, #735, #4224, .T. ) ;
#9811=ORIENTED_EDGE ( 'NONE', *, *, #13086, .T. ) ;
#9824=AXIS2_PLACEMENT_3D ( 'NONE', #1234, #5405, #16207 ) ;
#9825=FACE_OUTER_BOUND ( 'NONE', #16206, .T. ) ;
#9826=ORIENTED_EDGE ( 'NONE', *, *, #3062, .F. ) ;
#9827=CARTESIAN_POINT ( 'NONE',  ( -18.18164784767110120, 32.29378831700660157, 6.323624269675778287 ) ) ;
#9828=ADVANCED_FACE ( 'NONE', ( #5322 ), #14707, .T. ) ;
#9830=ORIENTED_EDGE ( 'NONE', *, *, #15036, .F. ) ;
#9833=CARTESIAN_POINT ( 'NONE',  ( -19.79962810613639945, 18.00000000000000711, 20.97942696524416206 ) ) ;
#9834=AXIS2_PLACEMENT_3D ( 'NONE', #3573, #2246, #11794 ) ;
#9838=CARTESIAN_POINT ( 'NONE',  ( -68.00000000000000000, 154.3022685259950038, 9.999999999999900524 ) ) ;
#9839=DIRECTION ( 'NONE',  ( -1.000000000000000000, -0.000000000000000000, -0.000000000000000000 ) ) ;
#9847=DIRECTION ( 'NONE',  ( 1.000000000000000000, 0.000000000000000000, 0.000000000000000000 ) ) ;
#9848=AXIS2_PLACEMENT_3D ( 'NONE', #5773, #11082, #4547 ) ;
#9851=CARTESIAN_POINT ( 'NONE',  ( -24.99999999999999645, 120.0000000000000284, 4.999999999999999112 ) ) ;
#9853=CARTESIAN_POINT ( 'NONE',  ( 15.93460003626534238, 136.8193095811534761, 3.708327557688629206 ) ) ;
#9854=CARTESIAN_POINT ( 'NONE',  ( 15.51497662817079082, 137.3737080369936905, 9.118346648348486738 ) ) ;
#9856=CARTESIAN_POINT ( 'NONE',  ( -100.0000000000000000, 143.0439382767972347, 16.49999999999984368 ) ) ;
#9858=CARTESIAN_POINT ( 'NONE',  ( -84.64903570047881942, 194.7608640721562381, 23.53240337055842701 ) ) ;
#9860=CARTESIAN_POINT ( 'NONE',  ( 18.23439605415255471, 29.93382634594462743, 12.29196570735054728 ) ) ;
#9863=CIRCLE ( 'NONE', #12409, 11.99999999999999645 ) ;
#9867=DIRECTION ( 'NONE',  ( -1.000000000000000000, -0.000000000000000000, -0.000000000000000000 ) ) ;
#9870=DIRECTION ( 'NONE',  ( -1.000000000000000000, 0.000000000000000000, 0.000000000000000000 ) ) ;
#9871=ORIENTED_EDGE ( 'NONE', *, *, #15837, .F. ) ;
#9874=EDGE_CURVE ( 'NONE', #12401, #14513, #10710, .T. ) ;
#9875=CARTESIAN_POINT ( 'NONE',  ( 12.56741672263938625, 143.7071609262609400, 17.59902447249972113 ) ) ;
#9880=AXIS2_PLACEMENT_3D ( 'NONE', #872, #13163, #10319 ) ;
#9881=EDGE_CURVE ( 'NONE', #16273, #190, #8053, .T. ) ;
#9885=DIRECTION ( 'NONE',  ( 0.000000000000000000, 0.000000000000000000, -1.000000000000000000 ) ) ;
#9886=CARTESIAN_POINT ( 'NONE',  ( 225.0000000000000000, 89.99999999999997158, 15.00000000000000000 ) ) ;
#9894=ORIENTED_EDGE ( 'NONE', *, *, #1598, .T. ) ;
#9895=CARTESIAN_POINT ( 'NONE',  ( 30.00000000000001066, 146.6227766016838245, 10.00000000000000178 ) ) ;
#9899=SURFACE_STYLE_USAGE ( .BOTH. , #15213 ) ;
#9900=CARTESIAN_POINT ( 'NONE',  ( 26.38776508739448801, 137.6838126476015134, 8.633687169601740763 ) ) ;
#9905=LINE ( 'NONE', #15390, #5293 ) ;
#9908=EDGE_CURVE ( 'NONE', #6775, #11482, #91, .T. ) ;
#9909=DIRECTION ( 'NONE',  ( -1.000000000000000000, -0.000000000000000000, -0.000000000000000000 ) ) ;
#9911=VERTEX_POINT ( 'NONE', #530 ) ;
#9912=AXIS2_PLACEMENT_3D ( 'NONE', #582, #7211, #13682 ) ;
#9918=DIRECTION ( 'NONE',  ( -0.000000000000000000, -0.000000000000000000, -1.000000000000000000 ) ) ;
#9920=EDGE_LOOP ( 'NONE', ( #8805, #16615 ) ) ;
#9922=VECTOR ( 'NONE', #10023, 1000.000000000000000 ) ;
#9926=CARTESIAN_POINT ( 'NONE',  ( -48.00000000000000000, 154.3022685259950038, 9.999999999999900524 ) ) ;
#9927=EDGE_CURVE ( 'NONE', #14513, #4275, #6991, .T. ) ;
#9932=CYLINDRICAL_SURFACE ( 'NONE', #9848, 33.00000000000000000 ) ;
#9933=ORIENTED_EDGE ( 'NONE', *, *, #14528, .F. ) ;
#9939=( BOUNDED_SURFACE ( )  B_SPLINE_SURFACE ( 3, 2, ( 
 ( #17046, #14396, #6250 ),
 ( #7658, #934, #7735 ),
 ( #6323, #11718, #7570 ),
 ( #14479, #13146, #4842 ),
 ( #10230, #17128, #5005 ),
 ( #10570, #10392, #5179 ),
 ( #14561, #15628, #8893 ),
 ( #15894, #1015, #6419 ),
 ( #11811, #17217, #5095 ),
 ( #3764, #9154, #1848 ),
 ( #12981, #2432, #7830 ),
 ( #15978, #13241, #1112 ),
 ( #6512, #3505, #11905 ),
 ( #17311, #3861, #13986 ),
 ( #12652, #9682, #478 ),
 ( #4383, #5882, #4563 ),
 ( #13947, #16440, #1730 ),
 ( #9948, #5626, #1808 ),
 ( #11019, #16514, #9860 ),
 ( #7203, #5714, #1900 ),
 ( #15348, #7294, #387 ),
 ( #11279, #11186, #9771 ),
 ( #15175, #578, #5977 ),
 ( #4300, #3143, #5789 ),
 ( #8715, #12608, #16694 ),
 ( #7041, #15081, #16603 ),
 ( #3046, #8619, #4476 ),
 ( #14123, #12524, #15268 ) ),
 .UNSPECIFIED., .F., .F., .T. ) 
 B_SPLINE_SURFACE_WITH_KNOTS ( ( 4, 2, 2, 2, 2, 2, 2, 2, 2, 2, 2, 2, 2, 4 ),
 ( 3, 3 ),
 ( 0.01342997177288655399, 0.01733910390705692070, 0.01929366997414210666, 0.02124823604122728915, 0.02515736817539765760, 0.02711193424248284356, 0.02906650030956802605, 0.03297563244373839797, 0.03493019851082358046, 0.03688476457790876295, 0.03883933064499394544, 0.03981661367853653322, 0.04079389671207912793, 0.04470302884624949985 ),
 ( 0.000000000000000000, 1.000000000000000000 ),
 .UNSPECIFIED. ) 
 GEOMETRIC_REPRESENTATION_ITEM ( )  RATIONAL_B_SPLINE_SURFACE ( (
 ( 1.000000000000000000, 0.7117435966472906994, 1.000000000000000000),
 ( 1.000000000000000000, 0.7117434842622243352, 1.000000000000000000),
 ( 1.000000000000000000, 0.7117144184577041122, 1.000000000000000000),
 ( 1.000000000000000000, 0.7116285301813174424, 1.000000000000000000),
 ( 1.000000000000000000, 0.7115928256594988843, 1.000000000000000000),
 ( 1.000000000000000000, 0.7115068832447583036, 1.000000000000000000),
 ( 1.000000000000000000, 0.7114564033772057261, 1.000000000000000000),
 ( 1.000000000000000000, 0.7112861117249480447, 1.000000000000000000),
 ( 1.000000000000000000, 0.7111469280185451769, 1.000000000000000000),
 ( 1.000000000000000000, 0.7108993804763810154, 1.000000000000000000),
 ( 1.000000000000000000, 0.7108100171490865371, 1.000000000000000000),
 ( 1.000000000000000000, 0.7106191415567553182, 1.000000000000000000),
 ( 1.000000000000000000, 0.7105185320923615988, 1.000000000000000000),
 ( 1.000000000000000000, 0.7102014790723295556, 1.000000000000000000),
 ( 1.000000000000000000, 0.7099699576740480245, 1.000000000000000000),
 ( 1.000000000000000000, 0.7095909300315041968, 1.000000000000000000),
 ( 1.000000000000000000, 0.7094593121158984106, 1.000000000000000000),
 ( 1.000000000000000000, 0.7091910831477740151, 1.000000000000000000),
 ( 1.000000000000000000, 0.7090537746377550965, 1.000000000000000000),
 ( 1.000000000000000000, 0.7087727591781153302, 1.000000000000000000),
 ( 1.000000000000000000, 0.7086290523620303317, 1.000000000000000000),
 ( 1.000000000000000000, 0.7084085592173990920, 1.000000000000000000),
 ( 1.000000000000000000, 0.7083342380281847372, 1.000000000000000000),
 ( 1.000000000000000000, 0.7081839094109132482, 1.000000000000000000),
 ( 1.000000000000000000, 0.7081077478408333015, 1.000000000000000000),
 ( 1.000000000000000000, 0.7077267031860466906, 1.000000000000000000),
 ( 1.000000000000000000, 0.7074184602291956336, 1.000000000000000000),
 ( 1.000000000000000000, 0.7071067811865476838, 1.000000000000000000) ) ) 
 REPRESENTATION_ITEM ( '' )  SURFACE ( )  );
#9941=CARTESIAN_POINT ( 'NONE',  ( 16.35719767791491819, 136.8501131444031387, 5.449348266248943418 ) ) ;
#9944=EDGE_CURVE ( 'NONE', #6282, #10721, #15219, .T. ) ;
#9946=LINE ( 'NONE', #11535, #14673 ) ;
#9948=CARTESIAN_POINT ( 'NONE',  ( 23.77503517897901375, 18.00000000000000000, 22.95135521423614833 ) ) ;
#9950=ORIENTED_EDGE ( 'NONE', *, *, #8573, .T. ) ;
#9956=ORIENTED_EDGE ( 'NONE', *, *, #10082, .F. ) ;
#9957=VERTEX_POINT ( 'NONE', #11233 ) ;
#9958=CARTESIAN_POINT ( 'NONE',  ( 9.276452510677492214, 132.6951329324795381, 12.46699917133672741 ) ) ;
#9963=CARTESIAN_POINT ( 'NONE',  ( 196.0000000000000000, 183.6227766016837961, 5.571800142134975431 ) ) ;
#9967=CARTESIAN_POINT ( 'NONE',  ( 34.48889888759456568, 144.3473407286824965, 18.59810793231920201 ) ) ;
#9968=DIRECTION ( 'NONE',  ( 0.000000000000000000, -0.8660254037844413721, 0.4999999999999953371 ) ) ;
#9969=CARTESIAN_POINT ( 'NONE',  ( -100.0000000000000000, 143.0439382767972347, 16.49999999999984368 ) ) ;
#9973=EDGE_CURVE ( 'NONE', #11927, #2395, #15145, .T. ) ;
#9976=DIRECTION ( 'NONE',  ( -1.000000000000000000, 0.000000000000000000, 0.000000000000000000 ) ) ;
#9978=DIRECTION ( 'NONE',  ( 0.01578383822436034076, -0.1110972697184772484, -0.9936841888205766304 ) ) ;
#9979=VERTEX_POINT ( 'NONE', #3004 ) ;
#9991=ORIENTED_EDGE ( 'NONE', *, *, #12630, .F. ) ;
#9992=CYLINDRICAL_SURFACE ( 'NONE', #12315, 10.00000000000000000 ) ;
#9994=ORIENTED_EDGE ( 'NONE', *, *, #9881, .F. ) ;
#9995=EDGE_CURVE ( 'NONE', #6282, #6096, #798, .T. ) ;
#9997=DIRECTION ( 'NONE',  ( -0.000000000000000000, -0.000000000000000000, -1.000000000000000000 ) ) ;
#9998=LINE ( 'NONE', #3200, #12619 ) ;
#10001=CARTESIAN_POINT ( 'NONE',  ( -8.720613081040614389, 18.00000000000000000, 24.99999999951824492 ) ) ;
#10007=VERTEX_POINT ( 'NONE', #12485 ) ;
#10010=VERTEX_POINT ( 'NONE', #14959 ) ;
#10014=AXIS2_PLACEMENT_3D ( 'NONE', #15332, #7370, #6038 ) ;
#10015=CARTESIAN_POINT ( 'NONE',  ( 22.87244304995705235, 29.89498257257996272, 11.09085247437311494 ) ) ;
#10017=CARTESIAN_POINT ( 'NONE',  ( 20.41303537792882139, 140.1262507166239573, 15.26811025958205015 ) ) ;
#10018=EDGE_LOOP ( 'NONE', ( #16525, #999, #4479, #8552 ) ) ;
#10021=CYLINDRICAL_SURFACE ( 'NONE', #3281, 2.499999999999998668 ) ;
#10022=CARTESIAN_POINT ( 'NONE',  ( -76.34901055807858938, 193.2024116766813506, 24.96685975555418224 ) ) ;
#10023=DIRECTION ( 'NONE',  ( -0.000000000000000000, 1.000000000000000000, 0.000000000000000000 ) ) ;
#10025=CARTESIAN_POINT ( 'NONE',  ( 196.0000000000000000, 163.6227766016838530, 12.50000337241049309 ) ) ;
#10029=LINE ( 'NONE', #581, #3050 ) ;
#10034=CIRCLE ( 'NONE', #8906, 10.00000000000000178 ) ;
#10036=ORIENTED_EDGE ( 'NONE', *, *, #13706, .T. ) ;
#10038=ORIENTED_EDGE ( 'NONE', *, *, #2843, .T. ) ;
#10039=CARTESIAN_POINT ( 'NONE',  ( 48.00000000000000711, 175.6227766016838530, 21.92820660268601074 ) ) ;
#10043=ORIENTED_EDGE ( 'NONE', *, *, #14669, .F. ) ;
#10048=CARTESIAN_POINT ( 'NONE',  ( -27.98221281347037959, 30.00000000000000000, 0.000000000000000000 ) ) ;
#10061=EDGE_CURVE ( 'NONE', #13439, #12155, #9578, .T. ) ;
#10072=VECTOR ( 'NONE', #1333, 1000.000000000000000 ) ;
#10075=EDGE_LOOP ( 'NONE', ( #64, #4342, #16688, #15880 ) ) ;
#10078=CARTESIAN_POINT ( 'NONE',  ( -84.01788347118190359, 199.6128501304145004, 17.48539201980444346 ) ) ;
#10080=ORIENTED_EDGE ( 'NONE', *, *, #12304, .T. ) ;
#10082=EDGE_CURVE ( 'NONE', #15131, #16992, #15391, .T. ) ;
#10084=B_SPLINE_CURVE_WITH_KNOTS ( 'NONE', 3,
 ( #10469, #17372, #7548, #6302 ),
 .UNSPECIFIED., .F., .F.,
 ( 4, 4 ),
 ( 0.000000000000000000, 0.0004807729677303993116 ),
 .UNSPECIFIED. ) ;
#10090=EDGE_CURVE ( 'NONE', #11495, #11331, #9289, .T. ) ;
#10093=ADVANCED_FACE ( 'NONE', ( #15483 ), #15650, .F. ) ;
#10094=EDGE_CURVE ( 'NONE', #2358, #6948, #16385, .T. ) ;
#10097=CARTESIAN_POINT ( 'NONE',  ( -12.79675654462651124, 18.00000000000000355, 5.581853174322293221 ) ) ;
#10100=AXIS2_PLACEMENT_3D ( 'NONE', #6136, #7774, #3723 ) ;
#10103=CYLINDRICAL_SURFACE ( 'NONE', #7582, 11.99999999999999645 ) ;
#10108=ORIENTED_EDGE ( 'NONE', *, *, #6850, .T. ) ;
#10109=CARTESIAN_POINT ( 'NONE',  ( 30.00000000000001066, 146.6227766016838245, 0.000000000000000000 ) ) ;
#10110=CARTESIAN_POINT ( 'NONE',  ( 23.71167364621568652, 19.99999999999772982, 10.06760101871518032 ) ) ;
#10114=CYLINDRICAL_SURFACE ( 'NONE', #4131, 27.69059892324149530 ) ;
#10120=CARTESIAN_POINT ( 'NONE',  ( -91.33974596215561803, 206.6227766016838245, 0.000000000000000000 ) ) ;
#10121=ORIENTED_EDGE ( 'NONE', *, *, #6112, .T. ) ;
#10123=ADVANCED_FACE ( 'NONE', ( #7597 ), #8671, .T. ) ;
#10125=VECTOR ( 'NONE', #14711, 1000.000000000000000 ) ;
#10127=ADVANCED_FACE ( 'NONE', ( #3450 ), #4503, .T. ) ;
#10128=ORIENTED_EDGE ( 'NONE', *, *, #995, .T. ) ;
#10130=CIRCLE ( 'NONE', #10988, 33.00000000000000000 ) ;
#10137=AXIS2_PLACEMENT_3D ( 'NONE', #8759, #704, #10330 ) ;
#10142=CARTESIAN_POINT ( 'NONE',  ( 7.743794661876905572, 133.6328069455646528, 12.86244959688548128 ) ) ;
#10143=DIRECTION ( 'NONE',  ( -0.000000000000000000, -0.000000000000000000, 1.000000000000000000 ) ) ;
#10144=LINE ( 'NONE', #2345, #17399 ) ;
#10146=CARTESIAN_POINT ( 'NONE',  ( 30.46461711770098546, 141.6391889668067563, 13.78368973859836011 ) ) ;
#10147=CARTESIAN_POINT ( 'NONE',  ( -80.00000000000001421, 196.6227766016838245, 10.00000000000000178 ) ) ;
#10149=CARTESIAN_POINT ( 'NONE',  ( -75.00000000000002842, 146.6227766016838245, 35.00200000000000244 ) ) ;
#10152=DIRECTION ( 'NONE',  ( 1.000000000000000000, -1.243449787580175325E-14, 0.000000000000000000 ) ) ;
#10157=ORIENTED_EDGE ( 'NONE', *, *, #2718, .T. ) ;
#10159=ORIENTED_EDGE ( 'NONE', *, *, #17062, .T. ) ;
#10165=EDGE_CURVE ( 'NONE', #10977, #7447, #10514, .T. ) ;
#10176=VECTOR ( 'NONE', #8107, 1000.000000000000000 ) ;
#10177=VECTOR ( 'NONE', #9909, 1000.000000000000000 ) ;
#10179=EDGE_LOOP ( 'NONE', ( #14535, #6332, #12430, #11238 ) ) ;
#10182=DIRECTION ( 'NONE',  ( -1.000000000000000000, -0.000000000000000000, -0.000000000000000000 ) ) ;
#10183=EDGE_LOOP ( 'NONE', ( #2598, #2422 ) ) ;
#10190=CARTESIAN_POINT ( 'NONE',  ( -15.37626115774789248, 32.49812920269235406, 8.581855491731886332 ) ) ;
#10192=AXIS2_PLACEMENT_3D ( 'NONE', #404, #7224, #12625 ) ;
#10198=EDGE_CURVE ( 'NONE', #12616, #13477, #13251, .T. ) ;
#10199=CARTESIAN_POINT ( 'NONE',  ( -82.50000000000002842, 146.6227766016838245, 10.00000000000000178 ) ) ;
#10200=EDGE_CURVE ( 'NONE', #12465, #4289, #5359, .T. ) ;
#10203=CARTESIAN_POINT ( 'NONE',  ( 34.80468147095351128, 20.00000000000000000, 7.619145204522578041 ) ) ;
#10205=CARTESIAN_POINT ( 'NONE',  ( 24.29786737972285238, 29.87659578631513568, 8.527395788633878482 ) ) ;
#10207=DIRECTION ( 'NONE',  ( 0.000000000000000000, -0.000000000000000000, -1.000000000000000000 ) ) ;
#10208=CARTESIAN_POINT ( 'NONE',  ( -75.01973743086520585, 196.1036955441148280, 22.13227804827260314 ) ) ;
#10210=DIRECTION ( 'NONE',  ( -0.000000000000000000, -0.000000000000000000, -1.000000000000000000 ) ) ;
#10216=EDGE_LOOP ( 'NONE', ( #12506, #4962 ) ) ;
#10218=CARTESIAN_POINT ( 'NONE',  ( -95.00000000000000000, 171.6227766016838245, 0.000000000000000000 ) ) ;
#10221=ORIENTED_EDGE ( 'NONE', *, *, #13567, .F. ) ;
#10224=EDGE_LOOP ( 'NONE', ( #14318, #11193, #10635, #13011, #5329, #9488, #3075, #14651, #1099, #13137 ) ) ;
#10230=CARTESIAN_POINT ( 'NONE',  ( 34.26467700469002153, 18.00000000000000000, 10.17319632352554137 ) ) ;
#10231=DIRECTION ( 'NONE',  ( 0.000000000000000000, 1.000000000000000000, 0.000000000000000000 ) ) ;
#10232=ORIENTED_EDGE ( 'NONE', *, *, #11046, .F. ) ;
#10235=CARTESIAN_POINT ( 'NONE',  ( -15.00000000000001421, 20.00000000000004263, 4.999999999999999112 ) ) ;
#10238=CARTESIAN_POINT ( 'NONE',  ( 29.39065902011773446, 201.5868197762109730, 13.82597759728686349 ) ) ;
#10240=DIRECTION ( 'NONE',  ( -0.000000000000000000, -0.000000000000000000, -1.000000000000000000 ) ) ;
#10241=ORIENTED_EDGE ( 'NONE', *, *, #8453, .F. ) ;
#10246=EDGE_CURVE ( 'NONE', #14256, #3772, #14771, .T. ) ;
#10250=CARTESIAN_POINT ( 'NONE',  ( 16.17028938446068764, 143.0439382767918346, 16.49999999999050360 ) ) ;
#10251=DIRECTION ( 'NONE',  ( 1.000000000000000000, 0.000000000000000000, 0.000000000000000000 ) ) ;
#10254=EDGE_LOOP ( 'NONE', ( #11378, #8728 ) ) ;
#10265=CARTESIAN_POINT ( 'NONE',  ( 27.50000000000001066, 146.6227766016838245, 0.000000000000000000 ) ) ;
#10266=CARTESIAN_POINT ( 'NONE',  ( -24.81085081034726869, 18.00000000000000000, 15.69149817755460496 ) ) ;
#10269=EDGE_LOOP ( 'NONE', ( #7649, #2026, #8630, #11409 ) ) ;
#10275=ORIENTED_EDGE ( 'NONE', *, *, #8629, .F. ) ;
#10276=EDGE_CURVE ( 'NONE', #4551, #13275, #3985, .T. ) ;
#10277=CARTESIAN_POINT ( 'NONE',  ( 19.49710218362280045, 19.99999999999999289, 24.48336163992366465 ) ) ;
#10278=CARTESIAN_POINT ( 'NONE',  ( 28.14717441101472772, 19.99999999999999645, 20.07001214883818108 ) ) ;
#10279=AXIS2_PLACEMENT_3D ( 'NONE', #3524, #6442, #2194 ) ;
#10280=ORIENTED_EDGE ( 'NONE', *, *, #658, .F. ) ;
#10283=DIRECTION ( 'NONE',  ( -0.000000000000000000, 1.000000000000000000, 0.000000000000000000 ) ) ;
#10284=CARTESIAN_POINT ( 'NONE',  ( -34.99999999999999289, 130.0000000000000000, 0.000000000000000000 ) ) ;
#10287=CARTESIAN_POINT ( 'NONE',  ( 35.00000000000000000, 196.6227766016838245, 35.00200000000000244 ) ) ;
#10289=ORIENTED_EDGE ( 'NONE', *, *, #8575, .F. ) ;
#10295=ORIENTED_EDGE ( 'NONE', *, *, #1598, .F. ) ;
#10300=CARTESIAN_POINT ( 'NONE',  ( -18.23240235453911140, 32.30379688028049401, 5.697301546657946858 ) ) ;
#10307=ORIENTED_EDGE ( 'NONE', *, *, #3391, .T. ) ;
#10309=CARTESIAN_POINT ( 'NONE',  ( -70.00000000000000000, 171.6227766016838245, 0.000000000000000000 ) ) ;
#10310=CARTESIAN_POINT ( 'NONE',  ( 30.00000000000000355, 196.6227766016838245, 0.000000000000000000 ) ) ;
#10314=CIRCLE ( 'NONE', #9487, 10.00000000000000178 ) ;
#10315=CARTESIAN_POINT ( 'NONE',  ( 27.29413616237980023, 200.8416626254457356, 15.34246182976916195 ) ) ;
#10319=DIRECTION ( 'NONE',  ( 0.000000000000000000, 1.000000000000000000, 0.000000000000000000 ) ) ;
#10323=DIRECTION ( 'NONE',  ( -1.224646799147353207E-16, -1.000000000000000000, 0.000000000000000000 ) ) ;
#10330=DIRECTION ( 'NONE',  ( -1.000000000000000000, 0.000000000000000000, -0.000000000000000000 ) ) ;
#10331=AXIS2_PLACEMENT_3D ( 'NONE', #7132, #5459, #6955 ) ;
#10340=ADVANCED_FACE ( 'NONE', ( #12373 ), #10860, .F. ) ;
#10342=ORIENTED_EDGE ( 'NONE', *, *, #11865, .T. ) ;
#10343=DIRECTION ( 'NONE',  ( -1.000000000000000000, -0.000000000000000000, -0.000000000000000000 ) ) ;
#10346=ORIENTED_EDGE ( 'NONE', *, *, #5015, .F. ) ;
#10349=DIRECTION ( 'NONE',  ( 1.000000000000000000, 0.000000000000000000, 0.000000000000000000 ) ) ;
#10351=DIRECTION ( 'NONE',  ( 0.000000000000000000, 0.000000000000000000, 1.000000000000000000 ) ) ;
#10352=CARTESIAN_POINT ( 'NONE',  ( -12.78422937319141184, 31.72181100014091726, 11.38907491820491913 ) ) ;
#10354=AXIS2_PLACEMENT_3D ( 'NONE', #1512, #9648, #5679 ) ;
#10365=CARTESIAN_POINT ( 'NONE',  ( 33.88556156013721932, 19.99999999999999645, 11.42442012027869858 ) ) ;
#10367=CARTESIAN_POINT ( 'NONE',  ( 23.06881488990584472, 29.89244155294396066, 10.82591622123929653 ) ) ;
#10368=ORIENTED_EDGE ( 'NONE', *, *, #2331, .F. ) ;
#10370=CARTESIAN_POINT ( 'NONE',  ( 49.99999999999998579, 187.6227766016837961, 12.50000337241049309 ) ) ;
#10372=CARTESIAN_POINT ( 'NONE',  ( -68.00000000000000000, 154.3022685259950038, 9.999999999999900524 ) ) ;
#10374=EDGE_CURVE ( 'NONE', #190, #4855, #2241, .T. ) ;
#10376=DIRECTION ( 'NONE',  ( -1.000000000000000000, -0.000000000000000000, 0.000000000000000000 ) ) ;
#10386=DIRECTION ( 'NONE',  ( 8.673617379884037937E-17, 0.000000000000000000, -1.000000000000000000 ) ) ;
#10387=ORIENTED_EDGE ( 'NONE', *, *, #14471, .T. ) ;
#10390=DIRECTION ( 'NONE',  ( -1.000000000000000000, -0.000000000000000000, -0.000000000000000000 ) ) ;
#10392=CARTESIAN_POINT ( 'NONE',  ( 22.65507808637627818, 17.99999999999885958, 7.619675430596801746 ) ) ;
#10394=EDGE_CURVE ( 'NONE', #2500, #14680, #7903, .T. ) ;
#10397=CARTESIAN_POINT ( 'NONE',  ( 21.47128797932978372, 141.5899928260317040, 13.68519783011616653 ) ) ;
#10398=DIRECTION ( 'NONE',  ( -1.000000000000000000, -6.938893903907228378E-16, 0.000000000000000000 ) ) ;
#10404=EDGE_CURVE ( 'NONE', #13335, #1164, #11123, .T. ) ;
#10407=CARTESIAN_POINT ( 'NONE',  ( 30.45233391750860363, 201.6036812327912457, 13.78933345224469420 ) ) ;
#10409=ORIENTED_EDGE ( 'NONE', *, *, #11865, .F. ) ;
#10414=CARTESIAN_POINT ( 'NONE',  ( -79.53538288229906073, 141.6391889668067279, 13.78368973859834767 ) ) ;
#10418=EDGE_LOOP ( 'NONE', ( #948, #1739, #10916, #4570 ) ) ;
#10422=CARTESIAN_POINT ( 'NONE',  ( 15.00000000000903455, 143.2885527162398489, 16.91661185963483760 ) ) ;
#10425=AXIS2_PLACEMENT_3D ( 'NONE', #14728, #4891, #13126 ) ;
#10427=EDGE_LOOP ( 'NONE', ( #15343, #1519 ) ) ;
#10428=B_SPLINE_CURVE_WITH_KNOTS ( 'NONE', 3,
 ( #13910, #14172, #4607, #8403, #4432, #4690, #10078, #1771, #9726, #13823, #8578, #12752, #11138, #12563, #11234, #1689, #7086, #8760, #620, #12486, #431, #351, #7347, #16905, #532, #7254, #13990, #16559, #1854, #14083, #8497, #15124, #5838, #11408, #12657, #705, #6018, #6099, #11330, #5751, #16654, #5938 ),
 .UNSPECIFIED., .F., .F.,
 ( 4, 2, 2, 2, 2, 2, 2, 2, 2, 2, 2, 2, 2, 2, 2, 2, 2, 2, 2, 2, 4 ),
 ( 0.000000000000000000, 0.002803867404946369657, 0.004205801107419573567, 0.005607734809892779212, 0.007009668512365983123, 0.008411602214839187033, 0.009112569066075807203, 0.009813535917312425638, 0.01051450276854904407, 0.01086498619416737324, 0.01121546961978570067, 0.01156595304540402810, 0.01191643647102235727, 0.01261740332225898438, 0.01331837017349561149, 0.01401933702473223860, 0.01542127072720551710, 0.01682320442967879734, 0.01822513813215207931, 0.01962707183462535782, 0.02243093923957190788 ),
 .UNSPECIFIED. ) ;
#10430=ORIENTED_EDGE ( 'NONE', *, *, #5159, .T. ) ;
#10432=ORIENTED_EDGE ( 'NONE', *, *, #3323, .T. ) ;
#10438=AXIS2_PLACEMENT_3D ( 'NONE', #1436, #10887, #9393 ) ;
#10439=DIRECTION ( 'NONE',  ( 0.000000000000000000, 0.000000000000000000, 1.000000000000000000 ) ) ;
#10440=AXIS2_PLACEMENT_3D ( 'NONE', #11343, #11601, #3633 ) ;
#10441=FACE_OUTER_BOUND ( 'NONE', #13539, .T. ) ;
#10445=CARTESIAN_POINT ( 'NONE',  ( -15.00000000000002132, 100.0000000000000142, 4.999999999999999112 ) ) ;
#10446=CARTESIAN_POINT ( 'NONE',  ( 34.93420767853316988, 20.00000000000000000, 4.999999999999999112 ) ) ;
#10448=CARTESIAN_POINT ( 'NONE',  ( -15.50256837817153333, 32.53516993624282350, 8.343687756225392604 ) ) ;
#10452=CARTESIAN_POINT ( 'NONE',  ( 49.99999999999998579, 163.6227766016838530, 15.00000337241049486 ) ) ;
#10455=EDGE_LOOP ( 'NONE', ( #895, #10793, #10346, #5643 ) ) ;
#10457=VECTOR ( 'NONE', #14676, 1000.000000000000000 ) ;
#10460=CARTESIAN_POINT ( 'NONE',  ( -13.34744738361370509, 20.00000000000116174, 11.18154278182822026 ) ) ;
#10461=CARTESIAN_POINT ( 'NONE',  ( 49.99999999999998579, 167.6227766016838814, 21.92820660268601074 ) ) ;
#10462=CARTESIAN_POINT ( 'NONE',  ( 16.23563086566769442, 20.00000000000456879, 14.95434718295347665 ) ) ;
#10463=VECTOR ( 'NONE', #12404, 1000.000000000000000 ) ;
#10466=ADVANCED_FACE ( 'NONE', ( #3077 ), #12989, .F. ) ;
#10468=EDGE_CURVE ( 'NONE', #6230, #16788, #14400, .T. ) ;
#10469=CARTESIAN_POINT ( 'NONE',  ( 15.00000000000903455, 143.2885527162398489, 16.91661185963483760 ) ) ;
#10471=DIRECTION ( 'NONE',  ( 1.000000000000000000, 0.000000000000000000, 0.000000000000000000 ) ) ;
#10473=EDGE_LOOP ( 'NONE', ( #8557, #1675, #580, #10818 ) ) ;
#10486=FACE_OUTER_BOUND ( 'NONE', #17421, .T. ) ;
#10489=FACE_OUTER_BOUND ( 'NONE', #15457, .T. ) ;
#10490=CARTESIAN_POINT ( 'NONE',  ( 27.48361012695488981, 138.6227766016838245, 1.225897272825924533 ) ) ;
#10491=ORIENTED_EDGE ( 'NONE', *, *, #12091, .T. ) ;
#10492=CARTESIAN_POINT ( 'NONE',  ( 26.01985846803728464, 139.8002605074728990, 8.764508151440994155 ) ) ;
#10495=CARTESIAN_POINT ( 'NONE',  ( 27.15273249069231198, 18.00000000000000000, 20.88767039909325973 ) ) ;
#10496=CARTESIAN_POINT ( 'NONE',  ( 18.77390920412167929, 29.94862569121198348, 14.25030649093772972 ) ) ;
#10497=ORIENTED_EDGE ( 'NONE', *, *, #2989, .T. ) ;
#10499=CARTESIAN_POINT ( 'NONE',  ( 17.58250999373992585, 125.2198453306090329, -1.325401613797208934E-14 ) ) ;
#10511=EDGE_CURVE ( 'NONE', #1871, #6747, #16946, .T. ) ;
#10512=ORIENTED_EDGE ( 'NONE', *, *, #8573, .F. ) ;
#10514=LINE ( 'NONE', #1312, #8447 ) ;
#10515=CYLINDRICAL_SURFACE ( 'NONE', #13578, 2.499999999999998668 ) ;
#10520=B_SPLINE_CURVE_WITH_KNOTS ( 'NONE', 3,
 ( #3938, #5516, #12068, #2775, #10904, #16155, #8254, #2607, #16236, #9407, #7992, #17377, #13398, #16328, #4194, #12241, #2511, #1361, #4028, #6767, #6922, #2860, #12163, #11976, #10653, #1266, #9577, #6672, #17477, #2687, #14732, #9231, #5247, #16059, #14984, #9321, #10552, #14810, #5346, #10745, #13583, #13663 ),
 .UNSPECIFIED., .F., .F.,
 ( 4, 2, 2, 2, 2, 2, 2, 2, 2, 2, 2, 2, 2, 2, 2, 2, 2, 2, 2, 2, 4 ),
 ( 0.000000000000000000, 0.002338598163723745824, 0.002923247704654685208, 0.003507897245585624591, 0.004677196327447558435, 0.005846495409309493581, 0.006431144950240438168, 0.007015794491171381889, 0.008185093573033232900, 0.008769743113964166212, 0.009354392654895101258, 0.01052369173675698003, 0.01110834127768790640, 0.01169299081861883277, 0.01286228990048068378, 0.01403158898234253132, 0.01461623852327344902, 0.01520088806420436672, 0.01637018714606625763, 0.01753948622792814507, 0.01870878530979003598 ),
 .UNSPECIFIED. ) ;
#10528=CARTESIAN_POINT ( 'NONE',  ( 48.00000000000000000, 171.6227766016838245, 12.50000337241049131 ) ) ;
#10532=DIRECTION ( 'NONE',  ( 0.000000000000000000, 0.000000000000000000, 1.000000000000000000 ) ) ;
#10533=DIRECTION ( 'NONE',  ( -1.000000000000000000, 0.000000000000000000, 0.000000000000000000 ) ) ;
#10534=CARTESIAN_POINT ( 'NONE',  ( -45.00000000000000000, 140.0000000000000000, 15.00000000000000000 ) ) ;
#10536=DIRECTION ( 'NONE',  ( -1.000000000000000000, -6.938893903907228378E-16, 0.000000000000000000 ) ) ;
#10537=EDGE_LOOP ( 'NONE', ( #1180, #15630, #4222, #11815 ) ) ;
#10542=LINE ( 'NONE', #13304, #2376 ) ;
#10543=CARTESIAN_POINT ( 'NONE',  ( 26.85584576128377066, 139.3465472469502231, 6.878002324459898453 ) ) ;
#10545=CARTESIAN_POINT ( 'NONE',  ( 15.58467296311467898, 20.00000000000226308, 15.00881168888636807 ) ) ;
#10546=EDGE_LOOP ( 'NONE', ( #10275, #6971, #10694, #2850 ) ) ;
#10547=DIRECTION ( 'NONE',  ( 1.000000000000000000, 0.000000000000000000, 0.000000000000000000 ) ) ;
#10552=CARTESIAN_POINT ( 'NONE',  ( 34.65073054311758938, 148.4807726931354068, 23.52860204907123887 ) ) ;
#10559=ORIENTED_EDGE ( 'NONE', *, *, #1193, .T. ) ;
#10561=ORIENTED_EDGE ( 'NONE', *, *, #7117, .T. ) ;
#10567=CARTESIAN_POINT ( 'NONE',  ( -16.30611068361787019, 32.76923076923078781, 4.999999999999999112 ) ) ;
#10568=CARTESIAN_POINT ( 'NONE',  ( -15.84744341939753021, 31.82541372190370055, 11.32583567006417624 ) ) ;
#10569=LINE ( 'NONE', #15977, #827 ) ;
#10570=CARTESIAN_POINT ( 'NONE',  ( 33.88365274872860766, 18.00000000000000000, 11.43011099234507277 ) ) ;
#10571=CARTESIAN_POINT ( 'NONE',  ( -84.46546100545653246, 148.8772865214095873, 23.90975478891752459 ) ) ;
#10579=CARTESIAN_POINT ( 'NONE',  ( 21.04314855419486108, 29.91877537971376455, 12.94423386069545323 ) ) ;
#10580=EDGE_LOOP ( 'NONE', ( #1449, #2332, #15659, #7787 ) ) ;
#10581=CARTESIAN_POINT ( 'NONE',  ( -95.00000000000000000, 171.6227766016838245, 30.00000000000000000 ) ) ;
#10583=ORIENTED_EDGE ( 'NONE', *, *, #10165, .T. ) ;
#10585=DIRECTION ( 'NONE',  ( 1.000000000000000000, 0.000000000000000000, 0.000000000000000000 ) ) ;
#10589=CARTESIAN_POINT ( 'NONE',  ( -76.36134094103634595, 143.1809062453614558, 16.74061342279920339 ) ) ;
#10591=DIRECTION ( 'NONE',  ( -1.000000000000000000, -0.000000000000000000, -0.000000000000000000 ) ) ;
#10593=LINE ( 'NONE', #14585, #17076 ) ;
#10594=ORIENTED_EDGE ( 'NONE', *, *, #11523, .F. ) ;
#10597=EDGE_CURVE ( 'NONE', #5655, #9695, #1926, .T. ) ;
#10602=VECTOR ( 'NONE', #15919, 1000.000000000000000 ) ;
#10606=CARTESIAN_POINT ( 'NONE',  ( -3.000000000000000888, 171.6227766016838245, 0.000000000000000000 ) ) ;
#10612=DIRECTION ( 'NONE',  ( -1.000000000000000000, -0.000000000000000000, -0.000000000000000000 ) ) ;
#10613=CYLINDRICAL_SURFACE ( 'NONE', #9319, 2.499999999999998668 ) ;
#10618=PLANE ( 'NONE',  #14059 ) ;
#10620=AXIS2_PLACEMENT_3D ( 'NONE', #7265, #5949, #3460 ) ;
#10625=DIRECTION ( 'NONE',  ( 1.000000000000000000, 0.000000000000000000, -0.000000000000000000 ) ) ;
#10630=DIRECTION ( 'NONE',  ( -1.000000000000000000, 0.000000000000000000, 0.000000000000000000 ) ) ;
#10634=CIRCLE ( 'NONE', #13473, 30.00000000000000000 ) ;
#10635=ORIENTED_EDGE ( 'NONE', *, *, #15550, .T. ) ;
#10636=EDGE_CURVE ( 'NONE', #15924, #1583, #8989, .T. ) ;
#10637=CARTESIAN_POINT ( 'NONE',  ( -8.097611523674038025, 19.99999999997653788, 14.83628426572619219 ) ) ;
#10638=EDGE_CURVE ( 'NONE', #9170, #6523, #11997, .T. ) ;
#10639=CARTESIAN_POINT ( 'NONE',  ( 15.45419697039644902, 125.5863960662987040, 6.086967932831932160 ) ) ;
#10640=ORIENTED_EDGE ( 'NONE', *, *, #320, .F. ) ;
#10641=CARTESIAN_POINT ( 'NONE',  ( 18.47379060770018810, 20.00000000000225953, 14.40819024183099728 ) ) ;
#10645=AXIS2_PLACEMENT_3D ( 'NONE', #6370, #11676, #13288 ) ;
#10647=DIRECTION ( 'NONE',  ( -1.000000000000000000, -0.000000000000000000, -0.000000000000000000 ) ) ;
#10651=CIRCLE ( 'NONE', #6398, 2.500000000000002220 ) ;
#10653=CARTESIAN_POINT ( 'NONE',  ( 31.52945631074817356, 151.3869516943736357, 26.06757126999134755 ) ) ;
#10656=DIRECTION ( 'NONE',  ( 0.000000000000000000, 0.000000000000000000, 1.000000000000000000 ) ) ;
#10658=ORIENTED_EDGE ( 'NONE', *, *, #6556, .T. ) ;
#10661=CARTESIAN_POINT ( 'NONE',  ( 15.00000000000000000, 206.6227766016838245, -2.143131898507868248E-15 ) ) ;
#10669=CARTESIAN_POINT ( 'NONE',  ( -81.91034726766426388, 151.2585272520459512, 25.96811968750270339 ) ) ;
#10670=EDGE_CURVE ( 'NONE', #11875, #16488, #6076, .T. ) ;
#10671=EDGE_LOOP ( 'NONE', ( #11807, #15798, #7561, #10832 ) ) ;
#10675=CARTESIAN_POINT ( 'NONE',  ( 16.69631138515844171, 126.9345490261019904, 8.565329098038530375 ) ) ;
#10679=ORIENTED_EDGE ( 'NONE', *, *, #15423, .F. ) ;
#10680=LINE ( 'NONE', #10771, #8356 ) ;
#10682=CARTESIAN_POINT ( 'NONE',  ( -40.00000000000000000, 20.00000000000000000, 30.00000000000000355 ) ) ;
#10683=LINE ( 'NONE', #5547, #9329 ) ;
#10684=EDGE_LOOP ( 'NONE', ( #5133, #7708 ) ) ;
#10689=MECHANICAL_DESIGN_GEOMETRIC_PRESENTATION_REPRESENTATION('',(#2787),#16069);
#10692=EDGE_CURVE ( 'NONE', #5017, #11907, #6423, .T. ) ;
#10693=DIRECTION ( 'NONE',  ( -1.000000000000000000, -0.000000000000000000, 0.000000000000000000 ) ) ;
#10694=ORIENTED_EDGE ( 'NONE', *, *, #6492, .T. ) ;
#10695=CARTESIAN_POINT ( 'NONE',  ( -725.0000000000000000, 19.99999999999995737, 13.00000000000000000 ) ) ;
#10696=CARTESIAN_POINT ( 'NONE',  ( 11.38015211399644500, 143.8700659084811093, 17.85516819212570638 ) ) ;
#10699=AXIS2_PLACEMENT_3D ( 'NONE', #11833, #17329, #16104 ) ;
#10702=VERTEX_POINT ( 'NONE', #17501 ) ;
#10705=VERTEX_POINT ( 'NONE', #10766 ) ;
#10706=DIRECTION ( 'NONE',  ( -1.000000000000000000, 0.000000000000000000, 0.000000000000000000 ) ) ;
#10710=CIRCLE ( 'NONE', #2226, 2.500000000000002220 ) ;
#10712=AXIS2_PLACEMENT_3D ( 'NONE', #5719, #3229, #15275 ) ;
#10713=CARTESIAN_POINT ( 'NONE',  ( 35.00000000000001421, 196.3674529106260707, 21.83698684826044101 ) ) ;
#10720=FACE_OUTER_BOUND ( 'NONE', #3330, .T. ) ;
#10721=VERTEX_POINT ( 'NONE', #5371 ) ;
#10722=DIRECTION ( 'NONE',  ( 0.000000000000000000, 0.000000000000000000, 1.000000000000000000 ) ) ;
#10723=ORIENTED_EDGE ( 'NONE', *, *, #3100, .T. ) ;
#10726=CARTESIAN_POINT ( 'NONE',  ( -45.00000000000000000, 122.0000000000000142, 0.000000000000000000 ) ) ;
#10729=CARTESIAN_POINT ( 'NONE',  ( -10.87333020471588974, 20.00000000000114753, 13.51515657978521645 ) ) ;
#10731=CARTESIAN_POINT ( 'NONE',  ( 14.12560798726494760, 138.8049619564753243, 7.597757983846928020 ) ) ;
#10733=CARTESIAN_POINT ( 'NONE',  ( 17.68052782483612617, 29.96314637258912583, 14.61659083303745632 ) ) ;
#10735=EDGE_LOOP ( 'NONE', ( #4195, #14390 ) ) ;
#10736=LINE ( 'NONE', #4100, #4711 ) ;
#10738=CIRCLE ( 'NONE', #586, 20.00000000000000355 ) ;
#10741=EDGE_CURVE ( 'NONE', #15996, #6096, #9159, .T. ) ;
#10743=ADVANCED_FACE ( 'NONE', ( #14568 ), #6518, .T. ) ;
#10744=ORIENTED_EDGE ( 'NONE', *, *, #6448, .F. ) ;
#10745=CARTESIAN_POINT ( 'NONE',  ( 34.98058807492896705, 147.1381844727102646, 22.12819033745955011 ) ) ;
#10746=VERTEX_POINT ( 'NONE', #5183 ) ;
#10747=DIRECTION ( 'NONE',  ( 0.000000000000000000, 0.000000000000000000, -1.000000000000000000 ) ) ;
#10749=EDGE_LOOP ( 'NONE', ( #14368, #7495, #15231, #9566 ) ) ;
#10754=CARTESIAN_POINT ( 'NONE',  ( 9.819856892917396607, 139.1316717379867214, 14.17181165802734988 ) ) ;
#10755=CIRCLE ( 'NONE', #3120, 35.00000000000000000 ) ;
#10760=CARTESIAN_POINT ( 'NONE',  ( -22.99999999999999289, 120.0000000000000142, 0.000000000000000000 ) ) ;
#10762=CARTESIAN_POINT ( 'NONE',  ( -75.68194015699739907, 149.1480937705748602, 24.16447509748838485 ) ) ;
#10764=DIRECTION ( 'NONE',  ( -1.000000000000000000, 0.000000000000000000, 0.000000000000000000 ) ) ;
#10766=CARTESIAN_POINT ( 'NONE',  ( 49.99999999999998579, 179.6227766016838245, 15.00000337241049486 ) ) ;
#10768=CARTESIAN_POINT ( 'NONE',  ( 16.25302816831168329, 18.00000000000000000, 25.00000000000000000 ) ) ;
#10771=CARTESIAN_POINT ( 'NONE',  ( -15.00000000000002132, 90.00000000000000000, 15.00000000000000000 ) ) ;
#10784=DIRECTION ( 'NONE',  ( 1.000000000000000000, 0.000000000000000000, 0.000000000000000000 ) ) ;
#10786=DIRECTION ( 'NONE',  ( -0.000000000000000000, -0.000000000000000000, -1.000000000000000000 ) ) ;
#10790=EDGE_CURVE ( 'NONE', #9609, #5289, #12286, .T. ) ;
#10793=ORIENTED_EDGE ( 'NONE', *, *, #13086, .F. ) ;
#10798=CARTESIAN_POINT ( 'NONE',  ( -27.99999999999998224, 10.00000000000000000, 0.000000000000000000 ) ) ;
#10800=CARTESIAN_POINT ( 'NONE',  ( 48.00000000000000711, 187.6227766016837961, 15.00000337241049486 ) ) ;
#10803=DIRECTION ( 'NONE',  ( 0.000000000000000000, 0.000000000000000000, 1.000000000000000000 ) ) ;
#10805=FACE_OUTER_BOUND ( 'NONE', #7239, .T. ) ;
#10808=DIRECTION ( 'NONE',  ( -1.000000000000000000, 0.000000000000000000, 0.000000000000000000 ) ) ;
#10810=EDGE_CURVE ( 'NONE', #4487, #2548, #8325, .T. ) ;
#10812=CARTESIAN_POINT ( 'NONE',  ( 196.0000000000000000, 159.6227766016838814, 5.571800142134975431 ) ) ;
#10814=CARTESIAN_POINT ( 'NONE',  ( -13.66886994730069560, 31.37497952739824214, 13.17845503416513075 ) ) ;
#10815=CARTESIAN_POINT ( 'NONE',  ( 13.54862175821475034, 128.4555333983033734, 9.713103375557215813 ) ) ;
#10817=CARTESIAN_POINT ( 'NONE',  ( 20.11141720500585350, 19.99999999999999645, 24.32074799214527516 ) ) ;
#10818=ORIENTED_EDGE ( 'NONE', *, *, #2506, .T. ) ;
#10823=ORIENTED_EDGE ( 'NONE', *, *, #847, .F. ) ;
#10824=CYLINDRICAL_SURFACE ( 'NONE', #8435, 2.500000000000002220 ) ;
#10827=ADVANCED_FACE ( 'NONE', ( #370 ), #3245, .F. ) ;
#10829=DIRECTION ( 'NONE',  ( -0.000000000000000000, -0.000000000000000000, -1.000000000000000000 ) ) ;
#10830=VERTEX_POINT ( 'NONE', #1880 ) ;
#10832=ORIENTED_EDGE ( 'NONE', *, *, #14371, .F. ) ;
#10834=EDGE_CURVE ( 'NONE', #6096, #817, #5771, .T. ) ;
#10837=DIRECTION ( 'NONE',  ( -1.000000000000000000, 0.000000000000000000, 0.000000000000000000 ) ) ;
#10838=DIRECTION ( 'NONE',  ( -1.000000000000000000, 0.000000000000000000, 0.000000000000000000 ) ) ;
#10839=CARTESIAN_POINT ( 'NONE',  ( -40.00000000000000000, 20.00000000000000000, 30.00000000000000355 ) ) ;
#10841=CARTESIAN_POINT ( 'NONE',  ( -79.62047275650606082, 151.6237922324447993, 26.24958334688937711 ) ) ;
#10850=CARTESIAN_POINT ( 'NONE',  ( 30.00000000000000355, 196.6227766016838245, 10.00000000000000178 ) ) ;
#10851=EDGE_CURVE ( 'NONE', #1349, #11959, #17385, .T. ) ;
#10860=CYLINDRICAL_SURFACE ( 'NONE', #7052, 2.499999999999998668 ) ;
#10865=AXIS2_PLACEMENT_3D ( 'NONE', #10534, #10625, #15941 ) ;
#10868=CARTESIAN_POINT ( 'NONE',  ( -22.99999999999999289, 100.0000000000000142, 0.000000000000000000 ) ) ;
#10874=CIRCLE ( 'NONE', #12579, 747.9999999999998863 ) ;
#10879=EDGE_CURVE ( 'NONE', #16992, #1871, #16495, .T. ) ;
#10883=DIRECTION ( 'NONE',  ( -0.000000000000000000, -0.000000000000000000, -1.000000000000000000 ) ) ;
#10886=ORIENTED_EDGE ( 'NONE', *, *, #17264, .T. ) ;
#10887=DIRECTION ( 'NONE',  ( -1.000000000000000000, 0.000000000000000000, -2.312964634635742464E-16 ) ) ;
#10889=ORIENTED_EDGE ( 'NONE', *, *, #10394, .T. ) ;
#10893=AXIS2_PLACEMENT_3D ( 'NONE', #13702, #16462, #13972 ) ;
#10896=VERTEX_POINT ( 'NONE', #13745 ) ;
#10898=CARTESIAN_POINT ( 'NONE',  ( 32.50000000000000000, 196.6227766016838245, 0.000000000000000000 ) ) ;
#10901=CARTESIAN_POINT ( 'NONE',  ( 30.00000000000001066, 146.6227766016838245, 35.00200000000000244 ) ) ;
#10904=CARTESIAN_POINT ( 'NONE',  ( 25.35214468288316070, 148.4718376841440204, 23.51742847763245337 ) ) ;
#10906=EDGE_LOOP ( 'NONE', ( #12424, #8633, #6551, #16134 ) ) ;
#10912=CARTESIAN_POINT ( 'NONE',  ( -27.99999999999998224, 10.00000000000000000, 0.000000000000000000 ) ) ;
#10913=CARTESIAN_POINT ( 'NONE',  ( 12.26645298401004425, 138.5600601684519120, 12.85897773338031946 ) ) ;
#10915=VECTOR ( 'NONE', #14348, 1000.000000000000000 ) ;
#10916=ORIENTED_EDGE ( 'NONE', *, *, #3787, .T. ) ;
#10921=FACE_OUTER_BOUND ( 'NONE', #10224, .T. ) ;
#10924=CARTESIAN_POINT ( 'NONE',  ( -76.03376373747714467, 149.6716700844112040, 24.64096846353360704 ) ) ;
#10925=ORIENTED_EDGE ( 'NONE', *, *, #7864, .T. ) ;
#10927=CARTESIAN_POINT ( 'NONE',  ( 14.80502546477524817, 129.0472650296936479, 11.28997929065621797 ) ) ;
#10929=DIRECTION ( 'NONE',  ( -1.000000000000000000, -0.000000000000000000, -0.000000000000000000 ) ) ;
#10931=AXIS2_PLACEMENT_3D ( 'NONE', #1686, #1590, #5835 ) ;
#10935=VECTOR ( 'NONE', #5111, 1000.000000000000000 ) ;
#10938=ORIENTED_EDGE ( 'NONE', *, *, #9874, .T. ) ;
#10941=LINE ( 'NONE', #239, #12453 ) ;
#10946=AXIS2_PLACEMENT_3D ( 'NONE', #6444, #4937, #9094 ) ;
#10948=CIRCLE ( 'NONE', #1635, 2.500000000000000000 ) ;
#10950=DIRECTION ( 'NONE',  ( 0.000000000000000000, -1.000000000000000000, 0.000000000000000000 ) ) ;
#10953=DIRECTION ( 'NONE',  ( 0.000000000000000000, 1.040834085586084059E-15, 1.000000000000000000 ) ) ;
#10960=CARTESIAN_POINT ( 'NONE',  ( 48.00000000000000711, 151.6227766016839098, 3.071800142134974099 ) ) ;
#10962=LINE ( 'NONE', #4245, #6372 ) ;
#10963=VERTEX_POINT ( 'NONE', #15858 ) ;
#10965=B_SPLINE_CURVE_WITH_KNOTS ( 'NONE', 3,
 ( #13154, #7665, #2180, #15718, #8991, #3870, #14402, #3512, #7745, #2270, #15813, #11912, #12001, #5276, #10579, #15988, #4920, #14664, #10496, #5012, #942, #17405, #7839, #11724, #7935 ),
 .UNSPECIFIED., .F., .F.,
 ( 4, 2, 2, 2, 2, 2, 2, 2, 2, 1, 2, 2, 4 ),
 ( 0.000000000000000000, 0.001953037758357041142, 0.002929556637535561930, 0.003906075516714082284, 0.005859113275071132533, 0.006835632154249659392, 0.007812151033428187119, 0.009765188791785242572, 0.01074170767096376509, 0.01171822655014228762, 0.01269474542932080841, 0.01367126430849933093, 0.01562430206685638465 ),
 .UNSPECIFIED. ) ;
#10970=CARTESIAN_POINT ( 'NONE',  ( 22.12508471281541134, 29.85770821936580433, 8.546410110412809402 ) ) ;
#10977=VERTEX_POINT ( 'NONE', #816 ) ;
#10980=ORIENTED_EDGE ( 'NONE', *, *, #5830, .T. ) ;
#10981=CARTESIAN_POINT ( 'NONE',  ( -27.98221281341758626, 19.99999999999999645, 6.321711414556861364 ) ) ;
#10988=AXIS2_PLACEMENT_3D ( 'NONE', #8835, #7590, #7246 ) ;
#10989=ORIENTED_EDGE ( 'NONE', *, *, #1766, .F. ) ;
#10990=CARTESIAN_POINT ( 'NONE',  ( -95.00000000000000000, 201.6227766016838245, 1.836970198721029589E-15 ) ) ;
#10992=CARTESIAN_POINT ( 'NONE',  ( 6.134011831684053284, 134.2062027339443944, 15.00000000000000000 ) ) ;
#10998=ORIENTED_EDGE ( 'NONE', *, *, #320, .T. ) ;
#11000=AXIS2_PLACEMENT_3D ( 'NONE', #2172, #7569, #857 ) ;
#11001=CARTESIAN_POINT ( 'NONE',  ( -40.00000000000000000, 20.00000000000000000, 28.00000000000000355 ) ) ;
#11003=VERTEX_POINT ( 'NONE', #13108 ) ;
#11007=EDGE_CURVE ( 'NONE', #7044, #6861, #11608, .T. ) ;
#11008=CARTESIAN_POINT ( 'NONE',  ( 196.0000000000000000, 171.6227766016838245, 12.50000337241049131 ) ) ;
#11010=CARTESIAN_POINT ( 'NONE',  ( 10.91733900447607830, 142.2434614804602404, 19.02291218241819593 ) ) ;
#11011=AXIS2_PLACEMENT_3D ( 'NONE', #1046, #5395, #1222 ) ;
#11016=DIRECTION ( 'NONE',  ( 0.000000000000000000, -0.000000000000000000, -1.000000000000000000 ) ) ;
#11017=DIRECTION ( 'NONE',  ( -1.000000000000000000, -0.000000000000000000, -0.000000000000000000 ) ) ;
#11018=DIRECTION ( 'NONE',  ( 1.000000000000000000, 0.000000000000000000, 0.000000000000000000 ) ) ;
#11019=CARTESIAN_POINT ( 'NONE',  ( 23.18512258076444610, 18.00000000000000000, 23.22991426836919615 ) ) ;
#11025=DIRECTION ( 'NONE',  ( 0.000000000000000000, -1.000000000000000000, 0.000000000000000000 ) ) ;
#11027=CIRCLE ( 'NONE', #12171, 2.500000000000002220 ) ;
#11034=VERTEX_POINT ( 'NONE', #14521 ) ;
#11035=CARTESIAN_POINT ( 'NONE',  ( -84.59125389484567847, 144.6221806392915425, 18.97834816100454702 ) ) ;
#11043=DIRECTION ( 'NONE',  ( 1.000000000000000000, 0.000000000000000000, 0.000000000000000000 ) ) ;
#11046=EDGE_CURVE ( 'NONE', #11034, #11927, #9742, .T. ) ;
#11050=DIRECTION ( 'NONE',  ( 0.000000000000000000, 0.000000000000000000, -1.000000000000000000 ) ) ;
#11055=ADVANCED_FACE ( 'NONE', ( #12222 ), #13465, .F. ) ;
#11056=FACE_OUTER_BOUND ( 'NONE', #7678, .T. ) ;
#11061=CARTESIAN_POINT ( 'NONE',  ( 20.22365234301270931, 29.89465715177047400, 11.02453202869212312 ) ) ;
#11073=EDGE_CURVE ( 'NONE', #3234, #2441, #17356, .T. ) ;
#11082=DIRECTION ( 'NONE',  ( 1.000000000000000000, 0.000000000000000000, 0.000000000000000000 ) ) ;
#11083=EDGE_CURVE ( 'NONE', #9695, #16992, #2693, .T. ) ;
#11084=ORIENTED_EDGE ( 'NONE', *, *, #16793, .F. ) ;
#11090=DIRECTION ( 'NONE',  ( -1.000000000000000000, -0.000000000000000000, -0.000000000000000000 ) ) ;
#11091=CARTESIAN_POINT ( 'NONE',  ( 15.96677753504215858, 136.6227766016837961, 4.434194661153730915E-13 ) ) ;
#11092=CARTESIAN_POINT ( 'NONE',  ( 16.01769397135268491, 136.8393535285714506, 3.937079669079953437 ) ) ;
#11099=CARTESIAN_POINT ( 'NONE',  ( -40.00000000000000000, 20.00000000000000000, 0.000000000000000000 ) ) ;
#11100=CARTESIAN_POINT ( 'NONE',  ( 17.56962100350864375, 125.3109322897003608, 3.333333333333324600 ) ) ;
#11102=CARTESIAN_POINT ( 'NONE',  ( 30.00000000000001066, 146.6227766016838245, 10.00000000000000178 ) ) ;
#11103=ADVANCED_FACE ( 'NONE', ( #10720 ), #5228, .F. ) ;
#11111=ORIENTED_EDGE ( 'NONE', *, *, #2329, .F. ) ;
#11116=EDGE_LOOP ( 'NONE', ( #8830, #13428, #8626, #1050 ) ) ;
#11119=LINE ( 'NONE', #7060, #8439 ) ;
#11122=CARTESIAN_POINT ( 'NONE',  ( 32.94787740378740892, 142.5723011982436788, 15.66001370690270633 ) ) ;
#11123=LINE ( 'NONE', #154, #16109 ) ;
#11124=CARTESIAN_POINT ( 'NONE',  ( -22.99999999999999645, 90.00000000000000000, 0.000000000000000000 ) ) ;
#11130=SHAPE_REPRESENTATION_RELATIONSHIP ( 'NONE' , 'NONE' ,  #16423, #5730 ) ;
#11132=DIRECTION ( 'NONE',  ( 1.000000000000000000, 0.000000000000000000, 0.000000000000000000 ) ) ;
#11133=CARTESIAN_POINT ( 'NONE',  ( 29.22485437292392518, 191.6792914357319546, 26.20566807848922153 ) ) ;
#11137=CARTESIAN_POINT ( 'NONE',  ( -43.00000000000001421, 125.3137084989847665, 13.00000000000000178 ) ) ;
#11138=CARTESIAN_POINT ( 'NONE',  ( -82.08787771659024202, 201.1698135001049934, 14.69689982759750535 ) ) ;
#11144=CARTESIAN_POINT ( 'NONE',  ( -34.99999999999999289, 130.0000000000000000, 0.000000000000000000 ) ) ;
#11145=DIRECTION ( 'NONE',  ( 0.000000000000000000, 0.000000000000000000, -1.000000000000000000 ) ) ;
#11158=CARTESIAN_POINT ( 'NONE',  ( -3.000000000000000888, 191.6227766016837961, -1.224646799147353454E-15 ) ) ;
#11161=VERTEX_POINT ( 'NONE', #15041 ) ;
#11162=LINE ( 'NONE', #3206, #810 ) ;
#11165=VERTEX_POINT ( 'NONE', #4433 ) ;
#11169=VECTOR ( 'NONE', #9768, 1000.000000000000000 ) ;
#11170=ORIENTED_EDGE ( 'NONE', *, *, #10879, .T. ) ;
#11173=EDGE_LOOP ( 'NONE', ( #16415, #1059, #354, #8785 ) ) ;
#11176=CARTESIAN_POINT ( 'NONE',  ( 22.72753210816244618, 139.3086630800672765, 13.45249220522710232 ) ) ;
#11182=CARTESIAN_POINT ( 'NONE',  ( -95.00000000000000000, 171.6227766016838245, 0.000000000000000000 ) ) ;
#11183=VECTOR ( 'NONE', #8644, 1000.000000000000000 ) ;
#11184=CARTESIAN_POINT ( 'NONE',  ( -77.42411652054217086, 192.3210352480456606, 25.70268529851927752 ) ) ;
#11186=CARTESIAN_POINT ( 'NONE',  ( 17.14315908062561533, 17.99999999999943157, 12.73566125713464636 ) ) ;
#11191=CARTESIAN_POINT ( 'NONE',  ( -34.99999999999999289, 130.0000000000000000, 15.00000000000000000 ) ) ;
#11193=ORIENTED_EDGE ( 'NONE', *, *, #7378, .T. ) ;
#11201=EDGE_CURVE ( 'NONE', #10746, #7694, #7426, .T. ) ;
#11202=LINE ( 'NONE', #16715, #5391 ) ;
#11208=CIRCLE ( 'NONE', #13481, 2.500000000000000444 ) ;
#11211=CARTESIAN_POINT ( 'NONE',  ( 30.23275679183038278, 141.6224873770942736, 13.74709594552941994 ) ) ;
#11216=MANIFOLD_SOLID_BREP ( 'Boss-Extrude6', #1868 ) ;
#11219=PLANE ( 'NONE',  #2555 ) ;
#11220=ORIENTED_EDGE ( 'NONE', *, *, #11264, .F. ) ;
#11225=VECTOR ( 'NONE', #7459, 1000.000000000000114 ) ;
#11230=CARTESIAN_POINT ( 'NONE',  ( -82.50000000000001421, 196.6227766016838245, 10.00000000000000178 ) ) ;
#11232=CARTESIAN_POINT ( 'NONE',  ( -48.00000000000000000, 154.3022685259950038, 9.999999999999900524 ) ) ;
#11233=CARTESIAN_POINT ( 'NONE',  ( 16.17028938446068764, 143.0439382767918346, 16.49999999999050360 ) ) ;
#11234=CARTESIAN_POINT ( 'NONE',  ( -81.55989001854683806, 201.3777828775944556, 14.27084532960631158 ) ) ;
#11238=ORIENTED_EDGE ( 'NONE', *, *, #7920, .T. ) ;
#11239=FACE_OUTER_BOUND ( 'NONE', #1435, .T. ) ;
#11244=CARTESIAN_POINT ( 'NONE',  ( -15.18548748502429468, 20.00000000000000000, 6.873064813191830602 ) ) ;
#11249=CARTESIAN_POINT ( 'NONE',  ( -23.65835920965563233, 18.00000000000000000, 17.33937328557891533 ) ) ;
#11250=CIRCLE ( 'NONE', #9553, 12.00000000000000000 ) ;
#11254=DIRECTION ( 'NONE',  ( 1.000000000000000000, 0.000000000000000000, 0.000000000000000000 ) ) ;
#11255=DIRECTION ( 'NONE',  ( -0.000000000000000000, -0.000000000000000000, 1.000000000000000000 ) ) ;
#11256=DIRECTION ( 'NONE',  ( -1.000000000000000000, 0.000000000000000000, 0.000000000000000000 ) ) ;
#11257=ORIENTED_EDGE ( 'NONE', *, *, #12303, .F. ) ;
#11258=DIRECTION ( 'NONE',  ( 1.000000000000000000, 0.000000000000000000, 0.000000000000000000 ) ) ;
#11260=FACE_OUTER_BOUND ( 'NONE', #3657, .T. ) ;
#11261=PLANE ( 'NONE',  #12603 ) ;
#11264=EDGE_CURVE ( 'NONE', #5481, #13477, #2646, .T. ) ;
#11267=FACE_OUTER_BOUND ( 'NONE', #12153, .T. ) ;
#11268=CARTESIAN_POINT ( 'NONE',  ( 16.36928288456784131, 136.8619714623083610, 5.700917076122240523 ) ) ;
#11272=AXIS2_PLACEMENT_3D ( 'NONE', #8457, #13952, #317 ) ;
#11279=CARTESIAN_POINT ( 'NONE',  ( 20.42763382733058108, 18.00000000000000000, 24.23318166603144164 ) ) ;
#11280=VECTOR ( 'NONE', #5696, 1000.000000000000000 ) ;
#11282=AXIS2_PLACEMENT_3D ( 'NONE', #6865, #4119, #9678 ) ;
#11283=ORIENTED_EDGE ( 'NONE', *, *, #4377, .F. ) ;
#11285=CARTESIAN_POINT ( 'NONE',  ( -27.98221281347037959, 19.99999999999999645, 0.000000000000000000 ) ) ;
#11286=ORIENTED_EDGE ( 'NONE', *, *, #11900, .F. ) ;
#11287=CARTESIAN_POINT ( 'NONE',  ( 15.00000000000000000, 154.3022685259950038, 9.999999999999900524 ) ) ;
#11290=VERTEX_POINT ( 'NONE', #3987 ) ;
#11292=AXIS2_PLACEMENT_3D ( 'NONE', #12665, #6281, #17004 ) ;
#11294=CARTESIAN_POINT ( 'NONE',  ( 9.072488053085830728, 140.2836875516620978, 12.31648485192419784 ) ) ;
#11299=CYLINDRICAL_SURFACE ( 'NONE', #10192, 5.000000000000000888 ) ;
#11300=CARTESIAN_POINT ( 'NONE',  ( 39.99999999999998579, 0.000000000000000000, 33.00000000000000711 ) ) ;
#11304=CARTESIAN_POINT ( 'NONE',  ( 26.56787054652181013, 142.9736659102427723, 16.38272693053711038 ) ) ;
#11307=CARTESIAN_POINT ( 'NONE',  ( -50.00000000000000000, 206.6227766016838245, -2.143131898507868248E-15 ) ) ;
#11313=CARTESIAN_POINT ( 'NONE',  ( -80.00000000000001421, 196.6227766016838245, 0.000000000000000000 ) ) ;
#11315=FACE_OUTER_BOUND ( 'NONE', #7632, .T. ) ;
#11320=B_SPLINE_CURVE_WITH_KNOTS ( 'NONE', 3,
 ( #9360, #13351, #2553, #8021, #17061, #11738, #12012, #10589, #11922, #7674, #14414, #13433, #5116, #11657, #2280, #13083, #949, #10414, #3881, #7946, #15911, #3702, #14495, #17240, #2363, #7754, #13168, #9175, #1038, #6438, #11831, #14581, #7851, #13261, #11035, #6879, #1399, #12366 ),
 .UNSPECIFIED., .F., .F.,
 ( 4, 2, 2, 2, 2, 2, 2, 2, 2, 2, 2, 2, 2, 2, 2, 2, 2, 2, 4 ),
 ( 0.01870878530979003598, 0.02011211734399856454, 0.02151544937820709658, 0.02432211344662422309, 0.02572544548083275859, 0.02712877751504130103, 0.02783044353214558092, 0.02853210954924986081, 0.02923377556635414765, 0.02993544158345842754, 0.03063710760056271090, 0.03133877361766699426, 0.03204043963477128110, 0.03274210565187556099, 0.03414543768608409302, 0.03554876972029263199, 0.03695210175450117096, 0.03835543378870970299, 0.04116209785712676705 ),
 .UNSPECIFIED. ) ;
#11321=LINE ( 'NONE', #4679, #11873 ) ;
#11328=DIRECTION ( 'NONE',  ( 1.000000000000000000, 0.000000000000000000, 0.000000000000000000 ) ) ;
#11329=CARTESIAN_POINT ( 'NONE',  ( -34.99999999999999289, 122.0000000000000284, 4.999999999999999112 ) ) ;
#11330=CARTESIAN_POINT ( 'NONE',  ( -75.41000427951827589, 198.6265692133321181, 18.97388360722737843 ) ) ;
#11331=VERTEX_POINT ( 'NONE', #5473 ) ;
#11332=AXIS2_PLACEMENT_3D ( 'NONE', #16865, #6234, #3490 ) ;
#11333=EDGE_CURVE ( 'NONE', #15131, #4289, #16277, .T. ) ;
#11334=EDGE_CURVE ( 'NONE', #1967, #14287, #512, .T. ) ;
#11340=CARTESIAN_POINT ( 'NONE',  ( 49.99999999999998579, 159.6227766016838814, 8.071800142134975431 ) ) ;
#11341=CARTESIAN_POINT ( 'NONE',  ( 48.00000000000000711, 175.6227766016838245, 5.571800142134975431 ) ) ;
#11343=CARTESIAN_POINT ( 'NONE',  ( 17.00000000000000000, 171.6227766016838245, 0.000000000000000000 ) ) ;
#11344=AXIS2_PLACEMENT_3D ( 'NONE', #2534, #7926, #1379 ) ;
#11345=CARTESIAN_POINT ( 'NONE',  ( -27.29618490519992591, 18.00000000000000000, 10.29570512375934044 ) ) ;
#11346=DIRECTION ( 'NONE',  ( 0.000000000000000000, 0.000000000000000000, -1.000000000000000000 ) ) ;
#11349=DIRECTION ( 'NONE',  ( -1.000000000000000000, -0.000000000000000000, -0.000000000000000000 ) ) ;
#11351=ORIENTED_EDGE ( 'NONE', *, *, #16954, .T. ) ;
#11353=ORIENTED_EDGE ( 'NONE', *, *, #13237, .F. ) ;
#11358=CARTESIAN_POINT ( 'NONE',  ( 21.38845554303141938, 19.99999999999999289, 23.94082098111162082 ) ) ;
#11359=CARTESIAN_POINT ( 'NONE',  ( 32.29171157738787912, 19.99999999999999645, 15.02090973094133375 ) ) ;
#11360=CARTESIAN_POINT ( 'NONE',  ( 27.42233524417435930, 136.9585154912620908, 4.953423069178740867 ) ) ;
#11361=EDGE_LOOP ( 'NONE', ( #11562, #3027, #10640, #5799 ) ) ;
#11362=CARTESIAN_POINT ( 'NONE',  ( 15.00000000000000000, 171.6227766016838245, 0.000000000000000000 ) ) ;
#11369=FACE_OUTER_BOUND ( 'NONE', #11361, .T. ) ;
#11370=EDGE_CURVE ( 'NONE', #5417, #14253, #7210, .T. ) ;
#11378=ORIENTED_EDGE ( 'NONE', *, *, #2565, .F. ) ;
#11381=ORIENTED_EDGE ( 'NONE', *, *, #14888, .F. ) ;
#11386=CARTESIAN_POINT ( 'NONE',  ( 12.84413890157916782, 129.3215245152910313, 10.42375118840982573 ) ) ;
#11390=CARTESIAN_POINT ( 'NONE',  ( 28.27146593557246490, 141.9273338169157341, 14.39467838667815691 ) ) ;
#11392=CYLINDRICAL_SURFACE ( 'NONE', #13877, 2.500000000000000444 ) ;
#11397=CARTESIAN_POINT ( 'NONE',  ( -68.00000000000000000, 191.6227766016837961, -1.224646799147353454E-15 ) ) ;
#11403=EDGE_CURVE ( 'NONE', #11501, #2395, #734, .T. ) ;
#11407=CARTESIAN_POINT ( 'NONE',  ( 27.99999999999998224, 9.999999999999998224, 0.000000000000000000 ) ) ;
#11408=CARTESIAN_POINT ( 'NONE',  ( -76.57310389028062048, 200.2770367110204006, 16.37379161636571823 ) ) ;
#11409=ORIENTED_EDGE ( 'NONE', *, *, #6417, .F. ) ;
#11412=DIRECTION ( 'NONE',  ( -1.000000000000000000, 0.000000000000000000, 0.000000000000000000 ) ) ;
#11419=CARTESIAN_POINT ( 'NONE',  ( -13.90980987654338286, 18.00000000000000355, 23.98326992096529864 ) ) ;
#11422=EDGE_CURVE ( 'NONE', #5356, #3326, #16635, .T. ) ;
#11426=CARTESIAN_POINT ( 'NONE',  ( -11.48222079042285770, 18.00000000000000355, 9.976350980977374050 ) ) ;
#11427=AXIS2_PLACEMENT_3D ( 'NONE', #14271, #1171, #9126 ) ;
#11429=CARTESIAN_POINT ( 'NONE',  ( -34.99999999999999289, 122.0000000000000284, 15.00000000000000000 ) ) ;
#11432=ORIENTED_EDGE ( 'NONE', *, *, #2331, .T. ) ;
#11439=CARTESIAN_POINT ( 'NONE',  ( 21.03709756577793399, 29.91885446100015145, 12.94894061605241831 ) ) ;
#11441=ORIENTED_EDGE ( 'NONE', *, *, #1487, .F. ) ;
#11443=EDGE_CURVE ( 'NONE', #9736, #11646, #4922, .T. ) ;
#11446=CARTESIAN_POINT ( 'NONE',  ( -81.34794908311457107, 191.8039921295446106, 26.10980206683226967 ) ) ;
#11449=CARTESIAN_POINT ( 'NONE',  ( -25.49999999999998579, 10.00000000000000000, 10.00000000000000178 ) ) ;
#11450=CIRCLE ( 'NONE', #12869, 25.00000000000000000 ) ;
#11456=DIRECTION ( 'NONE',  ( 0.000000000000000000, 0.000000000000000000, -1.000000000000000000 ) ) ;
#11459=EDGE_LOOP ( 'NONE', ( #4112, #10159, #12074, #870 ) ) ;
#11461=VERTEX_POINT ( 'NONE', #12815 ) ;
#11467=CARTESIAN_POINT ( 'NONE',  ( 10.69994788061133129, 131.5490474681699880, 11.88030112651796877 ) ) ;
#11470=DIRECTION ( 'NONE',  ( -0.000000000000000000, -0.000000000000000000, -1.000000000000000000 ) ) ;
#11472=CARTESIAN_POINT ( 'NONE',  ( 25.81930071191963805, 143.8651737624333578, 17.85267748742823812 ) ) ;
#11474=FACE_OUTER_BOUND ( 'NONE', #9781, .T. ) ;
#11480=CONICAL_SURFACE ( 'NONE', #6688, 2.499999999999998668, 1.029744260000002187 ) ;
#11481=DIRECTION ( 'NONE',  ( 0.000000000000000000, 0.000000000000000000, -1.000000000000000000 ) ) ;
#11482=VERTEX_POINT ( 'NONE', #6004 ) ;
#11483=ADVANCED_FACE ( 'NONE', ( #14155 ), #2093, .T. ) ;
#11484=DIRECTION ( 'NONE',  ( 0.000000000000000000, -1.000000000000000000, -1.836970198721028701E-16 ) ) ;
#11487=CARTESIAN_POINT ( 'NONE',  ( 15.72080254704531477, 141.4281235329943343, 17.70852598599439176 ) ) ;
#11490=VECTOR ( 'NONE', #5317, 1000.000000000000000 ) ;
#11495=VERTEX_POINT ( 'NONE', #7413 ) ;
#11501=VERTEX_POINT ( 'NONE', #6259 ) ;
#11505=EDGE_LOOP ( 'NONE', ( #536, #14135, #2082, #3471 ) ) ;
#11510=EDGE_LOOP ( 'NONE', ( #9258, #8772, #3553 ) ) ;
#11514=CARTESIAN_POINT ( 'NONE',  ( -9.672962866393921999, 30.74839102026217574, 12.74052981562734388 ) ) ;
#11516=CARTESIAN_POINT ( 'NONE',  ( -125.0000000000000000, 206.6227766016838245, 0.000000000000000000 ) ) ;
#11517=( GEOMETRIC_REPRESENTATION_CONTEXT ( 3 ) GLOBAL_UNCERTAINTY_ASSIGNED_CONTEXT ( ( #11932 ) ) GLOBAL_UNIT_ASSIGNED_CONTEXT ( ( #16549, #2910, #2742 ) ) REPRESENTATION_CONTEXT ( 'NONE', 'WORKASPACE' ) );
#11519=ORIENTED_EDGE ( 'NONE', *, *, #11073, .F. ) ;
#11523=EDGE_CURVE ( 'NONE', #12351, #11917, #16888, .T. ) ;
#11525=EDGE_CURVE ( 'NONE', #8489, #6919, #8642, .T. ) ;
#11527=CARTESIAN_POINT ( 'NONE',  ( 29.98123639043839006, 19.99999999999999645, 18.19121573219640098 ) ) ;
#11529=CARTESIAN_POINT ( 'NONE',  ( 33.88365274872861477, 19.99999999999999645, 11.43011099234506212 ) ) ;
#11530=CARTESIAN_POINT ( 'NONE',  ( 30.00000000000000355, 196.6227766016838245, 10.00000000000000178 ) ) ;
#11533=VERTEX_POINT ( 'NONE', #2272 ) ;
#11535=CARTESIAN_POINT ( 'NONE',  ( 48.00000000000000000, 171.6227766016838245, 0.000000000000000000 ) ) ;
#11540=DIRECTION ( 'NONE',  ( -1.000000000000000000, -0.000000000000000000, -0.000000000000000000 ) ) ;
#11542=DIRECTION ( 'NONE',  ( 0.8571673013836870192, 1.049727191973306873E-16, -0.5150380737757234151 ) ) ;
#11548=VERTEX_POINT ( 'NONE', #11568 ) ;
#11550=ORIENTED_EDGE ( 'NONE', *, *, #17518, .T. ) ;
#11552=ORIENTED_EDGE ( 'NONE', *, *, #7801, .F. ) ;
#11553=ORIENTED_EDGE ( 'NONE', *, *, #10790, .F. ) ;
#11555=VECTOR ( 'NONE', #5579, 1000.000000000000000 ) ;
#11558=TOROIDAL_SURFACE ( 'NONE', #2515, 740.0000000000000000, 8.000000000000000000 ) ;
#11559=CARTESIAN_POINT ( 'NONE',  ( 10.21857696054809317, 131.9747203951183110, 12.11181647197579636 ) ) ;
#11561=DIRECTION ( 'NONE',  ( 0.000000000000000000, 0.000000000000000000, 1.000000000000000000 ) ) ;
#11562=ORIENTED_EDGE ( 'NONE', *, *, #11900, .T. ) ;
#11563=CARTESIAN_POINT ( 'NONE',  ( 23.20616110506447072, 140.9816209840972192, 12.26578303444138207 ) ) ;
#11566=ADVANCED_FACE ( 'NONE', ( #17136 ), #14067, .T. ) ;
#11568=CARTESIAN_POINT ( 'NONE',  ( 15.56337975240373872, 125.2134999403456135, 4.999999999999997335 ) ) ;
#11571=FACE_OUTER_BOUND ( 'NONE', #4741, .T. ) ;
#11573=DIRECTION ( 'NONE',  ( -0.000000000000000000, -0.000000000000000000, -1.000000000000000000 ) ) ;
#11576=CARTESIAN_POINT ( 'NONE',  ( 12.22466323754103001, 142.0699085367067767, 18.75233045409083843 ) ) ;
#11580=AXIS2_PLACEMENT_3D ( 'NONE', #1151, #3803, #2382 ) ;
#11582=DIRECTION ( 'NONE',  ( 0.000000000000000000, 0.000000000000000000, 1.000000000000000000 ) ) ;
#11585=DIRECTION ( 'NONE',  ( 0.000000000000000000, 1.387778780781445676E-14, -1.000000000000000000 ) ) ;
#11586=ADVANCED_FACE ( 'NONE', ( #1390 ), #2543, .F. ) ;
#11590=ORIENTED_EDGE ( 'NONE', *, *, #5921, .T. ) ;
#11594=DIRECTION ( 'NONE',  ( -1.000000000000000000, -0.000000000000000000, -0.000000000000000000 ) ) ;
#11595=ORIENTED_EDGE ( 'NONE', *, *, #8453, .T. ) ;
#11597=CIRCLE ( 'NONE', #12175, 8.000000000000000000 ) ;
#11598=EDGE_CURVE ( 'NONE', #15841, #14845, #7841, .T. ) ;
#11599=LINE ( 'NONE', #8929, #12892 ) ;
#11601=DIRECTION ( 'NONE',  ( 1.000000000000000000, 0.000000000000000000, 0.000000000000000000 ) ) ;
#11604=VECTOR ( 'NONE', #11018, 1000.000000000000000 ) ;
#11605=CARTESIAN_POINT ( 'NONE',  ( -11.99122994684827503, 18.00000000000000000, 24.50500383881282573 ) ) ;
#11607=CIRCLE ( 'NONE', #6242, 2.500000000000002220 ) ;
#11608=LINE ( 'NONE', #7702, #6649 ) ;
#11615=ORIENTED_EDGE ( 'NONE', *, *, #12350, .T. ) ;
#11618=CIRCLE ( 'NONE', #6544, 10.00000000000000178 ) ;
#11619=CARTESIAN_POINT ( 'NONE',  ( 29.97257796258477569, 19.99999999999999645, 18.20111186907413270 ) ) ;
#11623=ADVANCED_FACE ( 'NONE', ( #15990, #7937 ), #59, .T. ) ;
#11635=CARTESIAN_POINT ( 'NONE',  ( 196.0000000000000000, 151.6227766016839098, 3.071800142134974099 ) ) ;
#11640=CYLINDRICAL_SURFACE ( 'NONE', #264, 5.000000000000004441 ) ;
#11641=EDGE_CURVE ( 'NONE', #9733, #4462, #11914, .T. ) ;
#11643=EDGE_CURVE ( 'NONE', #16355, #1583, #17319, .T. ) ;
#11645=EDGE_CURVE ( 'NONE', #12308, #12465, #5107, .T. ) ;
#11646=VERTEX_POINT ( 'NONE', #3872 ) ;
#11647=CARTESIAN_POINT ( 'NONE',  ( -80.00000000000002842, 146.6227766016838245, 0.000000000000000000 ) ) ;
#11657=CARTESIAN_POINT ( 'NONE',  ( -78.28305234797585399, 141.9230918234059686, 14.38591257614910468 ) ) ;
#11660=VERTEX_POINT ( 'NONE', #9352 ) ;
#11663=DIRECTION ( 'NONE',  ( -1.000000000000000000, -0.000000000000000000, -0.000000000000000000 ) ) ;
#11669=EDGE_LOOP ( 'NONE', ( #4638, #3965, #12654, #2041 ) ) ;
#11670=FACE_OUTER_BOUND ( 'NONE', #15254, .T. ) ;
#11672=EDGE_LOOP ( 'NONE', ( #10989, #519 ) ) ;
#11674=EDGE_CURVE ( 'NONE', #2616, #12728, #10680, .T. ) ;
#11675=CIRCLE ( 'NONE', #1215, 5.000000000000000888 ) ;
#11676=DIRECTION ( 'NONE',  ( -1.000000000000000000, -0.000000000000000000, -0.000000000000000000 ) ) ;
#11678=CARTESIAN_POINT ( 'NONE',  ( -13.91527097789399292, 18.00000000000000000, 23.98152295253420618 ) ) ;
#11682=LINE ( 'NONE', #16930, #9567 ) ;
#11683=ORIENTED_EDGE ( 'NONE', *, *, #10374, .F. ) ;
#11684=DIRECTION ( 'NONE',  ( 0.000000000000000000, 0.000000000000000000, -1.000000000000000000 ) ) ;
#11685=DIRECTION ( 'NONE',  ( -1.000000000000000000, -6.938893903907228378E-16, 0.000000000000000000 ) ) ;
#11687=CARTESIAN_POINT ( 'NONE',  ( 32.91012024024373517, 19.99999999999999289, 13.86436652238006673 ) ) ;
#11688=CARTESIAN_POINT ( 'NONE',  ( 24.72170379509201865, 19.99999999999999289, 7.619165077983454104 ) ) ;
#11691=ORIENTED_EDGE ( 'NONE', *, *, #3514, .T. ) ;
#11692=AXIS2_PLACEMENT_3D ( 'NONE', #13758, #11090, #3211 ) ;
#11699=ADVANCED_FACE ( 'NONE', ( #11822 ), #14833, .T. ) ;
#11704=CARTESIAN_POINT ( 'NONE',  ( 30.00000000000001066, 146.6227766016838245, 0.000000000000000000 ) ) ;
#11705=AXIS2_PLACEMENT_3D ( 'NONE', #4280, #9661, #4358 ) ;
#11709=AXIS2_PLACEMENT_3D ( 'NONE', #6744, #16032, #5492 ) ;
#11715=CARTESIAN_POINT ( 'NONE',  ( 32.50000000000000711, 146.6227766016838245, 10.00000000000000178 ) ) ;
#11718=CARTESIAN_POINT ( 'NONE',  ( 23.03715179780268585, 17.99999999999999645, 6.069068567132035241 ) ) ;
#11720=EDGE_LOOP ( 'NONE', ( #12429, #13928, #6167, #3439 ) ) ;
#11721=CARTESIAN_POINT ( 'NONE',  ( -80.00000000000002842, 146.6227766016838245, 10.00000000000000178 ) ) ;
#11724=CARTESIAN_POINT ( 'NONE',  ( 15.59275333247216366, 29.99107914678833353, 15.00000000000000000 ) ) ;
#11727=CARTESIAN_POINT ( 'NONE',  ( 33.63737915383075716, 200.0658281092903223, 16.73852573662798804 ) ) ;
#11730=VECTOR ( 'NONE', #3601, 1000.000000000000000 ) ;
#11737=VERTEX_POINT ( 'NONE', #16353 ) ;
#11738=CARTESIAN_POINT ( 'NONE',  ( -75.51110111240549827, 144.3473407286824681, 18.59810793231919845 ) ) ;
#11742=TOROIDAL_SURFACE ( 'NONE', #6110, 25.00000000000000000, 8.000000000000000000 ) ;
#11746=CIRCLE ( 'NONE', #6383, 30.00000000000000000 ) ;
#11755=EDGE_CURVE ( 'NONE', #5268, #5381, #9475, .T. ) ;
#11756=ADVANCED_FACE ( 'NONE', ( #140 ), #4221, .T. ) ;
#11757=EDGE_LOOP ( 'NONE', ( #16809, #9087, #1397, #12053 ) ) ;
#11760=AXIS2_PLACEMENT_3D ( 'NONE', #5953, #16833, #11346 ) ;
#11762=VECTOR ( 'NONE', #10210, 1000.000000000000000 ) ;
#11763=CARTESIAN_POINT ( 'NONE',  ( 225.0000000000000000, 89.99999999999997158, 4.999999999999999112 ) ) ;
#11765=CARTESIAN_POINT ( 'NONE',  ( 33.76178337805616536, 193.3250171236886388, 24.86042266551077518 ) ) ;
#11767=DIRECTION ( 'NONE',  ( 0.000000000000000000, -1.000000000000000000, 0.000000000000000000 ) ) ;
#11768=CARTESIAN_POINT ( 'NONE',  ( -11.61061639343520824, 17.99999999999999645, 9.781492982398956926 ) ) ;
#11772=EDGE_LOOP ( 'NONE', ( #11519, #14241, #13468, #12419 ) ) ;
#11775=ORIENTED_EDGE ( 'NONE', *, *, #14312, .F. ) ;
#11776=EDGE_CURVE ( 'NONE', #6665, #16876, #12531, .T. ) ;
#11779=AXIS2_PLACEMENT_3D ( 'NONE', #14339, #2209, #3995 ) ;
#11781=ORIENTED_EDGE ( 'NONE', *, *, #15931, .T. ) ;
#11783=CARTESIAN_POINT ( 'NONE',  ( 14.28882419134376747, 138.6263508161794675, 3.987386623658552232 ) ) ;
#11785=ORIENTED_EDGE ( 'NONE', *, *, #15870, .F. ) ;
#11794=DIRECTION ( 'NONE',  ( 0.000000000000000000, 1.000000000000000000, 0.000000000000000000 ) ) ;
#11800=VECTOR ( 'NONE', #5818, 1000.000000000000000 ) ;
#11801=VERTEX_POINT ( 'NONE', #9606 ) ;
#11802=VERTEX_POINT ( 'NONE', #4309 ) ;
#11807=ORIENTED_EDGE ( 'NONE', *, *, #2565, .T. ) ;
#11810=DIRECTION ( 'NONE',  ( -0.000000000000000000, -0.000000000000000000, -1.000000000000000000 ) ) ;
#11811=CARTESIAN_POINT ( 'NONE',  ( 32.29171157743327569, 18.00000000000000000, 15.02090973096405158 ) ) ;
#11812=CARTESIAN_POINT ( 'NONE',  ( -85.00000000000002842, 146.6227766016838245, 21.54065922853802562 ) ) ;
#11813=CIRCLE ( 'NONE', #5888, 2.500000000000002220 ) ;
#11814=CIRCLE ( 'NONE', #9269, 27.69059892324149175 ) ;
#11815=ORIENTED_EDGE ( 'NONE', *, *, #10670, .F. ) ;
#11819=CARTESIAN_POINT ( 'NONE',  ( 34.42405209918207731, 18.00000000000000000, 9.535225002503356251 ) ) ;
#11822=FACE_OUTER_BOUND ( 'NONE', #13688, .T. ) ;
#11823=DIRECTION ( 'NONE',  ( 0.000000000000000000, 0.000000000000000000, 1.000000000000000000 ) ) ;
#11824=CIRCLE ( 'NONE', #12686, 2.500000000000000444 ) ;
#11828=DIRECTION ( 'NONE',  ( 0.000000000000000000, 0.000000000000000000, 1.000000000000000000 ) ) ;
#11831=CARTESIAN_POINT ( 'NONE',  ( -83.64137593015411198, 143.1840127716920676, 16.74578779913499460 ) ) ;
#11832=CARTESIAN_POINT ( 'NONE',  ( 49.99999999999998579, 171.6227766016838245, 15.00000337241049131 ) ) ;
#11833=CARTESIAN_POINT ( 'NONE',  ( -43.00000000000000000, 140.0000000000000000, 15.00000000000000000 ) ) ;
#11838=CIRCLE ( 'NONE', #12421, 5.000000000000004441 ) ;
#11841=EDGE_CURVE ( 'NONE', #13780, #13530, #8363, .T. ) ;
#11846=VERTEX_POINT ( 'NONE', #8544 ) ;
#11852=ORIENTED_EDGE ( 'NONE', *, *, #2329, .T. ) ;
#11857=CARTESIAN_POINT ( 'NONE',  ( 33.41144845724742396, 192.9634543217044609, 25.17141653689332870 ) ) ;
#11858=DIRECTION ( 'NONE',  ( -1.000000000000000000, -0.000000000000000000, -0.000000000000000000 ) ) ;
#11860=CARTESIAN_POINT ( 'NONE',  ( -14.99999999999999467, 90.00000000000000000, 15.00000000000000000 ) ) ;
#11865=EDGE_CURVE ( 'NONE', #12308, #6571, #11746, .T. ) ;
#11871=ORIENTED_EDGE ( 'NONE', *, *, #394, .T. ) ;
#11873=VECTOR ( 'NONE', #15567, 1000.000000000000000 ) ;
#11875=VERTEX_POINT ( 'NONE', #14924 ) ;
#11877=CARTESIAN_POINT ( 'NONE',  ( 14.24852413927196970, 138.7494242586804489, 7.288003809479805639 ) ) ;
#11880=ORIENTED_EDGE ( 'NONE', *, *, #8773, .T. ) ;
#11881=AXIS2_PLACEMENT_3D ( 'NONE', #8089, #4115, #10837 ) ;
#11882=CARTESIAN_POINT ( 'NONE',  ( 17.00000000000000000, 171.6227766016838245, 0.000000000000000000 ) ) ;
#11886=ORIENTED_EDGE ( 'NONE', *, *, #11403, .T. ) ;
#11893=EDGE_LOOP ( 'NONE', ( #1527, #13994, #339, #7541, #7135 ) ) ;
#11895=DIRECTION ( 'NONE',  ( -1.000000000000000000, 0.000000000000000000, 0.000000000000000000 ) ) ;
#11896=ORIENTED_EDGE ( 'NONE', *, *, #4593, .F. ) ;
#11899=CARTESIAN_POINT ( 'NONE',  ( -7.379000772445021283, 30.00000000000000000, 13.00000000000000000 ) ) ;
#11900=EDGE_CURVE ( 'NONE', #13709, #12308, #10634, .T. ) ;
#11901=CARTESIAN_POINT ( 'NONE',  ( -13.49179905494335507, 31.33781166378165395, 13.29076615231557490 ) ) ;
#11905=CARTESIAN_POINT ( 'NONE',  ( 20.77386775082738879, 29.88392224133981401, 10.47448535043027462 ) ) ;
#11906=LINE ( 'NONE', #7571, #6089 ) ;
#11907=VERTEX_POINT ( 'NONE', #6061 ) ;
#11909=CARTESIAN_POINT ( 'NONE',  ( 0.000000000000000000, 0.000000000000000000, 0.000000000000000000 ) ) ;
#11910=CARTESIAN_POINT ( 'NONE',  ( 12.80996511848405994, 130.8496636614418094, 12.93682947221565804 ) ) ;
#11912=CARTESIAN_POINT ( 'NONE',  ( 22.45772829400591419, 29.90035839190693778, 11.59610751512981253 ) ) ;
#11913=EDGE_LOOP ( 'NONE', ( #10280, #2946, #16242 ) ) ;
#11914=LINE ( 'NONE', #13424, #7237 ) ;
#11917=VERTEX_POINT ( 'NONE', #3577 ) ;
#11920=EDGE_LOOP ( 'NONE', ( #12267, #1936, #3272, #14542, #186, #382, #14409 ) ) ;
#11922=CARTESIAN_POINT ( 'NONE',  ( -76.57381835343541354, 142.9679699711795990, 16.37278862731308493 ) ) ;
#11927=VERTEX_POINT ( 'NONE', #12710 ) ;
#11932=UNCERTAINTY_MEASURE_WITH_UNIT (LENGTH_MEASURE( 1.000000000000000082E-05 ), #16549, 'distance_accuracy_value', 'NONE');
#11933=EDGE_CURVE ( 'NONE', #11959, #15924, #2158, .T. ) ;
#11937=ORIENTED_EDGE ( 'NONE', *, *, #687, .F. ) ;
#11944=DIRECTION ( 'NONE',  ( -1.000000000000000000, 0.000000000000000000, 0.000000000000000000 ) ) ;
#11948=CARTESIAN_POINT ( 'NONE',  ( -77.50000000000002842, 146.6227766016838245, 10.00000000000000178 ) ) ;
#11949=DIRECTION ( 'NONE',  ( 0.000000000000000000, -0.000000000000000000, -1.000000000000000000 ) ) ;
#11951=FACE_OUTER_BOUND ( 'NONE', #13377, .T. ) ;
#11956=ORIENTED_EDGE ( 'NONE', *, *, #17330, .T. ) ;
#11957=CARTESIAN_POINT ( 'NONE',  ( -5.000000000000000888, 154.3022685259950038, 9.999999999999900524 ) ) ;
#11959=VERTEX_POINT ( 'NONE', #14132 ) ;
#11964=CARTESIAN_POINT ( 'NONE',  ( 12.95626684960129893, 129.1819364320672321, 10.30967895453046879 ) ) ;
#11965=EDGE_CURVE ( 'NONE', #7127, #10963, #17124, .T. ) ;
#11968=CARTESIAN_POINT ( 'NONE',  ( 17.52239125723112778, 29.96525225773407186, 14.66037399604394942 ) ) ;
#11971=DIRECTION ( 'NONE',  ( -1.000000000000000000, -0.000000000000000000, -0.000000000000000000 ) ) ;
#11972=LINE ( 'NONE', #2324, #1959 ) ;
#11976=CARTESIAN_POINT ( 'NONE',  ( 31.34525843090159825, 151.4423111973152061, 26.11038153352143709 ) ) ;
#11982=EDGE_LOOP ( 'NONE', ( #14671, #3675, #8064, #15909 ) ) ;
#11986=VERTEX_POINT ( 'NONE', #3845 ) ;
#11992=CARTESIAN_POINT ( 'NONE',  ( -78.47054368925184065, 151.3869516943736073, 26.06757126999134044 ) ) ;
#11997=LINE ( 'NONE', #3867, #832 ) ;
#12001=CARTESIAN_POINT ( 'NONE',  ( 22.23780067492955936, 29.90321370453013117, 11.83858959072850858 ) ) ;
#12006=DIRECTION ( 'NONE',  ( 0.8571673013836867971, 1.049727191973306626E-16, -0.5150380737757237481 ) ) ;
#12012=CARTESIAN_POINT ( 'NONE',  ( -75.79427778309866426, 143.8556217771935053, 17.85322440072383898 ) ) ;
#12015=CARTESIAN_POINT ( 'NONE',  ( -17.58288004918492931, 20.00000000000000355, 22.43027208364174285 ) ) ;
#12018=CARTESIAN_POINT ( 'NONE',  ( 9.156206820864191798, 144.1010407228830559, 18.21082046960973599 ) ) ;
#12021=VECTOR ( 'NONE', #5049, 1000.000000000000000 ) ;
#12022=VECTOR ( 'NONE', #6188, 1000.000000000000000 ) ;
#12023=EDGE_CURVE ( 'NONE', #12513, #9911, #16291, .T. ) ;
#12024=AXIS2_PLACEMENT_3D ( 'NONE', #7230, #15101, #7061 ) ;
#12027=PLANE ( 'NONE',  #1339 ) ;
#12031=ORIENTED_EDGE ( 'NONE', *, *, #13705, .F. ) ;
#12032=CARTESIAN_POINT ( 'NONE',  ( -27.99999999999998224, 10.00000000000000000, 10.00000000000000178 ) ) ;
#12034=EDGE_CURVE ( 'NONE', #13477, #2095, #9490, .T. ) ;
#12038=AXIS2_PLACEMENT_3D ( 'NONE', #8825, #2181, #16803 ) ;
#12039=CARTESIAN_POINT ( 'NONE',  ( -30.49999999999998224, 10.00000000000000000, 0.000000000000000000 ) ) ;
#12040=DIRECTION ( 'NONE',  ( 0.000000000000000000, 0.000000000000000000, -1.000000000000000000 ) ) ;
#12042=DIRECTION ( 'NONE',  ( 1.000000000000000000, -0.000000000000000000, -0.000000000000000000 ) ) ;
#12045=ORIENTED_EDGE ( 'NONE', *, *, #12411, .T. ) ;
#12048=DIRECTION ( 'NONE',  ( 0.000000000000000000, 0.000000000000000000, 1.000000000000000000 ) ) ;
#12051=CARTESIAN_POINT ( 'NONE',  ( -43.00000000000000000, 140.0000000000000000, 13.00000000000000000 ) ) ;
#12053=ORIENTED_EDGE ( 'NONE', *, *, #8845, .T. ) ;
#12054=CARTESIAN_POINT ( 'NONE',  ( -10.00647404944701258, 20.00000000000000000, 14.03129316391565951 ) ) ;
#12055=CARTESIAN_POINT ( 'NONE',  ( 26.76721132277178228, 139.3994271089711958, 7.121518580654788266 ) ) ;
#12064=AXIS2_PLACEMENT_3D ( 'NONE', #8355, #16778, #4643 ) ;
#12065=CARTESIAN_POINT ( 'NONE',  ( 49.99999999999998579, 163.6227766016838530, 12.50000337241049309 ) ) ;
#12066=VECTOR ( 'NONE', #9918, 1000.000000000000000 ) ;
#12068=CARTESIAN_POINT ( 'NONE',  ( 25.07772090985335467, 147.6670862717896000, 22.70911985051488458 ) ) ;
#12069=EDGE_CURVE ( 'NONE', #5481, #4609, #168, .T. ) ;
#12071=DIRECTION ( 'NONE',  ( 2.312964634635742464E-16, 0.000000000000000000, -1.000000000000000000 ) ) ;
#12072=PLANE ( 'NONE',  #8657 ) ;
#12074=ORIENTED_EDGE ( 'NONE', *, *, #1993, .T. ) ;
#12076=CIRCLE ( 'NONE', #16612, 20.00000000000000355 ) ;
#12079=CARTESIAN_POINT ( 'NONE',  ( 6.851232759387628768, 134.0993825829163200, 14.99999999999999822 ) ) ;
#12080=VECTOR ( 'NONE', #324, 1000.000000000000000 ) ;
#12087=CARTESIAN_POINT ( 'NONE',  ( -3.000000000000000888, 191.6227766016837961, -1.224646799147353454E-15 ) ) ;
#12089=CARTESIAN_POINT ( 'NONE',  ( -34.99999999999999289, 120.0000000000000284, 4.999999999999999112 ) ) ;
#12090=DIRECTION ( 'NONE',  ( 0.000000000000000000, 0.000000000000000000, -1.000000000000000000 ) ) ;
#12091=EDGE_CURVE ( 'NONE', #10963, #7127, #2429, .T. ) ;
#12092=EDGE_CURVE ( 'NONE', #8820, #13139, #9234, .T. ) ;
#12093=VECTOR ( 'NONE', #7595, 1000.000000000000000 ) ;
#12094=CARTESIAN_POINT ( 'NONE',  ( 17.54349574104648823, 125.4948194589026684, 4.999999999999997335 ) ) ;
#12097=CARTESIAN_POINT ( 'NONE',  ( 34.93420767853316988, 18.00000000000000355, 4.999999999999999112 ) ) ;
#12098=DIRECTION ( 'NONE',  ( -1.000000000000000000, 0.000000000000000000, 0.000000000000000000 ) ) ;
#12099=ADVANCED_FACE ( 'NONE', ( #13225 ), #12072, .T. ) ;
#12101=CARTESIAN_POINT ( 'NONE',  ( -22.99999999999999645, 100.0000000000000142, 15.00000000000000000 ) ) ;
#12104=ORIENTED_EDGE ( 'NONE', *, *, #8940, .F. ) ;
#12105=CARTESIAN_POINT ( 'NONE',  ( -90.80384757729339640, 171.6227766016838245, 0.000000000000000000 ) ) ;
#12109=AXIS2_PLACEMENT_3D ( 'NONE', #423, #9634, #4253 ) ;
#12114=CARTESIAN_POINT ( 'NONE',  ( -19.25702671965661850, 19.99999999999999645, 21.36300512502526416 ) ) ;
#12115=ORIENTED_EDGE ( 'NONE', *, *, #7648, .F. ) ;
#12117=CARTESIAN_POINT ( 'NONE',  ( 14.29542716350633214, 143.4273548044023698, 17.14909632368674508 ) ) ;
#12128=DIRECTION ( 'NONE',  ( -1.000000000000000000, 0.000000000000000000, 0.000000000000000000 ) ) ;
#12131=ADVANCED_FACE ( 'NONE', ( #13320 ), #11480, .F. ) ;
#12143=EDGE_LOOP ( 'NONE', ( #1274, #5585 ) ) ;
#12144=CARTESIAN_POINT ( 'NONE',  ( -18.25212770525996930, 32.30769230769230660, 15.00000000000000000 ) ) ;
#12150=CARTESIAN_POINT ( 'NONE',  ( -19.26597175465490963, 19.99999999999999645, 21.35691006828317384 ) ) ;
#12152=CARTESIAN_POINT ( 'NONE',  ( 14.50951369217283826, 138.6207054667691523, 6.378636156063609342 ) ) ;
#12153=EDGE_LOOP ( 'NONE', ( #12246, #8762, #2968, #9991 ) ) ;
#12155=VERTEX_POINT ( 'NONE', #16158 ) ;
#12163=CARTESIAN_POINT ( 'NONE',  ( 30.77905682277627619, 151.5769270156786206, 26.21405625665653005 ) ) ;
#12164=EDGE_LOOP ( 'NONE', ( #9495, #3057, #1790, #14507, #3228, #16161 ) ) ;
#12169=VERTEX_POINT ( 'NONE', #13493 ) ;
#12171=AXIS2_PLACEMENT_3D ( 'NONE', #11313, #15472, #6005 ) ;
#12172=AXIS2_PLACEMENT_3D ( 'NONE', #2269, #3432, #16886 ) ;
#12173=B_SPLINE_CURVE_WITH_KNOTS ( 'NONE', 3,
 ( #7419, #2027, #4511, #9900, #8662, #7338, #5927, #16647, #12821, #6091, #15305, #8569, #14073, #11487, #12910, #786, #11576, #16896, #8752, #3260, #13981, #12999 ),
 .UNSPECIFIED., .F., .F.,
 ( 4, 2, 2, 2, 2, 2, 2, 2, 2, 2, 4 ),
 ( 0.000000000000000000, 0.003698315653799323904, 0.007396631307598647807, 0.01109494696139797128, 0.01479326261519729561, 0.01664242044209697166, 0.01849157826899665291, 0.02218989392279601541, 0.02403905174969570360, 0.02588820957659539179, 0.02958652523039474735 ),
 .UNSPECIFIED. ) ;
#12174=CARTESIAN_POINT ( 'NONE',  ( 11.08062248138347528, 138.8595139650515193, 13.56485289974971842 ) ) ;
#12175=AXIS2_PLACEMENT_3D ( 'NONE', #2975, #6710, #16268 ) ;
#12176=ORIENTED_EDGE ( 'NONE', *, *, #10638, .F. ) ;
#12178=ADVANCED_FACE ( 'NONE', ( #4197 ), #6773, .F. ) ;
#12181=CARTESIAN_POINT ( 'NONE',  ( -3.000000000000002665, 142.8100939375178200, 16.63501009223129756 ) ) ;
#12183=CARTESIAN_POINT ( 'NONE',  ( -83.01610148909772136, 150.6144458722573063, 25.44936967851740306 ) ) ;
#12187=CARTESIAN_POINT ( 'NONE',  ( 17.51892952578853979, 125.6677330052578014, 5.783603459598163354 ) ) ;
#12188=CARTESIAN_POINT ( 'NONE',  ( 29.54149365486396661, 18.00000000000000355, 18.67620474358521676 ) ) ;
#12202=CARTESIAN_POINT ( 'NONE',  ( -27.94760966554430937, 19.99999999999999645, 6.338314452217975514 ) ) ;
#12204=CARTESIAN_POINT ( 'NONE',  ( 27.99999999999998224, 9.999999999999998224, 0.000000000000000000 ) ) ;
#12208=AXIS2_PLACEMENT_3D ( 'NONE', #9926, #16414, #16577 ) ;
#12210=VERTEX_POINT ( 'NONE', #1456 ) ;
#12222=FACE_OUTER_BOUND ( 'NONE', #6363, .T. ) ;
#12223=ORIENTED_EDGE ( 'NONE', *, *, #3538, .F. ) ;
#12229=EDGE_CURVE ( 'NONE', #15996, #3972, #9493, .T. ) ;
#12230=CARTESIAN_POINT ( 'NONE',  ( -16.58710929330769090, 31.97525413706907216, 10.34574908881256050 ) ) ;
#12231=CARTESIAN_POINT ( 'NONE',  ( -7.379000772444994638, 30.00000000000000000, 15.00000000000000000 ) ) ;
#12236=DIRECTION ( 'NONE',  ( 0.000000000000000000, 0.000000000000000000, -1.000000000000000000 ) ) ;
#12241=CARTESIAN_POINT ( 'NONE',  ( 28.08965273233581073, 151.2585272520459512, 25.96811968750270339 ) ) ;
#12242=ORIENTED_EDGE ( 'NONE', *, *, #5249, .F. ) ;
#12246=ORIENTED_EDGE ( 'NONE', *, *, #13208, .F. ) ;
#12247=ORIENTED_EDGE ( 'NONE', *, *, #4740, .T. ) ;
#12248=ADVANCED_FACE ( 'NONE', ( #5697, #8258, #39 ), #14901, .T. ) ;
#12249=CARTESIAN_POINT ( 'NONE',  ( 15.42236477930650906, 141.4984257577436892, 17.82510376534603580 ) ) ;
#12251=VERTEX_POINT ( 'NONE', #4286 ) ;
#12252=SHAPE_DEFINITION_REPRESENTATION ( #13651, #16423 ) ;
#12253=CARTESIAN_POINT ( 'NONE',  ( -45.00000000000001421, 124.1421356237309368, 15.00000000000000355 ) ) ;
#12257=B_SPLINE_CURVE_WITH_KNOTS ( 'NONE', 3,
 ( #16944, #4818, #10208, #655, #3405, #16776, #7201, #744, #14031, #3484, #10022, #15435, #3316, #8712, #11184, #476, #5880, #14277, #14120, #1987, #2148, #7388, #12785, #6052, #8798, #11446, #12521, #385, #16858, #14205, #8535, #2064, #7456, #12865, #16601, #4474, #9858, #15265, #3140, #13945 ),
 .UNSPECIFIED., .F., .F.,
 ( 4, 2, 2, 2, 2, 2, 2, 2, 2, 2, 2, 2, 2, 2, 2, 2, 2, 2, 2, 4 ),
 ( 0.02243093923957190788, 0.02359459467514175152, 0.02475825011071159515, 0.02592190554628143878, 0.02708556098185128241, 0.02766738869963622505, 0.02824921641742116421, 0.02941287185299101478, 0.03057652728856086188, 0.03115835500634581492, 0.03174018272413076797, 0.03232201044191572448, 0.03290383815970067405, 0.03348566587748562362, 0.03406749359527058013, 0.03523114903084052785, 0.03639480446641046862, 0.03755845990198040940, 0.03872211533755035018, 0.04104942620869018316 ),
 .UNSPECIFIED. ) ;
#12267=ORIENTED_EDGE ( 'NONE', *, *, #13239, .F. ) ;
#12270=DIRECTION ( 'NONE',  ( 0.000000000000000000, 0.000000000000000000, 1.000000000000000000 ) ) ;
#12279=CARTESIAN_POINT ( 'NONE',  ( -100.0000000000000000, 171.6227766016838245, 0.000000000000000000 ) ) ;
#12283=B_SPLINE_CURVE_WITH_KNOTS ( 'NONE', 3,
 ( #8537, #3223, #11100, #12699 ),
 .UNSPECIFIED., .F., .F.,
 ( 4, 4 ),
 ( 0.004999999999999983624, 0.009999999999999993269 ),
 .UNSPECIFIED. ) ;
#12286=CIRCLE ( 'NONE', #10014, 8.000000000000000000 ) ;
#12287=ORIENTED_EDGE ( 'NONE', *, *, #15962, .T. ) ;
#12288=FACE_BOUND ( 'NONE', #8187, .T. ) ;
#12293=DIRECTION ( 'NONE',  ( -1.000000000000000000, -0.000000000000000000, -0.000000000000000000 ) ) ;
#12297=CARTESIAN_POINT ( 'NONE',  ( -82.50000000000002842, 146.6227766016838245, 0.000000000000000000 ) ) ;
#12299=AXIS2_PLACEMENT_3D ( 'NONE', #13068, #7659, #11561 ) ;
#12303=EDGE_CURVE ( 'NONE', #254, #12210, #3805, .T. ) ;
#12304=EDGE_CURVE ( 'NONE', #13530, #16273, #5561, .T. ) ;
#12308=VERTEX_POINT ( 'NONE', #17175 ) ;
#12309=CARTESIAN_POINT ( 'NONE',  ( -15.09561842307794599, 19.99999999999308287, 7.342182892333040556 ) ) ;
#12311=AXIS2_PLACEMENT_3D ( 'NONE', #9963, #16794, #14222 ) ;
#12312=ORIENTED_EDGE ( 'NONE', *, *, #2937, .F. ) ;
#12313=AXIS2_PLACEMENT_3D ( 'NONE', #4591, #3080, #1755 ) ;
#12315=AXIS2_PLACEMENT_3D ( 'NONE', #14254, #15320, #6107 ) ;
#12316=( BOUNDED_SURFACE ( )  B_SPLINE_SURFACE ( 3, 2, ( 
 ( #15713, #9072, #14225 ),
 ( #5096, #4754, #10490 ),
 ( #14480, #2086, #14397 ),
 ( #6251, #3685, #15551 ) ),
 .UNSPECIFIED., .F., .F., .F. ) 
 B_SPLINE_SURFACE_WITH_KNOTS ( ( 4, 4 ),
 ( 3, 3 ),
 ( 0.1516087691302821228, 0.1566150273425061523 ),
 ( 0.000000000000000000, 1.000000000000000000 ),
 .UNSPECIFIED. ) 
 GEOMETRIC_REPRESENTATION_ITEM ( )  RATIONAL_B_SPLINE_SURFACE ( (
 ( 1.000000000000000000, 0.6556320892438535219, 1.000000000000000000),
 ( 1.000000000000000000, 0.6556321914870770762, 1.000000000000000000),
 ( 1.000000000000000000, 0.6556957163104851771, 1.000000000000000000),
 ( 1.000000000000000000, 0.6558243695371216431, 1.000000000000000000) ) ) 
 REPRESENTATION_ITEM ( '' )  SURFACE ( )  );
#12319=LINE ( 'NONE', #10990, #1323 ) ;
#12322=ORIENTED_EDGE ( 'NONE', *, *, #6415, .F. ) ;
#12323=FACE_OUTER_BOUND ( 'NONE', #8924, .T. ) ;
#12328=CARTESIAN_POINT ( 'NONE',  ( -80.00000000000001421, 196.6227766016838245, 0.000000000000000000 ) ) ;
#12332=DIRECTION ( 'NONE',  ( -1.000000000000000000, 0.000000000000000000, -8.673617379884037937E-17 ) ) ;
#12334=AXIS2_PLACEMENT_3D ( 'NONE', #4071, #9630, #15112 ) ;
#12335=ORIENTED_EDGE ( 'NONE', *, *, #10200, .F. ) ;
#12336=ORIENTED_EDGE ( 'NONE', *, *, #1919, .F. ) ;
#12337=CARTESIAN_POINT ( 'NONE',  ( 30.00000000000000355, 196.6227766016838245, 0.000000000000000000 ) ) ;
#12338=CYLINDRICAL_SURFACE ( 'NONE', #12940, 2.500000000000000444 ) ;
#12339=CARTESIAN_POINT ( 'NONE',  ( 12.97014296496520736, 138.3438685529228565, 12.30864880703445330 ) ) ;
#12340=CIRCLE ( 'NONE', #13762, 33.00000000000000000 ) ;
#12344=CARTESIAN_POINT ( 'NONE',  ( -45.00000000000000000, 130.0000000000000000, 15.00000000000000000 ) ) ;
#12345=FACE_OUTER_BOUND ( 'NONE', #5287, .T. ) ;
#12349=DIRECTION ( 'NONE',  ( 0.000000000000000000, 0.000000000000000000, 1.000000000000000000 ) ) ;
#12350=EDGE_CURVE ( 'NONE', #10830, #6313, #15453, .T. ) ;
#12351=VERTEX_POINT ( 'NONE', #13457 ) ;
#12354=FACE_OUTER_BOUND ( 'NONE', #15283, .T. ) ;
#12358=VECTOR ( 'NONE', #4337, 1000.000000000000000 ) ;
#12359=EDGE_CURVE ( 'NONE', #17318, #3061, #15854, .T. ) ;
#12362=LINE ( 'NONE', #8017, #14712 ) ;
#12366=CARTESIAN_POINT ( 'NONE',  ( -85.00000000000002842, 146.6227766016838245, 21.54065922853802562 ) ) ;
#12368=DIRECTION ( 'NONE',  ( 0.000000000000000000, 0.000000000000000000, -1.000000000000000000 ) ) ;
#12373=FACE_OUTER_BOUND ( 'NONE', #11772, .T. ) ;
#12374=FACE_BOUND ( 'NONE', #7885, .T. ) ;
#12381=AXIS2_PLACEMENT_3D ( 'NONE', #13985, #7081, #11132 ) ;
#12384=VERTEX_POINT ( 'NONE', #10800 ) ;
#12387=DIRECTION ( 'NONE',  ( 0.000000000000000000, 0.000000000000000000, -1.000000000000000000 ) ) ;
#12389=CARTESIAN_POINT ( 'NONE',  ( 39.99999999999998579, 4.000000000000000000, 33.00000000000000711 ) ) ;
#12392=CARTESIAN_POINT ( 'NONE',  ( -725.0000000000000000, 130.0000000000000000, 13.00000000000000000 ) ) ;
#12396=ORIENTED_EDGE ( 'NONE', *, *, #9808, .F. ) ;
#12397=LINE ( 'NONE', #16397, #13536 ) ;
#12398=ORIENTED_EDGE ( 'NONE', *, *, #10741, .F. ) ;
#12401=VERTEX_POINT ( 'NONE', #11948 ) ;
#12402=AXIS2_PLACEMENT_3D ( 'NONE', #9687, #9867, #15085 ) ;
#12403=CARTESIAN_POINT ( 'NONE',  ( -23.00000000000002132, 100.0000000000000142, 4.999999999999999112 ) ) ;
#12404=DIRECTION ( 'NONE',  ( -0.000000000000000000, -0.000000000000000000, -1.000000000000000000 ) ) ;
#12409=AXIS2_PLACEMENT_3D ( 'NONE', #10048, #10143, #14145 ) ;
#12411=EDGE_CURVE ( 'NONE', #11461, #8974, #17444, .T. ) ;
#12412=EDGE_CURVE ( 'NONE', #8580, #5427, #17349, .T. ) ;
#12418=DIRECTION ( 'NONE',  ( 0.000000000000000000, 0.000000000000000000, -1.000000000000000000 ) ) ;
#12419=ORIENTED_EDGE ( 'NONE', *, *, #16165, .T. ) ;
#12421=AXIS2_PLACEMENT_3D ( 'NONE', #3016, #8507, #13918 ) ;
#12424=ORIENTED_EDGE ( 'NONE', *, *, #1533, .F. ) ;
#12425=DIRECTION ( 'NONE',  ( 0.000000000000000000, 0.000000000000000000, 1.000000000000000000 ) ) ;
#12428=DIRECTION ( 'NONE',  ( -1.000000000000000000, -0.000000000000000000, -0.000000000000000000 ) ) ;
#12429=ORIENTED_EDGE ( 'NONE', *, *, #5159, .F. ) ;
#12430=ORIENTED_EDGE ( 'NONE', *, *, #2930, .T. ) ;
#12432=DIRECTION ( 'NONE',  ( 1.000000000000000000, 0.000000000000000000, 0.000000000000000000 ) ) ;
#12433=CARTESIAN_POINT ( 'NONE',  ( 19.90854668962809626, 140.2883655178033848, 15.59737012465792461 ) ) ;
#12436=DIRECTION ( 'NONE',  ( 0.000000000000000000, 0.000000000000000000, 1.000000000000000000 ) ) ;
#12437=CIRCLE ( 'NONE', #9610, 33.00000000000000000 ) ;
#12440=CARTESIAN_POINT ( 'NONE',  ( 15.60228996708978855, 124.9392590763941371, 1.671781470417840199 ) ) ;
#12442=EDGE_LOOP ( 'NONE', ( #17117, #1472, #17325, #12577 ) ) ;
#12443=DIRECTION ( 'NONE',  ( -1.000000000000000000, -0.000000000000000000, -0.000000000000000000 ) ) ;
#12447=DIRECTION ( 'NONE',  ( 0.8571673013836867971, 1.049727191973306626E-16, -0.5150380737757237481 ) ) ;
#12453=VECTOR ( 'NONE', #6803, 1000.000000000000000 ) ;
#12454=CARTESIAN_POINT ( 'NONE',  ( 13.53786153804126435, 143.5554826938402755, 17.35616514752890183 ) ) ;
#12455=VERTEX_POINT ( 'NONE', #4076 ) ;
#12462=VECTOR ( 'NONE', #13420, 1000.000000000000000 ) ;
#12465=VERTEX_POINT ( 'NONE', #5047 ) ;
#12468=CARTESIAN_POINT ( 'NONE',  ( -85.00000000000002842, 196.6227766016838245, 21.54065922853802562 ) ) ;
#12472=EDGE_CURVE ( 'NONE', #16355, #11917, #7261, .T. ) ;
#12475=ORIENTED_EDGE ( 'NONE', *, *, #6923, .F. ) ;
#12480=EDGE_CURVE ( 'NONE', #544, #1967, #15864, .T. ) ;
#12482=EDGE_CURVE ( 'NONE', #10010, #14157, #15118, .T. ) ;
#12483=CARTESIAN_POINT ( 'NONE',  ( -3.000000000000000888, 154.3022685259950038, 9.999999999999900524 ) ) ;
#12485=CARTESIAN_POINT ( 'NONE',  ( 48.00000000000000711, 167.6227766016838814, 21.92820660268601074 ) ) ;
#12486=CARTESIAN_POINT ( 'NONE',  ( -80.25919237425941333, 201.6174249061529054, 13.75941557453014497 ) ) ;
#12491=FACE_OUTER_BOUND ( 'NONE', #16790, .T. ) ;
#12496=ORIENTED_EDGE ( 'NONE', *, *, #5294, .F. ) ;
#12501=CARTESIAN_POINT ( 'NONE',  ( -77.50000000000002842, 146.6227766016838245, 0.000000000000000000 ) ) ;
#12502=CARTESIAN_POINT ( 'NONE',  ( -23.00000000000000000, 120.0000000000000284, 0.000000000000000000 ) ) ;
#12504=VERTEX_POINT ( 'NONE', #12389 ) ;
#12506=ORIENTED_EDGE ( 'NONE', *, *, #12350, .F. ) ;
#12507=DIRECTION ( 'NONE',  ( -0.000000000000000000, -1.000000000000000000, -0.000000000000000000 ) ) ;
#12511=ORIENTED_EDGE ( 'NONE', *, *, #12091, .F. ) ;
#12513=VERTEX_POINT ( 'NONE', #11230 ) ;
#12516=FACE_OUTER_BOUND ( 'NONE', #2840, .T. ) ;
#12517=CARTESIAN_POINT ( 'NONE',  ( 14.17453072134883030, 137.9246278893784847, 11.09209212451273707 ) ) ;
#12518=ORIENTED_EDGE ( 'NONE', *, *, #11598, .F. ) ;
#12519=LINE ( 'NONE', #9856, #13244 ) ;
#12520=CARTESIAN_POINT ( 'NONE',  ( -27.98221281347036893, 30.00000000000000355, 4.999999999999999112 ) ) ;
#12521=CARTESIAN_POINT ( 'NONE',  ( -81.53182587509584778, 191.8593874686152105, 26.06696055488265529 ) ) ;
#12522=CARTESIAN_POINT ( 'NONE',  ( 225.0000000000000000, 89.99999999999997158, 4.999999999999999112 ) ) ;
#12524=CARTESIAN_POINT ( 'NONE',  ( 14.93242934743710570, 18.00000000000000355, 12.99999999999999822 ) ) ;
#12525=DIRECTION ( 'NONE',  ( 0.000000000000000000, 0.000000000000000000, -1.000000000000000000 ) ) ;
#12526=EDGE_LOOP ( 'NONE', ( #3106, #958, #13123, #1643 ) ) ;
#12531=LINE ( 'NONE', #1738, #8076 ) ;
#12536=CARTESIAN_POINT ( 'NONE',  ( 8.147273376221958685, 133.4207317082267537, 12.78321197947435728 ) ) ;
#12537=ORIENTED_EDGE ( 'NONE', *, *, #14791, .T. ) ;
#12543=CARTESIAN_POINT ( 'NONE',  ( -16.30611068361787019, 32.76923076923078781, 0.000000000000000000 ) ) ;
#12563=CARTESIAN_POINT ( 'NONE',  ( -81.74336020400447467, 201.3127097690254175, 14.40604465277978541 ) ) ;
#12566=AXIS2_PLACEMENT_3D ( 'NONE', #1069, #6470, #9207 ) ;
#12571=DIRECTION ( 'NONE',  ( -0.000000000000000000, -0.000000000000000000, -1.000000000000000000 ) ) ;
#12576=CARTESIAN_POINT ( 'NONE',  ( 196.0000000000000000, 163.6227766016838530, 12.50000337241049309 ) ) ;
#12577=ORIENTED_EDGE ( 'NONE', *, *, #10165, .F. ) ;
#12579=AXIS2_PLACEMENT_3D ( 'NONE', #4876, #15856, #17177 ) ;
#12580=CARTESIAN_POINT ( 'NONE',  ( -12.63167751028164965, 18.00000000000000000, 24.35243221814330994 ) ) ;
#12581=VECTOR ( 'NONE', #8482, 1000.000000000000000 ) ;
#12584=FACE_OUTER_BOUND ( 'NONE', #2853, .T. ) ;
#12586=CARTESIAN_POINT ( 'NONE',  ( 17.00000000000000000, 171.6227766016838245, 0.000000000000000000 ) ) ;
#12592=DIRECTION ( 'NONE',  ( 0.000000000000000000, -1.000000000000000000, 6.123233995736762338E-17 ) ) ;
#12599=CARTESIAN_POINT ( 'NONE',  ( 14.91849273675205545, 128.9263856399286396, 11.14803070335530855 ) ) ;
#12603=AXIS2_PLACEMENT_3D ( 'NONE', #13587, #9668, #16425 ) ;
#12604=AXIS2_PLACEMENT_3D ( 'NONE', #10370, #10547, #2409 ) ;
#12608=CARTESIAN_POINT ( 'NONE',  ( 16.62686111071178630, 17.99999999999885603, 12.85442640772723344 ) ) ;
#12616=VERTEX_POINT ( 'NONE', #2344 ) ;
#12619=VECTOR ( 'NONE', #8593, 1000.000000000000000 ) ;
#12620=CARTESIAN_POINT ( 'NONE',  ( 8.904477399773945479, 144.1137579919043787, 18.22932967255391290 ) ) ;
#12623=ORIENTED_EDGE ( 'NONE', *, *, #3975, .F. ) ;
#12625=DIRECTION ( 'NONE',  ( -1.000000000000000000, 0.000000000000000000, 0.000000000000000000 ) ) ;
#12626=FACE_OUTER_BOUND ( 'NONE', #13691, .T. ) ;
#12628=ADVANCED_FACE ( 'NONE', ( #10489 ), #9939, .T. ) ;
#12630=EDGE_CURVE ( 'NONE', #978, #8489, #12283, .T. ) ;
#12634=ORIENTED_EDGE ( 'NONE', *, *, #9045, .T. ) ;
#12635=CARTESIAN_POINT ( 'NONE',  ( 32.50000000000000000, 196.6227766016838245, 10.00000000000000178 ) ) ;
#12643=EDGE_LOOP ( 'NONE', ( #15185, #3353 ) ) ;
#12648=DIRECTION ( 'NONE',  ( 0.000000000000000000, 0.000000000000000000, 1.000000000000000000 ) ) ;
#12652=CARTESIAN_POINT ( 'NONE',  ( 27.13959012325753406, 18.00000000000000000, 20.89788123228700556 ) ) ;
#12653=CARTESIAN_POINT ( 'NONE',  ( -22.99999999999998224, 10.00000000000000000, 28.00000000000000355 ) ) ;
#12654=ORIENTED_EDGE ( 'NONE', *, *, #12359, .T. ) ;
#12655=CARTESIAN_POINT ( 'NONE',  ( -80.00000000000002842, 146.6227766016838245, 0.000000000000000000 ) ) ;
#12656=CARTESIAN_POINT ( 'NONE',  ( 22.66773460012013430, 29.84724857135450193, 7.067878044979525320 ) ) ;
#12657=CARTESIAN_POINT ( 'NONE',  ( -76.36262084616922152, 200.0658281092903508, 16.73852573662796317 ) ) ;
#12658=ORIENTED_EDGE ( 'NONE', *, *, #16449, .T. ) ;
#12659=ORIENTED_EDGE ( 'NONE', *, *, #11422, .F. ) ;
#12661=AXIS2_PLACEMENT_3D ( 'NONE', #7918, #10386, #11895 ) ;
#12665=CARTESIAN_POINT ( 'NONE',  ( 49.99999999999998579, 167.6227766016838814, 19.42820660268601074 ) ) ;
#12666=EDGE_LOOP ( 'NONE', ( #10157, #1186, #10289, #6137 ) ) ;
#12667=EDGE_CURVE ( 'NONE', #9322, #9733, #6703, .T. ) ;
#12670=ADVANCED_FACE ( 'NONE', ( #1641 ), #13772, .F. ) ;
#12678=CARTESIAN_POINT ( 'NONE',  ( -48.00000000000000000, 191.6227766016837961, -1.224646799147353454E-15 ) ) ;
#12679=ADVANCED_FACE ( 'NONE', ( #312 ), #3318, .F. ) ;
#12682=FACE_OUTER_BOUND ( 'NONE', #16845, .T. ) ;
#12686=AXIS2_PLACEMENT_3D ( 'NONE', #179, #16802, #14066 ) ;
#12689=AXIS2_PLACEMENT_3D ( 'NONE', #1488, #6880, #12368 ) ;
#12690=DIRECTION ( 'NONE',  ( 0.000000000000000000, 0.000000000000000000, -1.000000000000000000 ) ) ;
#12691=CARTESIAN_POINT ( 'NONE',  ( 16.25737266305939599, 136.9911583880083015, 7.117438641153603918 ) ) ;
#12692=VERTEX_POINT ( 'NONE', #223 ) ;
#12694=CARTESIAN_POINT ( 'NONE',  ( 48.00000000000000711, 179.6227766016838245, 12.50000337241049309 ) ) ;
#12696=DIRECTION ( 'NONE',  ( -0.000000000000000000, 1.000000000000000000, 0.000000000000000000 ) ) ;
#12699=CARTESIAN_POINT ( 'NONE',  ( 17.54349574104648823, 125.4948194589026684, 4.999999999999997335 ) ) ;
#12703=AXIS2_PLACEMENT_3D ( 'NONE', #1087, #14458, #13218 ) ;
#12710=CARTESIAN_POINT ( 'NONE',  ( 22.93524650466160963, 29.84210526315773748, 4.999999999999999112 ) ) ;
#12711=ORIENTED_EDGE ( 'NONE', *, *, #14772, .T. ) ;
#12715=CARTESIAN_POINT ( 'NONE',  ( 9.414336857517209722, 132.5946763488762770, 12.41924194405873649 ) ) ;
#12717=AXIS2_PLACEMENT_3D ( 'NONE', #2493, #14716, #2592 ) ;
#12721=B_SPLINE_CURVE_WITH_KNOTS ( 'NONE', 3,
 ( #11812, #5006, #15807, #17218, #2434, #1113, #10571, #1471, #17312, #2621, #5453, #12183, #13333, #9249, #9600, #10669, #14826, #8007, #53, #2535, #3958, #10841, #16252, #16174, #11992, #3863, #5368, #14750, #13414, #13602, #4045, #10924, #13679, #17495, #10762, #1198, #8094, #4121, #9421, #17397, #9507, #8271 ),
 .UNSPECIFIED., .F., .F.,
 ( 4, 2, 2, 2, 2, 2, 2, 2, 2, 2, 2, 2, 2, 2, 2, 2, 2, 2, 2, 2, 4 ),
 ( 0.000000000000000000, 0.002338598163723741054, 0.002923247704654684340, 0.003507897245585628061, 0.004677196327447571446, 0.005846495409309514397, 0.006431144950240465057, 0.007015794491171416583, 0.008185093573033283207, 0.008769743113964226927, 0.009354392654895168913, 0.01052369173675701645, 0.01110834127768793762, 0.01169299081861886053, 0.01286228990048070633, 0.01403158898234255214, 0.01461623852327346637, 0.01520088806420438060, 0.01637018714606626457, 0.01753948622792815201, 0.01870878530979003598 ),
 .UNSPECIFIED. ) ;
#12725=CARTESIAN_POINT ( 'NONE',  ( 14.23753691287610579, 127.5498911642838635, 8.870798623635511859 ) ) ;
#12727=CARTESIAN_POINT ( 'NONE',  ( 49.99999999999998579, 183.6227766016837961, 3.071800142134975431 ) ) ;
#12728=VERTEX_POINT ( 'NONE', #11860 ) ;
#12729=CARTESIAN_POINT ( 'NONE',  ( 31.52965557968541432, 141.8580068101642269, 14.25043922611180136 ) ) ;
#12733=CARTESIAN_POINT ( 'NONE',  ( 50.00000000000000000, 171.6227766016838245, 0.000000000000000000 ) ) ;
#12736=FACE_OUTER_BOUND ( 'NONE', #2670, .T. ) ;
#12738=ADVANCED_FACE ( 'NONE', ( #9205 ), #6561, .T. ) ;
#12739=EDGE_CURVE ( 'NONE', #15148, #11161, #7881, .T. ) ;
#12741=LINE ( 'NONE', #7240, #15456 ) ;
#12742=AXIS2_PLACEMENT_3D ( 'NONE', #12576, #5762, #8155 ) ;
#12746=CIRCLE ( 'NONE', #11881, 2.500000000000002220 ) ;
#12748=FACE_OUTER_BOUND ( 'NONE', #16361, .T. ) ;
#12749=ORIENTED_EDGE ( 'NONE', *, *, #15325, .T. ) ;
#12752=CARTESIAN_POINT ( 'NONE',  ( -82.24876160832761229, 201.0919203481101363, 14.85271610579512114 ) ) ;
#12753=ORIENTED_EDGE ( 'NONE', *, *, #6786, .F. ) ;
#12754=VECTOR ( 'NONE', #5625, 1000.000000000000000 ) ;
#12755=EDGE_LOOP ( 'NONE', ( #7311, #15889, #6760, #6626 ) ) ;
#12756=DIRECTION ( 'NONE',  ( 1.000000000000000000, 0.000000000000000000, 8.673617379884036705E-17 ) ) ;
#12763=CARTESIAN_POINT ( 'NONE',  ( -27.99999999999998224, 10.00000000000000000, 28.00000000000000355 ) ) ;
#12765=CARTESIAN_POINT ( 'NONE',  ( 48.00000000000000711, 167.6227766016838814, 16.92820660268601429 ) ) ;
#12767=DIRECTION ( 'NONE',  ( 0.000000000000000000, 0.8660254037844413721, -0.4999999999999952816 ) ) ;
#12768=CARTESIAN_POINT ( 'NONE',  ( -27.84784281930893357, 18.00000000000000000, 7.647248539284095870 ) ) ;
#12769=LINE ( 'NONE', #11516, #13992 ) ;
#12771=ORIENTED_EDGE ( 'NONE', *, *, #17138, .T. ) ;
#12774=ADVANCED_FACE ( 'NONE', ( #11951 ), #17353, .F. ) ;
#12778=CARTESIAN_POINT ( 'NONE',  ( 16.25302816831168329, 19.99999999999999645, 25.00000000000000000 ) ) ;
#12779=CARTESIAN_POINT ( 'NONE',  ( 20.25331481973466907, 20.00000000000113687, 13.55662431013403868 ) ) ;
#12780=CARTESIAN_POINT ( 'NONE',  ( 12.82285603306638144, 130.8395207603766153, 12.92896204370639524 ) ) ;
#12784=DIRECTION ( 'NONE',  ( -1.000000000000000000, 0.000000000000000000, 0.000000000000000000 ) ) ;
#12785=CARTESIAN_POINT ( 'NONE',  ( -80.38335849529188692, 191.6335950462331823, 26.24057872661396118 ) ) ;
#12796=DIRECTION ( 'NONE',  ( -1.000000000000000000, 0.000000000000000000, 0.000000000000000000 ) ) ;
#12800=VERTEX_POINT ( 'NONE', #17270 ) ;
#12801=EDGE_CURVE ( 'NONE', #13379, #12251, #2584, .T. ) ;
#12802=DIRECTION ( 'NONE',  ( -1.000000000000000000, 0.000000000000000000, 0.000000000000000000 ) ) ;
#12806=FACE_OUTER_BOUND ( 'NONE', #15845, .T. ) ;
#12807=LINE ( 'NONE', #11300, #11183 ) ;
#12815=CARTESIAN_POINT ( 'NONE',  ( 49.99999999999998579, 167.6227766016838814, 16.92820660268601429 ) ) ;
#12821=CARTESIAN_POINT ( 'NONE',  ( 20.99355996702781724, 139.9415946336124534, 14.89340340269096785 ) ) ;
#12823=CYLINDRICAL_SURFACE ( 'NONE', #1816, 2.500000000000000444 ) ;
#12825=CARTESIAN_POINT ( 'NONE',  ( 22.93524650466160963, 29.84210526315773748, 15.00000000000000000 ) ) ;
#12826=DIRECTION ( 'NONE',  ( 0.000000000000000000, 0.000000000000000000, -1.000000000000000000 ) ) ;
#12836=FACE_OUTER_BOUND ( 'NONE', #402, .T. ) ;
#12837=LINE ( 'NONE', #17081, #5254 ) ;
#12843=CARTESIAN_POINT ( 'NONE',  ( 17.00000000000000000, 154.3022685259950038, 9.999999999999900524 ) ) ;
#12844=CARTESIAN_POINT ( 'NONE',  ( -9.480043248727735516, 17.99999999999769784, 11.96743332394513715 ) ) ;
#12845=ADVANCED_FACE ( 'NONE', ( #6647 ), #15749, .T. ) ;
#12848=EDGE_CURVE ( 'NONE', #2606, #15093, #8401, .T. ) ;
#12851=EDGE_LOOP ( 'NONE', ( #16186, #5232, #7301, #3494 ) ) ;
#12861=CYLINDRICAL_SURFACE ( 'NONE', #13519, 2.500000000000000444 ) ;
#12862=ORIENTED_EDGE ( 'NONE', *, *, #25, .F. ) ;
#12864=DIRECTION ( 'NONE',  ( 0.000000000000000000, 0.000000000000000000, 1.000000000000000000 ) ) ;
#12865=CARTESIAN_POINT ( 'NONE',  ( -84.06590298985813092, 193.6946896392257997, 24.53450862945289401 ) ) ;
#12869=AXIS2_PLACEMENT_3D ( 'NONE', #6620, #950, #6440 ) ;
#12874=ORIENTED_EDGE ( 'NONE', *, *, #6721, .T. ) ;
#12875=DIRECTION ( 'NONE',  ( 1.000000000000000000, -0.000000000000000000, -0.000000000000000000 ) ) ;
#12878=VERTEX_POINT ( 'NONE', #3003 ) ;
#12879=EDGE_LOOP ( 'NONE', ( #3917, #13662, #6215, #610, #16464 ) ) ;
#12881=ORIENTED_EDGE ( 'NONE', *, *, #12034, .T. ) ;
#12884=ORIENTED_EDGE ( 'NONE', *, *, #1233, .T. ) ;
#12891=( BOUNDED_CURVE ( )  B_SPLINE_CURVE ( 3, ( #7213, #16444, #4307, #6871 ),
 .UNSPECIFIED., .F., .F. ) 
 B_SPLINE_CURVE_WITH_KNOTS ( ( 4, 4 ),
 ( 1.570796326794899000, 3.141592653589791340 ),
 .UNSPECIFIED. ) 
 CURVE ( )  GEOMETRIC_REPRESENTATION_ITEM ( )  RATIONAL_B_SPLINE_CURVE ( ( 1.000000000000000000, 0.8047378541243659367, 0.8047378541243659367, 1.000000000000000000 ) ) 
 REPRESENTATION_ITEM ( '' )  );
#12892=VECTOR ( 'NONE', #715, 1000.000000000000000 ) ;
#12893=CARTESIAN_POINT ( 'NONE',  ( 49.99999999999998579, 167.6227766016838814, 19.42820660268601074 ) ) ;
#12898=DIRECTION ( 'NONE',  ( -0.000000000000000000, -0.000000000000000000, -1.000000000000000000 ) ) ;
#12899=ADVANCED_FACE ( 'NONE', ( #1687 ), #13818, .F. ) ;
#12903=CIRCLE ( 'NONE', #5546, 9.999999999999998224 ) ;
#12905=CARTESIAN_POINT ( 'NONE',  ( -27.99999999999998224, 10.00000000000000000, 35.00200000000000244 ) ) ;
#12906=ORIENTED_EDGE ( 'NONE', *, *, #10061, .T. ) ;
#12907=CARTESIAN_POINT ( 'NONE',  ( -3.000000000000000888, 204.6227766016838245, -2.020667218593133100E-15 ) ) ;
#12909=ORIENTED_EDGE ( 'NONE', *, *, #4926, .T. ) ;
#12910=CARTESIAN_POINT ( 'NONE',  ( 14.58358448378887928, 141.6717822189192191, 18.11319387340528309 ) ) ;
#12916=DIRECTION ( 'NONE',  ( -1.000000000000000000, -0.000000000000000000, -0.000000000000000000 ) ) ;
#12922=EDGE_LOOP ( 'NONE', ( #8872, #3469, #11590, #1636, #17130, #2925, #16665 ) ) ;
#12929=CARTESIAN_POINT ( 'NONE',  ( 30.00000000000001066, 146.6227766016838245, 35.00200000000000244 ) ) ;
#12935=CARTESIAN_POINT ( 'NONE',  ( -68.00000000000000000, 171.6227766016838245, 0.000000000000000000 ) ) ;
#12937=CARTESIAN_POINT ( 'NONE',  ( -10.50630597522742171, 31.01369813559846378, 12.50559288035636563 ) ) ;
#12939=CARTESIAN_POINT ( 'NONE',  ( -23.00000000000001421, 122.0000000000000284, 4.999999999999999112 ) ) ;
#12940=AXIS2_PLACEMENT_3D ( 'NONE', #11008, #2950, #3214 ) ;
#12943=EDGE_LOOP ( 'NONE', ( #13079, #5398 ) ) ;
#12946=CARTESIAN_POINT ( 'NONE',  ( 225.0000000000000000, 89.99999999999997158, 0.000000000000000000 ) ) ;
#12947=DIRECTION ( 'NONE',  ( 1.000000000000000000, 0.000000000000000000, 0.000000000000000000 ) ) ;
#12948=ORIENTED_EDGE ( 'NONE', *, *, #9211, .T. ) ;
#12949=CARTESIAN_POINT ( 'NONE',  ( 30.81698523721487604, 20.00000000000000355, 17.17210857557096659 ) ) ;
#12952=CIRCLE ( 'NONE', #14364, 2.499999999999998668 ) ;
#12953=CARTESIAN_POINT ( 'NONE',  ( 23.92105171931311958, 29.88144160311327724, 9.435928464502936208 ) ) ;
#12958=CYLINDRICAL_SURFACE ( 'NONE', #10425, 10.00000000000000000 ) ;
#12960=LINE ( 'NONE', #11449, #15656 ) ;
#12968=DIRECTION ( 'NONE',  ( -1.000000000000000000, 0.000000000000000000, 0.000000000000000000 ) ) ;
#12971=ORIENTED_EDGE ( 'NONE', *, *, #3347, .T. ) ;
#12972=LINE ( 'NONE', #11635, #6156 ) ;
#12973=VECTOR ( 'NONE', #14171, 1000.000000000000000 ) ;
#12976=AXIS2_PLACEMENT_3D ( 'NONE', #3413, #2074, #4738 ) ;
#12978=AXIS2_PLACEMENT_3D ( 'NONE', #9069, #14395, #2533 ) ;
#12981=CARTESIAN_POINT ( 'NONE',  ( 30.80964797964692536, 18.00000000000000000, 17.18170494867161224 ) ) ;
#12982=FACE_OUTER_BOUND ( 'NONE', #1628, .T. ) ;
#12989=CONICAL_SURFACE ( 'NONE', #9023, 2.500000000000002220, 1.029744260000002631 ) ;
#12992=AXIS2_PLACEMENT_3D ( 'NONE', #5781, #12432, #12690 ) ;
#12995=DIRECTION ( 'NONE',  ( -1.000000000000000000, -0.000000000000000000, -0.000000000000000000 ) ) ;
#12999=CARTESIAN_POINT ( 'NONE',  ( 6.134011831684053284, 142.5209969267753820, 19.44444444444444642 ) ) ;
#13003=AXIS2_PLACEMENT_3D ( 'NONE', #2586, #9463, #13464 ) ;
#13006=ORIENTED_EDGE ( 'NONE', *, *, #15704, .F. ) ;
#13008=DIRECTION ( 'NONE',  ( 1.000000000000000000, 0.000000000000000000, 0.000000000000000000 ) ) ;
#13009=CARTESIAN_POINT ( 'NONE',  ( -32.99999999999998579, 10.00000000000000000, 0.000000000000000000 ) ) ;
#13011=ORIENTED_EDGE ( 'NONE', *, *, #10246, .T. ) ;
#13012=ORIENTED_EDGE ( 'NONE', *, *, #4441, .F. ) ;
#13023=EDGE_LOOP ( 'NONE', ( #14448, #3974, #3623, #9994 ) ) ;
#13026=EDGE_CURVE ( 'NONE', #17370, #11034, #9905, .T. ) ;
#13027=DIRECTION ( 'NONE',  ( -0.000000000000000000, -0.000000000000000000, -1.000000000000000000 ) ) ;
#13029=CARTESIAN_POINT ( 'NONE',  ( -11.82448321327245466, 31.42688426858654438, 11.97038274549936254 ) ) ;
#13034=DIRECTION ( 'NONE',  ( 0.8571673013836867971, 1.049727191973306626E-16, -0.5150380737757237481 ) ) ;
#13040=CARTESIAN_POINT ( 'NONE',  ( 25.51458778375578973, 19.99999999999999289, 21.98440010584615578 ) ) ;
#13043=CARTESIAN_POINT ( 'NONE',  ( 22.23358001889399205, 29.90326853444953059, 11.84310668804517697 ) ) ;
#13046=CARTESIAN_POINT ( 'NONE',  ( 49.99999999999998579, 167.6227766016838530, 3.071800142134975431 ) ) ;
#13051=CIRCLE ( 'NONE', #2305, 2.500000000000002220 ) ;
#13052=ADVANCED_FACE ( 'NONE', ( #16815, #6014 ), #3449, .F. ) ;
#13055=ORIENTED_EDGE ( 'NONE', *, *, #14370, .F. ) ;
#13064=CARTESIAN_POINT ( 'NONE',  ( -12.54777316999452275, 31.64944667534048861, 11.54374194473465920 ) ) ;
#13065=CARTESIAN_POINT ( 'NONE',  ( -18.25212770525996930, 32.30769230769229949, 5.349717987761776428 ) ) ;
#13068=CARTESIAN_POINT ( 'NONE',  ( -68.00000000000000000, 171.6227766016838245, 0.000000000000000000 ) ) ;
#13070=DIRECTION ( 'NONE',  ( -1.000000000000000000, 0.000000000000000000, 0.000000000000000000 ) ) ;
#13071=DIRECTION ( 'NONE',  ( 0.000000000000000000, -1.000000000000000000, 0.000000000000000000 ) ) ;
#13074=CYLINDRICAL_SURFACE ( 'NONE', #12172, 2.499999999999998668 ) ;
#13078=CARTESIAN_POINT ( 'NONE',  ( 28.25663979599552178, 201.3127097690254175, 14.40604465277983159 ) ) ;
#13079=ORIENTED_EDGE ( 'NONE', *, *, #16165, .F. ) ;
#13083=CARTESIAN_POINT ( 'NONE',  ( -78.86956020503002662, 141.7478424248370175, 14.01801864773821649 ) ) ;
#13086=EDGE_CURVE ( 'NONE', #11927, #17386, #3362, .T. ) ;
#13090=DIRECTION ( 'NONE',  ( 1.000000000000000000, 0.000000000000000000, 0.000000000000000000 ) ) ;
#13093=ORIENTED_EDGE ( 'NONE', *, *, #1103, .T. ) ;
#13096=DIRECTION ( 'NONE',  ( 1.000000000000000000, 0.000000000000000000, 0.000000000000000000 ) ) ;
#13101=DIRECTION ( 'NONE',  ( 1.000000000000000000, 0.000000000000000000, 0.000000000000000000 ) ) ;
#13103=EDGE_CURVE ( 'NONE', #12728, #6874, #3597, .T. ) ;
#13106=CARTESIAN_POINT ( 'NONE',  ( -17.59086657693884703, 18.00000000000000000, 22.42595686383721443 ) ) ;
#13107=FACE_OUTER_BOUND ( 'NONE', #10018, .T. ) ;
#13108=CARTESIAN_POINT ( 'NONE',  ( 37.99999999999999289, 18.00000000000000355, 0.000000000000000000 ) ) ;
#13110=LINE ( 'NONE', #2053, #6175 ) ;
#13111=ADVANCED_FACE ( 'NONE', ( #703 ), #15310, .F. ) ;
#13115=EDGE_CURVE ( 'NONE', #13379, #16488, #4518, .T. ) ;
#13118=CARTESIAN_POINT ( 'NONE',  ( -10.04118010627649049, 19.99999999999999645, 24.87462214923097648 ) ) ;
#13119=CARTESIAN_POINT ( 'NONE',  ( 14.09268385650717015, 127.7503171827756034, 9.071975374176082241 ) ) ;
#13120=CARTESIAN_POINT ( 'NONE',  ( 29.53214135918837968, 19.99999999999999645, 18.68621337608103516 ) ) ;
#13123=ORIENTED_EDGE ( 'NONE', *, *, #3658, .T. ) ;
#13124=VECTOR ( 'NONE', #15600, 1000.000000000000114 ) ;
#13126=DIRECTION ( 'NONE',  ( 0.000000000000000000, 0.000000000000000000, -1.000000000000000000 ) ) ;
#13131=ORIENTED_EDGE ( 'NONE', *, *, #4526, .T. ) ;
#13133=DIRECTION ( 'NONE',  ( 0.000000000000000000, 0.000000000000000000, 1.000000000000000000 ) ) ;
#13134=ORIENTED_EDGE ( 'NONE', *, *, #11965, .F. ) ;
#13137=ORIENTED_EDGE ( 'NONE', *, *, #4965, .T. ) ;
#13139=VERTEX_POINT ( 'NONE', #16903 ) ;
#13141=EDGE_CURVE ( 'NONE', #15746, #7447, #16614, .T. ) ;
#13143=CARTESIAN_POINT ( 'NONE',  ( 48.00000000000000711, 159.6227766016838814, 5.571800142134975431 ) ) ;
#13146=CARTESIAN_POINT ( 'NONE',  ( 22.87887136921732889, 17.99999999999999645, 6.850254086360624939 ) ) ;
#13154=CARTESIAN_POINT ( 'NONE',  ( 24.93507336697352628, 29.86842105263157876, 4.999999999999999112 ) ) ;
#13156=DIRECTION ( 'NONE',  ( 0.000000000000000000, 0.000000000000000000, -1.000000000000000000 ) ) ;
#13162=VECTOR ( 'NONE', #6692, 1000.000000000000000 ) ;
#13163=DIRECTION ( 'NONE',  ( -1.000000000000000000, -0.000000000000000000, -0.000000000000000000 ) ) ;
#13168=CARTESIAN_POINT ( 'NONE',  ( -82.23503736807776932, 142.1468147500167447, 14.83914868552980515 ) ) ;
#13172=FACE_OUTER_BOUND ( 'NONE', #11459, .T. ) ;
#13175=DIRECTION ( 'NONE',  ( 1.000000000000000000, 0.000000000000000000, 0.000000000000000000 ) ) ;
#13176=CARTESIAN_POINT ( 'NONE',  ( 7.655193733048226257, 144.1839557653416080, 18.33333333333333925 ) ) ;
#13179=ORIENTED_EDGE ( 'NONE', *, *, #11201, .T. ) ;
#13180=ORIENTED_EDGE ( 'NONE', *, *, #2566, .F. ) ;
#13181=DIRECTION ( 'NONE',  ( 0.000000000000000000, 0.000000000000000000, -1.000000000000000000 ) ) ;
#13183=CARTESIAN_POINT ( 'NONE',  ( -95.00000000000000000, 201.6227766016838245, 0.000000000000000000 ) ) ;
#13186=ORIENTED_EDGE ( 'NONE', *, *, #6173, .T. ) ;
#13192=CARTESIAN_POINT ( 'NONE',  ( 196.0000000000000000, 167.6227766016838814, 16.92820660268601429 ) ) ;
#13197=CYLINDRICAL_SURFACE ( 'NONE', #3242, 2.499999999999998668 ) ;
#13208=EDGE_CURVE ( 'NONE', #17091, #978, #14063, .T. ) ;
#13209=CARTESIAN_POINT ( 'NONE',  ( -8.766611209709614272, 19.99999999999771916, 14.60748648876205458 ) ) ;
#13210=CARTESIAN_POINT ( 'NONE',  ( 14.60960092688903700, 138.5353766997065179, 5.001077596137333714 ) ) ;
#13215=DIRECTION ( 'NONE',  ( 0.000000000000000000, 0.000000000000000000, 1.000000000000000000 ) ) ;
#13216=EDGE_CURVE ( 'NONE', #11533, #14594, #17154, .T. ) ;
#13218=DIRECTION ( 'NONE',  ( 0.000000000000000000, 0.000000000000000000, -1.000000000000000000 ) ) ;
#13221=ORIENTED_EDGE ( 'NONE', *, *, #5015, .T. ) ;
#13225=FACE_OUTER_BOUND ( 'NONE', #16333, .T. ) ;
#13230=ADVANCED_FACE ( 'NONE', ( #7760 ), #3709, .F. ) ;
#13236=CARTESIAN_POINT ( 'NONE',  ( 27.99999999999998224, 9.999999999999998224, 0.000000000000000000 ) ) ;
#13237=EDGE_CURVE ( 'NONE', #16986, #15051, #3526, .T. ) ;
#13239=EDGE_CURVE ( 'NONE', #9957, #16088, #5301, .T. ) ;
#13241=CARTESIAN_POINT ( 'NONE',  ( 21.03896850327926060, 17.99999999999885247, 10.35865908471247643 ) ) ;
#13244=VECTOR ( 'NONE', #13943, 1000.000000000000000 ) ;
#13248=DIRECTION ( 'NONE',  ( 0.000000000000000000, 1.000000000000000000, 0.000000000000000000 ) ) ;
#13249=DIRECTION ( 'NONE',  ( 0.000000000000000000, 0.000000000000000000, -1.000000000000000000 ) ) ;
#13251=B_SPLINE_CURVE_WITH_KNOTS ( 'NONE', 3,
 ( #10422, #12117, #17155, #2466, #10696, #12018, #13176, #9095 ),
 .UNSPECIFIED., .F., .F.,
 ( 4, 2, 2, 4 ),
 ( 0.01981773175714084123, 0.02208185334846130693, 0.02434597493978176916, 0.02887421812242269709 ),
 .UNSPECIFIED. ) ;
#13253=CARTESIAN_POINT ( 'NONE',  ( -151.9615242270660929, 171.6227766016838245, 0.000000000000000000 ) ) ;
#13255=CARTESIAN_POINT ( 'NONE',  ( 31.12398805554424541, 201.4991975277559106, 14.01484360552157327 ) ) ;
#13261=CARTESIAN_POINT ( 'NONE',  ( -84.46916791769895383, 144.3624319200459070, 18.60312384224724980 ) ) ;
#13264=CARTESIAN_POINT ( 'NONE',  ( -27.29618490519992591, 19.99999999999999645, 10.29570512375934399 ) ) ;
#13269=CONICAL_SURFACE ( 'NONE', #14124, 2.500000000000002220, 1.029744260000002631 ) ;
#13274=EDGE_CURVE ( 'NONE', #12800, #14446, #2189, .T. ) ;
#13275=VERTEX_POINT ( 'NONE', #15916 ) ;
#13276=ORIENTED_EDGE ( 'NONE', *, *, #3391, .F. ) ;
#13278=ORIENTED_EDGE ( 'NONE', *, *, #10636, .T. ) ;
#13283=DIRECTION ( 'NONE',  ( 0.000000000000000000, 0.000000000000000000, 1.000000000000000000 ) ) ;
#13287=DIRECTION ( 'NONE',  ( 0.000000000000000000, 1.000000000000000000, 0.000000000000000000 ) ) ;
#13288=DIRECTION ( 'NONE',  ( 0.000000000000000000, 0.000000000000000000, 1.000000000000000000 ) ) ;
#13292=DIRECTION ( 'NONE',  ( 1.000000000000000000, 0.000000000000000000, 0.000000000000000000 ) ) ;
#13299=FACE_OUTER_BOUND ( 'NONE', #2156, .T. ) ;
#13303=ORIENTED_EDGE ( 'NONE', *, *, #10198, .T. ) ;
#13304=CARTESIAN_POINT ( 'NONE',  ( 27.50000000000001066, 146.6227766016838245, 0.000000000000000000 ) ) ;
#13305=CARTESIAN_POINT ( 'NONE',  ( 13.82444641086477866, 138.9325364249946517, 8.217559156358525740 ) ) ;
#13309=ORIENTED_EDGE ( 'NONE', *, *, #9681, .T. ) ;
#13313=FACE_OUTER_BOUND ( 'NONE', #11173, .T. ) ;
#13316=VERTEX_POINT ( 'NONE', #6541 ) ;
#13317=DIRECTION ( 'NONE',  ( -6.938893903907228378E-16, 1.000000000000000000, 0.000000000000000000 ) ) ;
#13320=FACE_OUTER_BOUND ( 'NONE', #6608, .T. ) ;
#13321=AXIS2_PLACEMENT_3D ( 'NONE', #8093, #3957, #52 ) ;
#13333=CARTESIAN_POINT ( 'NONE',  ( -82.87337507697658623, 150.7186413122655892, 25.53493815998142935 ) ) ;
#13335=VERTEX_POINT ( 'NONE', #15649 ) ;
#13346=CARTESIAN_POINT ( 'NONE',  ( 25.98211652881812483, 199.6128501304145004, 17.48539201980446123 ) ) ;
#13351=CARTESIAN_POINT ( 'NONE',  ( -75.00000000000002842, 146.3163998792643952, 21.18507967179267482 ) ) ;
#13352=CARTESIAN_POINT ( 'NONE',  ( -16.30611068361787019, 32.76923076923078781, 4.999999999999999112 ) ) ;
#13354=CARTESIAN_POINT ( 'NONE',  ( -24.80114670877660643, 19.99999999999999289, 15.70637264050929538 ) ) ;
#13355=ORIENTED_EDGE ( 'NONE', *, *, #10851, .T. ) ;
#13374=CARTESIAN_POINT ( 'NONE',  ( -27.98221281347032274, 18.00000000000000000, 4.999999999999996447 ) ) ;
#13377=EDGE_LOOP ( 'NONE', ( #2245, #7462, #14220, #9570 ) ) ;
#13378=CARTESIAN_POINT ( 'NONE',  ( -68.00000000000000000, 154.3022685259950038, 9.999999999999900524 ) ) ;
#13379=VERTEX_POINT ( 'NONE', #16274 ) ;
#13383=CARTESIAN_POINT ( 'NONE',  ( -12.63609539511577218, 19.99999999999999645, 24.35132453916816431 ) ) ;
#13384=CARTESIAN_POINT ( 'NONE',  ( 13.63270490666636192, 138.8028880870465969, 3.449993069226350517 ) ) ;
#13385=ORIENTED_EDGE ( 'NONE', *, *, #9747, .F. ) ;
#13387=EDGE_LOOP ( 'NONE', ( #11785, #1860 ) ) ;
#13389=EDGE_CURVE ( 'NONE', #9250, #12210, #15023, .T. ) ;
#13391=EDGE_CURVE ( 'NONE', #2395, #2095, #7560, .T. ) ;
#13394=EDGE_CURVE ( 'NONE', #11331, #11495, #4465, .T. ) ;
#13398=CARTESIAN_POINT ( 'NONE',  ( 27.12662492302345996, 150.7186413122655892, 25.53493815998142225 ) ) ;
#13402=ORIENTED_EDGE ( 'NONE', *, *, #15800, .T. ) ;
#13406=ADVANCED_FACE ( 'NONE', ( #9365 ), #17521, .F. ) ;
#13407=DIRECTION ( 'NONE',  ( 0.000000000000000000, -1.000000000000000000, 6.123233995736762338E-17 ) ) ;
#13411=CARTESIAN_POINT ( 'NONE',  ( -18.09555036921010540, 32.27673591576833445, 6.733025906873759681 ) ) ;
#13414=CARTESIAN_POINT ( 'NONE',  ( -77.13041205501343711, 150.7324203247391381, 25.54751979981075394 ) ) ;
#13418=CARTESIAN_POINT ( 'NONE',  ( -50.00000000000000000, 171.6227766016838245, 0.000000000000000000 ) ) ;
#13420=DIRECTION ( 'NONE',  ( -1.000000000000000000, -0.000000000000000000, -0.000000000000000000 ) ) ;
#13421=DIRECTION ( 'NONE',  ( -1.000000000000000000, -0.000000000000000000, -0.000000000000000000 ) ) ;
#13422=DIRECTION ( 'NONE',  ( 1.000000000000000000, 0.000000000000000000, 0.000000000000000000 ) ) ;
#13424=CARTESIAN_POINT ( 'NONE',  ( -45.00000000000000000, 134.2062027339443944, 15.00000000000000000 ) ) ;
#13427=ADVANCED_FACE ( 'NONE', ( #1404 ), #2815, .F. ) ;
#13428=ORIENTED_EDGE ( 'NONE', *, *, #15077, .F. ) ;
#13431=AXIS2_PLACEMENT_3D ( 'NONE', #30, #2771, #8162 ) ;
#13433=CARTESIAN_POINT ( 'NONE',  ( -77.77610210663782198, 142.1412512070565413, 14.82809033015227307 ) ) ;
#13435=LINE ( 'NONE', #5117, #8337 ) ;
#13437=CARTESIAN_POINT ( 'NONE',  ( -27.98221281347037959, 20.00000000000000355, 5.670874406215274277 ) ) ;
#13439=VERTEX_POINT ( 'NONE', #15103 ) ;
#13446=ORIENTED_EDGE ( 'NONE', *, *, #12472, .T. ) ;
#13453=FACE_OUTER_BOUND ( 'NONE', #294, .T. ) ;
#13456=VECTOR ( 'NONE', #7150, 1000.000000000000000 ) ;
#13457=CARTESIAN_POINT ( 'NONE',  ( -24.94987437106622252, 100.0000000000000142, 6.000000000000000000 ) ) ;
#13463=CARTESIAN_POINT ( 'NONE',  ( 27.50000000000000355, 196.6227766016838245, 0.000000000000000000 ) ) ;
#13464=DIRECTION ( 'NONE',  ( 0.000000000000000000, 0.000000000000000000, 1.000000000000000000 ) ) ;
#13465=CYLINDRICAL_SURFACE ( 'NONE', #11709, 20.00000000000000355 ) ;
#13468=ORIENTED_EDGE ( 'NONE', *, *, #16262, .T. ) ;
#13473=AXIS2_PLACEMENT_3D ( 'NONE', #10218, #12796, #7642 ) ;
#13475=CARTESIAN_POINT ( 'NONE',  ( -17.59086657693882927, 19.99999999999999645, 22.42595686383492293 ) ) ;
#13476=CARTESIAN_POINT ( 'NONE',  ( 12.08578903453337183, 130.1663611114758510, 11.02150463548631976 ) ) ;
#13477=VERTEX_POINT ( 'NONE', #7063 ) ;
#13478=CARTESIAN_POINT ( 'NONE',  ( 19.14963388379468157, 19.99999999999999645, 24.55317681541820463 ) ) ;
#13481=AXIS2_PLACEMENT_3D ( 'NONE', #7005, #2924, #15130 ) ;
#13482=VECTOR ( 'NONE', #4022, 1000.000000000000114 ) ;
#13484=CARTESIAN_POINT ( 'NONE',  ( 49.99999999999998579, 151.6227766016839098, 3.071800142134974099 ) ) ;
#13485=AXIS2_PLACEMENT_3D ( 'NONE', #10025, #13868, #15437 ) ;
#13486=CARTESIAN_POINT ( 'NONE',  ( 27.47046400057530846, 138.6909045376442009, 2.448381753924629756 ) ) ;
#13489=VERTEX_POINT ( 'NONE', #244 ) ;
#13493=CARTESIAN_POINT ( 'NONE',  ( -43.00000000000000000, 130.0000000000000000, 0.000000000000000000 ) ) ;
#13495=EDGE_LOOP ( 'NONE', ( #12518, #12247, #5114, #3701, #16828, #14046, #13093, #6059, #6568, #1549, #16983, #16434, #14470, #10561, #14595 ) ) ;
#13502=CARTESIAN_POINT ( 'NONE',  ( 10.67016715011939176, 138.9541284244158419, 13.78020913810612491 ) ) ;
#13506=DIRECTION ( 'NONE',  ( -1.000000000000000000, -0.000000000000000000, -0.000000000000000000 ) ) ;
#13507=DIRECTION ( 'NONE',  ( 0.000000000000000000, -0.000000000000000000, -1.000000000000000000 ) ) ;
#13510=DIRECTION ( 'NONE',  ( 1.000000000000000000, 0.000000000000000000, 0.000000000000000000 ) ) ;
#13515=LINE ( 'NONE', #8011, #12462 ) ;
#13519=AXIS2_PLACEMENT_3D ( 'NONE', #14698, #3999, #1325 ) ;
#13526=CONICAL_SURFACE ( 'NONE', #6453, 2.499999999999998668, 1.029744260000002187 ) ;
#13527=CARTESIAN_POINT ( 'NONE',  ( -95.00000000000000000, 171.6227766016838245, 0.000000000000000000 ) ) ;
#13529=FACE_OUTER_BOUND ( 'NONE', #8203, .T. ) ;
#13530=VERTEX_POINT ( 'NONE', #12635 ) ;
#13536=VECTOR ( 'NONE', #5583, 1000.000000000000114 ) ;
#13539=EDGE_LOOP ( 'NONE', ( #7309, #13813, #2006, #8815 ) ) ;
#13540=FACE_OUTER_BOUND ( 'NONE', #11672, .T. ) ;
#13548=CIRCLE ( 'NONE', #12976, 2.500000000000002220 ) ;
#13549=CARTESIAN_POINT ( 'NONE',  ( 34.24368835419660684, 193.9611582889533281, 24.29263104154015096 ) ) ;
#13551=CARTESIAN_POINT ( 'NONE',  ( 27.99999999999998224, 9.999999999999998224, 11.50215154306610188 ) ) ;
#13554=CARTESIAN_POINT ( 'NONE',  ( -12.80328004466210601, 17.99999999999999645, 4.999999999999999112 ) ) ;
#13555=CARTESIAN_POINT ( 'NONE',  ( 50.00000000000000000, 196.6227766016838245, 0.000000000000000000 ) ) ;
#13556=EDGE_CURVE ( 'NONE', #13489, #11737, #16349, .T. ) ;
#13561=DIRECTION ( 'NONE',  ( 0.000000000000000000, 0.000000000000000000, -1.000000000000000000 ) ) ;
#13564=EDGE_CURVE ( 'NONE', #11802, #10896, #15636, .T. ) ;
#13566=ORIENTED_EDGE ( 'NONE', *, *, #6786, .T. ) ;
#13567=EDGE_CURVE ( 'NONE', #13780, #16273, #15554, .T. ) ;
#13568=CARTESIAN_POINT ( 'NONE',  ( -18.25212770525992667, 32.30769230769230660, 4.999999999999998224 ) ) ;
#13578=AXIS2_PLACEMENT_3D ( 'NONE', #4940, #1141, #14425 ) ;
#13580=CARTESIAN_POINT ( 'NONE',  ( 27.48361012698968864, 138.6227766016838245, 1.063447695028166570E-14 ) ) ;
#13581=AXIS2_PLACEMENT_3D ( 'NONE', #2302, #13101, #6732 ) ;
#13583=CARTESIAN_POINT ( 'NONE',  ( 35.00000000000001421, 146.8780590376976249, 21.83693896782702382 ) ) ;
#13584=VERTEX_POINT ( 'NONE', #15715 ) ;
#13587=CARTESIAN_POINT ( 'NONE',  ( -100.0000000000000000, 100.0000000000000142, 6.000000000000000000 ) ) ;
#13591=VECTOR ( 'NONE', #15202, 1000.000000000000000 ) ;
#13592=CARTESIAN_POINT ( 'NONE',  ( 11.28101412774664958, 138.8108036852440250, 13.45198100927934348 ) ) ;
#13596=CARTESIAN_POINT ( 'NONE',  ( 48.00000000000000711, 167.6227766016838530, 5.571800142134975431 ) ) ;
#13599=EDGE_CURVE ( 'NONE', #9285, #9957, #15417, .T. ) ;
#13601=ADVANCED_FACE ( 'NONE', ( #3767 ), #4917, .F. ) ;
#13602=CARTESIAN_POINT ( 'NONE',  ( -76.58334154245484626, 150.2902214191207975, 25.17945278758670824 ) ) ;
#13603=ADVANCED_FACE ( 'NONE', ( #14567 ), #9158, .F. ) ;
#13605=DIRECTION ( 'NONE',  ( 0.000000000000000000, 0.000000000000000000, 1.000000000000000000 ) ) ;
#13606=AXIS2_PLACEMENT_3D ( 'NONE', #13839, #9997, #9741 ) ;
#13608=DIRECTION ( 'NONE',  ( -1.000000000000000000, -0.000000000000000000, -0.000000000000000000 ) ) ;
#13615=AXIS2_PLACEMENT_3D ( 'NONE', #10284, #8963, #14374 ) ;
#13627=CARTESIAN_POINT ( 'NONE',  ( 14.93242934743711992, 30.00000000000000000, 25.00000000000000000 ) ) ;
#13632=DIRECTION ( 'NONE',  ( -0.000000000000000000, -0.000000000000000000, -1.000000000000000000 ) ) ;
#13637=CARTESIAN_POINT ( 'NONE',  ( 31.55028006451160394, 191.8535701216948155, 26.07159546787933024 ) ) ;
#13640=CARTESIAN_POINT ( 'NONE',  ( 17.01457324639674695, 29.95810005730942649, 12.72891809691981102 ) ) ;
#13647=ORIENTED_EDGE ( 'NONE', *, *, #10200, .T. ) ;
#13648=CARTESIAN_POINT ( 'NONE',  ( -3.000000000000000888, 154.3022685259950038, 9.999999999999900524 ) ) ;
#13650=ORIENTED_EDGE ( 'NONE', *, *, #9927, .F. ) ;
#13651=PRODUCT_DEFINITION_SHAPE ( 'NONE', 'NONE',  #3279 ) ;
#13660=ADVANCED_FACE ( 'NONE', ( #17221 ), #13807, .F. ) ;
#13662=ORIENTED_EDGE ( 'NONE', *, *, #9391, .T. ) ;
#13663=CARTESIAN_POINT ( 'NONE',  ( 35.00000000000000711, 146.6227766016838245, 21.54065922853802562 ) ) ;
#13666=LINE ( 'NONE', #4107, #5062 ) ;
#13667=DIRECTION ( 'NONE',  ( 8.673617379884037937E-17, 0.000000000000000000, -1.000000000000000000 ) ) ;
#13670=VERTEX_POINT ( 'NONE', #15631 ) ;
#13675=LINE ( 'NONE', #5363, #3134 ) ;
#13677=FACE_OUTER_BOUND ( 'NONE', #6821, .T. ) ;
#13679=CARTESIAN_POINT ( 'NONE',  ( -75.93727504753279334, 149.5415222133261182, 24.52446659945425367 ) ) ;
#13682=DIRECTION ( 'NONE',  ( 1.000000000000000000, 6.217248937900877415E-15, 0.000000000000000000 ) ) ;
#13683=DIRECTION ( 'NONE',  ( -1.000000000000000000, -0.000000000000000000, -0.000000000000000000 ) ) ;
#13684=AXIS2_PLACEMENT_3D ( 'NONE', #13873, #13683, #15274 ) ;
#13688=EDGE_LOOP ( 'NONE', ( #17302, #2203, #4171, #104, #9398 ) ) ;
#13691=EDGE_LOOP ( 'NONE', ( #10241, #4311, #3453, #1884 ) ) ;
#13692=ORIENTED_EDGE ( 'NONE', *, *, #13208, .T. ) ;
#13693=CARTESIAN_POINT ( 'NONE',  ( -15.00000000000001421, 19.99999999999995737, 13.00000000000000000 ) ) ;
#13695=AXIS2_PLACEMENT_3D ( 'NONE', #8538, #3487, #7460 ) ;
#13701=DIRECTION ( 'NONE',  ( 0.000000000000000000, 0.000000000000000000, -1.000000000000000000 ) ) ;
#13702=CARTESIAN_POINT ( 'NONE',  ( 48.00000000000000711, 191.6227766016837677, 5.571800142134975431 ) ) ;
#13705=EDGE_CURVE ( 'NONE', #14253, #5417, #11813, .T. ) ;
#13706=EDGE_CURVE ( 'NONE', #10977, #3421, #12952, .T. ) ;
#13707=AXIS2_PLACEMENT_3D ( 'NONE', #11909, #13071, #17315 ) ;
#13708=ADVANCED_FACE ( 'NONE', ( #3960, #4217 ), #16083, .F. ) ;
#13709=VERTEX_POINT ( 'NONE', #1289 ) ;
#13715=CARTESIAN_POINT ( 'NONE',  ( 29.02955226949582368, 191.7140209832038238, 26.17909706909631851 ) ) ;
#13717=PLANE ( 'NONE',  #7259 ) ;
#13731=CARTESIAN_POINT ( 'NONE',  ( -15.33310217279680288, 19.99999999999999645, 4.999999999999999112 ) ) ;
#13735=AXIS2_PLACEMENT_3D ( 'NONE', #6524, #9168, #9080 ) ;
#13740=CARTESIAN_POINT ( 'NONE',  ( -23.00000000000000000, 120.0000000000000284, 4.999999999999999112 ) ) ;
#13744=AXIS2_PLACEMENT_3D ( 'NONE', #1886, #12947, #1974 ) ;
#13745=CARTESIAN_POINT ( 'NONE',  ( 25.00000000000000711, 146.6227766016838245, 21.54065922853802562 ) ) ;
#13746=CIRCLE ( 'NONE', #16003, 33.00000000000000000 ) ;
#13751=VERTEX_POINT ( 'NONE', #6949 ) ;
#13752=ADVANCED_FACE ( 'NONE', ( #4302 ), #135, .F. ) ;
#13756=VERTEX_POINT ( 'NONE', #12089 ) ;
#13757=ORIENTED_EDGE ( 'NONE', *, *, #3571, .F. ) ;
#13758=CARTESIAN_POINT ( 'NONE',  ( 48.00000000000000711, 151.6227766016839098, 5.571800142134973655 ) ) ;
#13759=CARTESIAN_POINT ( 'NONE',  ( 17.56954167074719919, 125.3114906870353167, 3.338394383324010395 ) ) ;
#13760=CARTESIAN_POINT ( 'NONE',  ( 18.30724418481576166, 140.7653321920888345, 16.52022657272140904 ) ) ;
#13762=AXIS2_PLACEMENT_3D ( 'NONE', #5421, #16223, #11145 ) ;
#13764=ORIENTED_EDGE ( 'NONE', *, *, #16931, .T. ) ;
#13766=DIRECTION ( 'NONE',  ( 0.000000000000000000, 1.000000000000000000, 0.000000000000000000 ) ) ;
#13772=CYLINDRICAL_SURFACE ( 'NONE', #13485, 2.500000000000000444 ) ;
#13773=ORIENTED_EDGE ( 'NONE', *, *, #3323, .F. ) ;
#13775=DIRECTION ( 'NONE',  ( -0.000000000000000000, -0.000000000000000000, 1.000000000000000000 ) ) ;
#13777=EDGE_CURVE ( 'NONE', #8027, #5427, #515, .T. ) ;
#13778=CARTESIAN_POINT ( 'NONE',  ( -40.00000000000000711, 0.000000000000000000, 0.000000000000000000 ) ) ;
#13780=VERTEX_POINT ( 'NONE', #3049 ) ;
#13793=DIRECTION ( 'NONE',  ( -1.000000000000000000, 0.000000000000000000, 0.000000000000000000 ) ) ;
#13799=AXIS2_PLACEMENT_3D ( 'NONE', #2080, #8816, #12802 ) ;
#13801=CARTESIAN_POINT ( 'NONE',  ( 49.99999999999998579, 175.6227766016838245, 5.571800142134975431 ) ) ;
#13807=CONICAL_SURFACE ( 'NONE', #6165, 2.500000000000002220, 1.029744260000002631 ) ;
#13810=AXIS2_PLACEMENT_3D ( 'NONE', #5045, #14607, #6733 ) ;
#13813=ORIENTED_EDGE ( 'NONE', *, *, #10094, .T. ) ;
#13815=CYLINDRICAL_SURFACE ( 'NONE', #1935, 5.000000000000004441 ) ;
#13818=CYLINDRICAL_SURFACE ( 'NONE', #3885, 2.499999999999998668 ) ;
#13819=CARTESIAN_POINT ( 'NONE',  ( -43.00000000000000711, 130.0000000000000000, 12.99999999999999822 ) ) ;
#13823=CARTESIAN_POINT ( 'NONE',  ( -82.96816024544703794, 200.6580771142793651, 15.68801935549125481 ) ) ;
#13824=EDGE_CURVE ( 'NONE', #4320, #805, #7572, .T. ) ;
#13829=LINE ( 'NONE', #8411, #14289 ) ;
#13830=FACE_OUTER_BOUND ( 'NONE', #4942, .T. ) ;
#13832=CARTESIAN_POINT ( 'NONE',  ( -17.11671918504270451, 32.08177433558115865, 9.477319364664337442 ) ) ;
#13834=AXIS2_PLACEMENT_3D ( 'NONE', #16131, #10532, #5490 ) ;
#13835=VERTEX_POINT ( 'NONE', #2962 ) ;
#13839=CARTESIAN_POINT ( 'NONE',  ( 27.99999999999998224, 9.999999999999998224, 35.00200000000000244 ) ) ;
#13843=EDGE_CURVE ( 'NONE', #15544, #2395, #10029, .T. ) ;
#13845=CARTESIAN_POINT ( 'NONE',  ( -70.00000000000000000, 206.6227766016838245, -2.143131898507868248E-15 ) ) ;
#13849=VECTOR ( 'NONE', #15597, 1000.000000000000000 ) ;
#13853=LINE ( 'NONE', #9757, #14029 ) ;
#13854=ORIENTED_EDGE ( 'NONE', *, *, #14670, .F. ) ;
#13858=CARTESIAN_POINT ( 'NONE',  ( 15.33542211484438056, 137.4551579351393400, 9.454295640946218882 ) ) ;
#13861=EDGE_LOOP ( 'NONE', ( #2098, #8647, #3488, #8675 ) ) ;
#13866=DIRECTION ( 'NONE',  ( 1.000000000000000000, -0.000000000000000000, 0.000000000000000000 ) ) ;
#13868=DIRECTION ( 'NONE',  ( -1.000000000000000000, -0.000000000000000000, -0.000000000000000000 ) ) ;
#13872=DIRECTION ( 'NONE',  ( -1.000000000000000000, 0.000000000000000000, 0.000000000000000000 ) ) ;
#13873=CARTESIAN_POINT ( 'NONE',  ( 196.0000000000000000, 175.6227766016838530, 19.42820660268601074 ) ) ;
#13877=AXIS2_PLACEMENT_3D ( 'NONE', #9801, #16542, #13895 ) ;
#13880=AXIS2_PLACEMENT_3D ( 'NONE', #14477, #17214, #5091 ) ;
#13881=CARTESIAN_POINT ( 'NONE',  ( 11.58137902169841027, 143.8440485058968363, 17.81491816053495825 ) ) ;
#13882=ORIENTED_EDGE ( 'NONE', *, *, #279, .T. ) ;
#13884=VERTEX_POINT ( 'NONE', #3226 ) ;
#13889=AXIS2_PLACEMENT_3D ( 'NONE', #1646, #13775, #2964 ) ;
#13893=CARTESIAN_POINT ( 'NONE',  ( 34.97205211421869819, 146.0169975363979802, 20.82225907110314012 ) ) ;
#13895=DIRECTION ( 'NONE',  ( 0.000000000000000000, 0.000000000000000000, 1.000000000000000000 ) ) ;
#13897=CARTESIAN_POINT ( 'NONE',  ( -40.00000000000000000, 0.000000000000000000, 33.00000000000000711 ) ) ;
#13898=ADVANCED_FACE ( 'NONE', ( #5716 ), #14645, .F. ) ;
#13899=VECTOR ( 'NONE', #2957, 1000.000000000000000 ) ;
#13901=ORIENTED_EDGE ( 'NONE', *, *, #2622, .F. ) ;
#13905=CARTESIAN_POINT ( 'NONE',  ( 27.99999999999998224, 9.999999999999998224, 35.00200000000000244 ) ) ;
#13910=CARTESIAN_POINT ( 'NONE',  ( -85.00000000000002842, 196.6227766016838245, 21.54065922853802562 ) ) ;
#13914=CARTESIAN_POINT ( 'NONE',  ( 48.00000000000000711, 163.6227766016838530, 12.50000337241049309 ) ) ;
#13917=CARTESIAN_POINT ( 'NONE',  ( -26.11264420168842904, 19.99999999999999645, 13.35921939055851482 ) ) ;
#13918=DIRECTION ( 'NONE',  ( 1.000000000000000000, 0.000000000000000000, 0.000000000000000000 ) ) ;
#13924=LINE ( 'NONE', #3201, #16266 ) ;
#13928=ORIENTED_EDGE ( 'NONE', *, *, #15837, .T. ) ;
#13931=LINE ( 'NONE', #3392, #1107 ) ;
#13934=EDGE_LOOP ( 'NONE', ( #16347, #963 ) ) ;
#13937=EDGE_CURVE ( 'NONE', #16675, #11660, #5323, .T. ) ;
#13940=CARTESIAN_POINT ( 'NONE',  ( 21.84350049701297536, 139.6359888969276426, 14.21326463380156646 ) ) ;
#13943=DIRECTION ( 'NONE',  ( 1.000000000000000000, 0.000000000000000000, 0.000000000000000000 ) ) ;
#13945=CARTESIAN_POINT ( 'NONE',  ( -85.00000000000002842, 196.6227766016838245, 21.54065922853802562 ) ) ;
#13947=CARTESIAN_POINT ( 'NONE',  ( 24.93034343272520204, 18.00000000000000000, 22.33460256651928333 ) ) ;
#13952=DIRECTION ( 'NONE',  ( -0.000000000000000000, -0.000000000000000000, -1.000000000000000000 ) ) ;
#13959=CARTESIAN_POINT ( 'NONE',  ( 6.134011831684059501, 140.6204725398426092, 12.99999999999999822 ) ) ;
#13960=ORIENTED_EDGE ( 'NONE', *, *, #520, .T. ) ;
#13964=DIRECTION ( 'NONE',  ( 0.000000000000000000, 0.000000000000000000, -1.000000000000000000 ) ) ;
#13965=DIRECTION ( 'NONE',  ( 1.000000000000000000, 0.000000000000000000, -0.000000000000000000 ) ) ;
#13969=CARTESIAN_POINT ( 'NONE',  ( 29.51948765637180827, 141.6406938050144220, 13.78697217532817376 ) ) ;
#13972=DIRECTION ( 'NONE',  ( 0.000000000000000000, 1.000000000000000000, 0.000000000000000000 ) ) ;
#13973=EDGE_CURVE ( 'NONE', #544, #5825, #7554, .T. ) ;
#13981=CARTESIAN_POINT ( 'NONE',  ( 7.376038361426209278, 142.5209969267753536, 19.44444444444444642 ) ) ;
#13982=CIRCLE ( 'NONE', #11692, 2.500000000000002220 ) ;
#13985=CARTESIAN_POINT ( 'NONE',  ( 30.00000000000000355, 196.6227766016838245, 0.000000000000000000 ) ) ;
#13986=CARTESIAN_POINT ( 'NONE',  ( 20.21973759693270267, 29.89473369120481294, 11.02800485953945930 ) ) ;
#13988=DIRECTION ( 'NONE',  ( -0.000000000000000000, -0.000000000000000000, -1.000000000000000000 ) ) ;
#13989=CARTESIAN_POINT ( 'NONE',  ( 22.93524650466161674, 29.84210526315774104, 5.528366322421692125 ) ) ;
#13990=CARTESIAN_POINT ( 'NONE',  ( -78.87601194445579722, 201.4991975277559675, 14.01484360552155373 ) ) ;
#13992=VECTOR ( 'NONE', #552, 1000.000000000000000 ) ;
#13993=ORIENTED_EDGE ( 'NONE', *, *, #11334, .T. ) ;
#13994=ORIENTED_EDGE ( 'NONE', *, *, #13239, .T. ) ;
#13995=DIRECTION ( 'NONE',  ( -1.000000000000000000, 0.000000000000000000, 0.000000000000000000 ) ) ;
#13997=ORIENTED_EDGE ( 'NONE', *, *, #6417, .T. ) ;
#14002=CARTESIAN_POINT ( 'NONE',  ( 14.93242934743710393, 30.00000000000000000, 13.00000000000000178 ) ) ;
#14013=EDGE_CURVE ( 'NONE', #6313, #10830, #9266, .T. ) ;
#14015=CARTESIAN_POINT ( 'NONE',  ( 27.48361012698969930, 136.6227766016838245, 1.296296296296295614 ) ) ;
#14016=AXIS2_PLACEMENT_3D ( 'NONE', #4318, #16270, #4407 ) ;
#14022=CIRCLE ( 'NONE', #3808, 25.00000000000000000 ) ;
#14023=CARTESIAN_POINT ( 'NONE',  ( 17.54349574104652021, 125.4948194589026684, 5.000000000000000888 ) ) ;
#14024=CARTESIAN_POINT ( 'NONE',  ( 23.14977753070778377, 139.1449216839932319, 13.05325656350955654 ) ) ;
#14029=VECTOR ( 'NONE', #461, 1000.000000000000000 ) ;
#14031=CARTESIAN_POINT ( 'NONE',  ( -75.92991404580537562, 193.7005638513908252, 24.52922227238014230 ) ) ;
#14032=DIRECTION ( 'NONE',  ( 1.000000000000000000, 0.000000000000000000, 0.000000000000000000 ) ) ;
#14036=ORIENTED_EDGE ( 'NONE', *, *, #5474, .T. ) ;
#14041=DIRECTION ( 'NONE',  ( 8.673617379884037937E-17, 0.000000000000000000, -1.000000000000000000 ) ) ;
#14046=ORIENTED_EDGE ( 'NONE', *, *, #15675, .T. ) ;
#14047=ORIENTED_EDGE ( 'NONE', *, *, #5815, .T. ) ;
#14048=ORIENTED_EDGE ( 'NONE', *, *, #14670, .T. ) ;
#14050=CARTESIAN_POINT ( 'NONE',  ( 9.466951579747838963, 140.2095812714875080, 12.14773935231147739 ) ) ;
#14059=AXIS2_PLACEMENT_3D ( 'NONE', #2832, #12040, #8229 ) ;
#14061=CARTESIAN_POINT ( 'NONE',  ( 28.85491924750536796, 141.7513145237122387, 14.02541974480121034 ) ) ;
#14062=DIRECTION ( 'NONE',  ( 1.000000000000000000, -0.000000000000000000, -0.000000000000000000 ) ) ;
#14063=CIRCLE ( 'NONE', #6409, 9.999999999999998224 ) ;
#14064=CARTESIAN_POINT ( 'NONE',  ( 196.0000000000000000, 167.6227766016838814, 21.92820660268601074 ) ) ;
#14066=DIRECTION ( 'NONE',  ( 0.000000000000000000, 0.000000000000000000, -1.000000000000000000 ) ) ;
#14067=PLANE ( 'NONE',  #5534 ) ;
#14073=CARTESIAN_POINT ( 'NONE',  ( 17.37251483187831624, 141.0177972567464906, 16.98271123612915545 ) ) ;
#14075=ORIENTED_EDGE ( 'NONE', *, *, #9328, .F. ) ;
#14080=ORIENTED_EDGE ( 'NONE', *, *, #10468, .F. ) ;
#14083=CARTESIAN_POINT ( 'NONE',  ( -77.93947261911883118, 201.1823876344234350, 14.67159435888866525 ) ) ;
#14086=VERTEX_POINT ( 'NONE', #920 ) ;
#14088=VECTOR ( 'NONE', #4657, 1000.000000000000000 ) ;
#14096=CARTESIAN_POINT ( 'NONE',  ( -19.25702671965663626, 18.00000000000000355, 21.36300512502526061 ) ) ;
#14100=DIRECTION ( 'NONE',  ( 0.000000000000000000, -0.8660254037844413721, 0.4999999999999953371 ) ) ;
#14106=EDGE_CURVE ( 'NONE', #15544, #8340, #11250, .T. ) ;
#14110=EDGE_CURVE ( 'NONE', #10896, #11802, #10520, .T. ) ;
#14112=ORIENTED_EDGE ( 'NONE', *, *, #5206, .T. ) ;
#14113=CYLINDRICAL_SURFACE ( 'NONE', #11427, 8.000000000000000000 ) ;
#14114=CIRCLE ( 'NONE', #241, 20.00000000000000355 ) ;
#14115=CARTESIAN_POINT ( 'NONE',  ( 24.87018239537452757, 29.86925179676151032, 6.310755877675157777 ) ) ;
#14116=CARTESIAN_POINT ( 'NONE',  ( 26.85584576128377066, 137.3904121345421458, 7.294850950184896377 ) ) ;
#14118=DIRECTION ( 'NONE',  ( -0.000000000000000000, -0.000000000000000000, -1.000000000000000000 ) ) ;
#14119=FACE_OUTER_BOUND ( 'NONE', #6404, .T. ) ;
#14120=CARTESIAN_POINT ( 'NONE',  ( -79.20543317789827142, 191.6823464236538825, 26.20333082749371556 ) ) ;
#14122=LINE ( 'NONE', #5881, #16159 ) ;
#14123=CARTESIAN_POINT ( 'NONE',  ( 14.93242934743710570, 18.00000000000000000, 25.00000000000000000 ) ) ;
#14124=AXIS2_PLACEMENT_3D ( 'NONE', #2943, #9580, #2862 ) ;
#14132=CARTESIAN_POINT ( 'NONE',  ( -24.99999999999999289, 90.00000000000000000, 0.000000000000000000 ) ) ;
#14134=ORIENTED_EDGE ( 'NONE', *, *, #6721, .F. ) ;
#14135=ORIENTED_EDGE ( 'NONE', *, *, #13389, .F. ) ;
#14139=CIRCLE ( 'NONE', #1124, 5.000000000000004441 ) ;
#14142=ADVANCED_FACE ( 'NONE', ( #7908 ), #10824, .F. ) ;
#14145=DIRECTION ( 'NONE',  ( -1.000000000000000000, 8.673617379884038430E-16, 0.000000000000000000 ) ) ;
#14147=ORIENTED_EDGE ( 'NONE', *, *, #2937, .T. ) ;
#14148=DIRECTION ( 'NONE',  ( 0.000000000000000000, 0.000000000000000000, -1.000000000000000000 ) ) ;
#14155=FACE_OUTER_BOUND ( 'NONE', #716, .T. ) ;
#14156=LINE ( 'NONE', #11397, #3676 ) ;
#14157=VERTEX_POINT ( 'NONE', #14897 ) ;
#14158=CARTESIAN_POINT ( 'NONE',  ( 37.99999999999998579, 2.000000000000000000, 28.00000000000001066 ) ) ;
#14161=ADVANCED_FACE ( 'NONE', ( #202 ), #15960, .F. ) ;
#14171=DIRECTION ( 'NONE',  ( 1.000000000000000000, 0.000000000000000000, 0.000000000000000000 ) ) ;
#14172=CARTESIAN_POINT ( 'NONE',  ( -85.00000000000001421, 197.2415780845126676, 20.82248078717324091 ) ) ;
#14180=EDGE_CURVE ( 'NONE', #11846, #9474, #3067, .T. ) ;
#14182=DIRECTION ( 'NONE',  ( 0.000000000000000000, 1.000000000000000000, 0.000000000000000000 ) ) ;
#14183=ORIENTED_EDGE ( 'NONE', *, *, #700, .F. ) ;
#14185=CIRCLE ( 'NONE', #14748, 33.00000000000000000 ) ;
#14187=PLANE ( 'NONE',  #15120 ) ;
#14188=CARTESIAN_POINT ( 'NONE',  ( -14.55266450408069723, 18.00000000000000000, 23.76398220081675206 ) ) ;
#14192=CARTESIAN_POINT ( 'NONE',  ( -77.50000000000002842, 146.6227766016838245, 0.000000000000000000 ) ) ;
#14198=DIRECTION ( 'NONE',  ( -0.000000000000000000, -0.000000000000000000, -1.000000000000000000 ) ) ;
#14199=CARTESIAN_POINT ( 'NONE',  ( 24.93507336697353338, 29.86842105263157521, 5.000000000000004441 ) ) ;
#14200=CARTESIAN_POINT ( 'NONE',  ( 13.66217116581496249, 130.1207327347060527, 12.31521373833130717 ) ) ;
#14201=EDGE_LOOP ( 'NONE', ( #10038, #2153, #4410, #9811 ) ) ;
#14202=ADVANCED_FACE ( 'NONE', ( #3124, #2941, #12682 ), #9932, .F. ) ;
#14204=EDGE_CURVE ( 'NONE', #15970, #14594, #11162, .T. ) ;
#14205=CARTESIAN_POINT ( 'NONE',  ( -82.56615862916986259, 192.3153571870206804, 25.70724251753716061 ) ) ;
#14206=CARTESIAN_POINT ( 'NONE',  ( -50.00000000000000000, 171.6227766016838245, 0.000000000000000000 ) ) ;
#14214=DIRECTION ( 'NONE',  ( -1.156482317317868274E-16, 1.000000000000000000, 0.000000000000000000 ) ) ;
#14220=ORIENTED_EDGE ( 'NONE', *, *, #8285, .T. ) ;
#14222=DIRECTION ( 'NONE',  ( 0.000000000000000000, 0.000000000000000000, 1.000000000000000000 ) ) ;
#14223=EDGE_CURVE ( 'NONE', #9474, #11846, #17201, .T. ) ;
#14224=CARTESIAN_POINT ( 'NONE',  ( -80.00000000000002842, 146.6227766016838245, 35.00200000000000244 ) ) ;
#14225=CARTESIAN_POINT ( 'NONE',  ( 27.48361012698968864, 138.6227766016838245, 1.063447695028167043E-14 ) ) ;
#14227=CARTESIAN_POINT ( 'NONE',  ( 28.45845633961465992, 141.8618947663538279, 14.25856086977510984 ) ) ;
#14228=CARTESIAN_POINT ( 'NONE',  ( -70.00000000000000000, 154.3022685259950038, 9.999999999999900524 ) ) ;
#14233=B_SPLINE_CURVE_WITH_KNOTS ( 'NONE', 3,
 ( #15059, #13486, #14894, #13580 ),
 .UNSPECIFIED., .F., .F.,
 ( 4, 4 ),
 ( 0.000000000000000000, 0.003672568685860802366 ),
 .UNSPECIFIED. ) ;
#14241=ORIENTED_EDGE ( 'NONE', *, *, #8003, .F. ) ;
#14242=DIRECTION ( 'NONE',  ( -0.000000000000000000, -0.000000000000000000, -1.000000000000000000 ) ) ;
#14244=DIRECTION ( 'NONE',  ( -1.000000000000000000, 0.000000000000000000, 0.000000000000000000 ) ) ;
#14246=ORIENTED_EDGE ( 'NONE', *, *, #17287, .T. ) ;
#14252=DIRECTION ( 'NONE',  ( 0.000000000000000000, 0.000000000000000000, -1.000000000000000000 ) ) ;
#14253=VERTEX_POINT ( 'NONE', #3734 ) ;
#14254=CARTESIAN_POINT ( 'NONE',  ( -100.0000000000000000, 134.2062027339443944, 25.00000000000000000 ) ) ;
#14256=VERTEX_POINT ( 'NONE', #6377 ) ;
#14261=CARTESIAN_POINT ( 'NONE',  ( -26.11264420168958722, 18.00000000000000000, 13.35921939055965524 ) ) ;
#14265=ORIENTED_EDGE ( 'NONE', *, *, #12630, .T. ) ;
#14267=ORIENTED_EDGE ( 'NONE', *, *, #9705, .T. ) ;
#14271=CARTESIAN_POINT ( 'NONE',  ( -15.00000000000001421, 20.00000000000004263, 4.999999999999999112 ) ) ;
#14274=CARTESIAN_POINT ( 'NONE',  ( 19.08196460475218714, 19.99999999999773337, 14.16502029867040235 ) ) ;
#14277=CARTESIAN_POINT ( 'NONE',  ( -79.01193031122193133, 191.7175861903016312, 26.17636150746912094 ) ) ;
#14281=ADVANCED_FACE ( 'NONE', ( #7446 ), #10103, .T. ) ;
#14283=ORIENTED_EDGE ( 'NONE', *, *, #17229, .F. ) ;
#14286=CARTESIAN_POINT ( 'NONE',  ( -85.00000000000002842, 196.6227766016838245, 0.000000000000000000 ) ) ;
#14287=VERTEX_POINT ( 'NONE', #15509 ) ;
#14289=VECTOR ( 'NONE', #15228, 1000.000000000000000 ) ;
#14292=EDGE_LOOP ( 'NONE', ( #13882, #4072, #12398, #3750 ) ) ;
#14297=CARTESIAN_POINT ( 'NONE',  ( -13.22984127103138796, 31.85746429949665881, 11.06592603413638898 ) ) ;
#14300=CARTESIAN_POINT ( 'NONE',  ( 48.00000000000000711, 163.6227766016838530, 15.00000337241049486 ) ) ;
#14302=CARTESIAN_POINT ( 'NONE',  ( -45.00000000000000000, 136.6227766016838245, 0.000000000000000000 ) ) ;
#14305=DIRECTION ( 'NONE',  ( 8.673617379884037937E-17, 0.000000000000000000, -1.000000000000000000 ) ) ;
#14307=FACE_OUTER_BOUND ( 'NONE', #14201, .T. ) ;
#14309=AXIS2_PLACEMENT_3D ( 'NONE', #830, #11971, #13215 ) ;
#14311=VECTOR ( 'NONE', #12447, 1000.000000000000000 ) ;
#14312=EDGE_CURVE ( 'NONE', #16894, #14086, #4881, .T. ) ;
#14318=ORIENTED_EDGE ( 'NONE', *, *, #16898, .F. ) ;
#14322=CARTESIAN_POINT ( 'NONE',  ( -23.00000000000000000, 122.0000000000000284, 0.000000000000000000 ) ) ;
#14323=ADVANCED_FACE ( 'NONE', ( #9120 ), #7788, .F. ) ;
#14324=DIRECTION ( 'NONE',  ( -1.000000000000000000, -0.000000000000000000, -0.000000000000000000 ) ) ;
#14325=AXIS2_PLACEMENT_3D ( 'NONE', #15642, #3517, #9976 ) ;
#14328=CARTESIAN_POINT ( 'NONE',  ( -5.000000000000004441, 134.2062027339443944, 25.00000000000000000 ) ) ;
#14333=ORIENTED_EDGE ( 'NONE', *, *, #16098, .F. ) ;
#14339=CARTESIAN_POINT ( 'NONE',  ( 196.0000000000000000, 155.6227766016839098, 12.50000337241049309 ) ) ;
#14345=EDGE_CURVE ( 'NONE', #12401, #9730, #729, .T. ) ;
#14348=DIRECTION ( 'NONE',  ( -0.000000000000000000, -0.000000000000000000, -1.000000000000000000 ) ) ;
#14349=CARTESIAN_POINT ( 'NONE',  ( 48.00000000000000711, 167.6227766016838814, 19.42820660268601074 ) ) ;
#14350=CARTESIAN_POINT ( 'NONE',  ( -11.84409501751983207, 17.99999999999999645, 9.388895791866135099 ) ) ;
#14359=DIRECTION ( 'NONE',  ( 2.312964634635742464E-16, 0.000000000000000000, -1.000000000000000000 ) ) ;
#14362=CARTESIAN_POINT ( 'NONE',  ( 17.55923266082603007, 19.99999999999999645, 24.87049340120105612 ) ) ;
#14363=CARTESIAN_POINT ( 'NONE',  ( 12.23870813552851722, 139.5070109101417302, 10.31054875319067143 ) ) ;
#14364=AXIS2_PLACEMENT_3D ( 'NONE', #5269, #15083, #10764 ) ;
#14365=CARTESIAN_POINT ( 'NONE',  ( 32.90650748920315039, 19.99999999999999645, 13.87185692902932921 ) ) ;
#14368=ORIENTED_EDGE ( 'NONE', *, *, #4441, .T. ) ;
#14369=EDGE_CURVE ( 'NONE', #6576, #3421, #13110, .T. ) ;
#14370=EDGE_CURVE ( 'NONE', #14513, #12401, #9278, .T. ) ;
#14371=EDGE_CURVE ( 'NONE', #14379, #4320, #11682, .T. ) ;
#14374=DIRECTION ( 'NONE',  ( -1.000000000000000000, 0.000000000000000000, 0.000000000000000000 ) ) ;
#14377=CARTESIAN_POINT ( 'NONE',  ( 48.00000000000000711, 151.6227766016839098, 5.571800142134973655 ) ) ;
#14379=VERTEX_POINT ( 'NONE', #10452 ) ;
#14384=VERTEX_POINT ( 'NONE', #15860 ) ;
#14385=ORIENTED_EDGE ( 'NONE', *, *, #16931, .F. ) ;
#14389=AXIS2_PLACEMENT_3D ( 'NONE', #11407, #3363, #2032 ) ;
#14390=ORIENTED_EDGE ( 'NONE', *, *, #9045, .F. ) ;
#14394=CARTESIAN_POINT ( 'NONE',  ( -14.33532356861720380, 31.51408589783374126, 12.70909354450696149 ) ) ;
#14395=DIRECTION ( 'NONE',  ( -0.000000000000000000, -0.000000000000000000, -1.000000000000000000 ) ) ;
#14396=CARTESIAN_POINT ( 'NONE',  ( 23.09107716925733911, 17.99999999999999645, 5.000000000000003553 ) ) ;
#14397=CARTESIAN_POINT ( 'NONE',  ( 27.47046887122067105, 138.6908793960143669, 2.448156880351273657 ) ) ;
#14398=ORIENTED_EDGE ( 'NONE', *, *, #8565, .F. ) ;
#14399=CARTESIAN_POINT ( 'NONE',  ( 16.87754908408646415, 142.8876428028120813, 16.22928829806427942 ) ) ;
#14400=LINE ( 'NONE', #11307, #16677 ) ;
#14401=DIRECTION ( 'NONE',  ( -1.156482317317868274E-16, 1.000000000000000000, 0.000000000000000000 ) ) ;
#14402=CARTESIAN_POINT ( 'NONE',  ( 24.29886777166023393, 29.87658293154515832, 8.524716167024733338 ) ) ;
#14407=CIRCLE ( 'NONE', #12992, 20.00000000000000355 ) ;
#14409=ORIENTED_EDGE ( 'NONE', *, *, #5922, .T. ) ;
#14414=CARTESIAN_POINT ( 'NONE',  ( -77.32048138630932499, 142.3872899932706559, 15.31067380954019796 ) ) ;
#14417=AXIS2_PLACEMENT_3D ( 'NONE', #4862, #883, #14244 ) ;
#14422=ORIENTED_EDGE ( 'NONE', *, *, #12303, .T. ) ;
#14424=CARTESIAN_POINT ( 'NONE',  ( 49.99999999999998579, 191.6227766016837677, 5.571800142134975431 ) ) ;
#14425=DIRECTION ( 'NONE',  ( -1.000000000000000000, 0.000000000000000000, 0.000000000000000000 ) ) ;
#14427=ORIENTED_EDGE ( 'NONE', *, *, #3215, .T. ) ;
#14428=ORIENTED_EDGE ( 'NONE', *, *, #15036, .T. ) ;
#14431=CIRCLE ( 'NONE', #2570, 2.500000000000002220 ) ;
#14432=DIRECTION ( 'NONE',  ( 0.000000000000000000, -0.000000000000000000, -1.000000000000000000 ) ) ;
#14437=ORIENTED_EDGE ( 'NONE', *, *, #13556, .T. ) ;
#14438=CARTESIAN_POINT ( 'NONE',  ( 17.00000000000000000, 154.3022685259950038, 9.999999999999900524 ) ) ;
#14443=CARTESIAN_POINT ( 'NONE',  ( -26.90043998675938397, 18.00000000000000000, 11.53672424425030840 ) ) ;
#14445=DIRECTION ( 'NONE',  ( -0.8660254037844378194, -0.5000000000000015543, -0.000000000000000000 ) ) ;
#14446=VERTEX_POINT ( 'NONE', #13378 ) ;
#14448=ORIENTED_EDGE ( 'NONE', *, *, #12304, .F. ) ;
#14453=CARTESIAN_POINT ( 'NONE',  ( -9.703671380219899945, 20.00000000000115463, 14.18606485937966788 ) ) ;
#14454=CARTESIAN_POINT ( 'NONE',  ( 7.010070850708371992, 140.5745599005093425, 12.93128425349117983 ) ) ;
#14455=CARTESIAN_POINT ( 'NONE',  ( 24.40970717605596718, 29.87515913883691354, 8.215055496182330330 ) ) ;
#14458=DIRECTION ( 'NONE',  ( 1.000000000000000000, 0.000000000000000000, -0.000000000000000000 ) ) ;
#14466=DIRECTION ( 'NONE',  ( -1.000000000000000000, -0.000000000000000000, 0.000000000000000000 ) ) ;
#14467=EDGE_CURVE ( 'NONE', #15051, #2616, #17276, .T. ) ;
#14469=EDGE_CURVE ( 'NONE', #5700, #9733, #6463, .T. ) ;
#14470=ORIENTED_EDGE ( 'NONE', *, *, #15585, .F. ) ;
#14471=EDGE_CURVE ( 'NONE', #15093, #12155, #1165, .T. ) ;
#14477=CARTESIAN_POINT ( 'NONE',  ( 27.99999999999998224, 9.999999999999998224, 10.00000000000000178 ) ) ;
#14479=CARTESIAN_POINT ( 'NONE',  ( 34.42312820349192037, 18.00000000000000000, 9.539278825333477485 ) ) ;
#14480=CARTESIAN_POINT ( 'NONE',  ( 15.58935622847965163, 125.0306600298041815, 3.338394242842863679 ) ) ;
#14481=EDGE_LOOP ( 'NONE', ( #6241, #7914, #400, #7556, #15319, #10387 ) ) ;
#14482=CARTESIAN_POINT ( 'NONE',  ( 27.04079503965286690, 139.2301514590222098, 6.313402927548398047 ) ) ;
#14485=CARTESIAN_POINT ( 'NONE',  ( 33.66231827095856488, 18.00000000000000000, 12.04861179558545636 ) ) ;
#14486=CARTESIAN_POINT ( 'NONE',  ( -40.00000000000000000, 4.000000000000000000, 30.00000000000000711 ) ) ;
#14489=CARTESIAN_POINT ( 'NONE',  ( 35.00000000000000000, 196.6227766016838245, 21.54065922853802206 ) ) ;
#14492=CARTESIAN_POINT ( 'NONE',  ( 25.00000000000000000, 196.6227766016838245, 21.54065922853802562 ) ) ;
#14495=CARTESIAN_POINT ( 'NONE',  ( -81.14508075249469243, 141.7513145237122671, 14.02541974480121567 ) ) ;
#14499=VERTEX_POINT ( 'NONE', #4087 ) ;
#14507=ORIENTED_EDGE ( 'NONE', *, *, #15931, .F. ) ;
#14511=ADVANCED_FACE ( 'NONE', ( #6833 ), #1073, .T. ) ;
#14513=VERTEX_POINT ( 'NONE', #3817 ) ;
#14514=CARTESIAN_POINT ( 'NONE',  ( -40.00000000000000000, 0.000000000000000000, 33.00000000000000711 ) ) ;
#14515=DIRECTION ( 'NONE',  ( -1.000000000000000000, -0.000000000000000000, -0.000000000000000000 ) ) ;
#14517=CARTESIAN_POINT ( 'NONE',  ( 34.83135640459488513, 195.3043783022528146, 22.98536326679100128 ) ) ;
#14520=DIRECTION ( 'NONE',  ( 0.000000000000000000, 8.410780489584519664E-16, -1.000000000000000000 ) ) ;
#14521=CARTESIAN_POINT ( 'NONE',  ( 34.93420767853316988, 18.00000000000000355, 4.999999999999999112 ) ) ;
#14522=ORIENTED_EDGE ( 'NONE', *, *, #15425, .F. ) ;
#14528=EDGE_CURVE ( 'NONE', #2606, #4609, #12397, .T. ) ;
#14529=CARTESIAN_POINT ( 'NONE',  ( -77.50000000000001421, 196.6227766016838245, 0.000000000000000000 ) ) ;
#14530=EDGE_CURVE ( 'NONE', #13670, #2134, #11824, .T. ) ;
#14531=DIRECTION ( 'NONE',  ( -1.000000000000000000, -0.000000000000000000, -0.000000000000000000 ) ) ;
#14532=ORIENTED_EDGE ( 'NONE', *, *, #3825, .T. ) ;
#14535=ORIENTED_EDGE ( 'NONE', *, *, #17264, .F. ) ;
#14536=CIRCLE ( 'NONE', #15954, 5.000000000000000888 ) ;
#14539=DIRECTION ( 'NONE',  ( 0.000000000000000000, 0.8660254037844413721, -0.4999999999999952816 ) ) ;
#14542=ORIENTED_EDGE ( 'NONE', *, *, #5450, .T. ) ;
#14546=CARTESIAN_POINT ( 'NONE',  ( 39.99999999999998579, 0.000000000000000000, 30.00000000000001066 ) ) ;
#14553=ORIENTED_EDGE ( 'NONE', *, *, #12480, .T. ) ;
#14556=PLANE ( 'NONE',  #14726 ) ;
#14557=CARTESIAN_POINT ( 'NONE',  ( -10.71009414332545973, 30.74249144840758063, 14.53036023671900168 ) ) ;
#14561=CARTESIAN_POINT ( 'NONE',  ( 33.66001102075319551, 18.00000000000000000, 12.05479157725487482 ) ) ;
#14562=EDGE_CURVE ( 'NONE', #6919, #9322, #10965, .T. ) ;
#14563=DIRECTION ( 'NONE',  ( -0.000000000000000000, -0.000000000000000000, 1.000000000000000000 ) ) ;
#14567=FACE_OUTER_BOUND ( 'NONE', #11116, .T. ) ;
#14568=FACE_OUTER_BOUND ( 'NONE', #4062, .T. ) ;
#14570=DIRECTION ( 'NONE',  ( -1.000000000000000000, -0.000000000000000000, -0.000000000000000000 ) ) ;
#14573=CARTESIAN_POINT ( 'NONE',  ( 0.000000000000000000, 0.000000000000000000, 33.00000000000000711 ) ) ;
#14574=CIRCLE ( 'NONE', #4415, 2.500000000000002220 ) ;
#14579=EDGE_LOOP ( 'NONE', ( #14692, #9684 ) ) ;
#14581=CARTESIAN_POINT ( 'NONE',  ( -84.01578204813917239, 143.6297497249236415, 17.48070775079457917 ) ) ;
#14585=CARTESIAN_POINT ( 'NONE',  ( -725.0000000000000000, 134.2062027339443944, 13.00000000000000000 ) ) ;
#14593=CARTESIAN_POINT ( 'NONE',  ( -100.0000000000000000, 144.1839557653416080, 18.33333333333335702 ) ) ;
#14594=VERTEX_POINT ( 'NONE', #14486 ) ;
#14595=ORIENTED_EDGE ( 'NONE', *, *, #16042, .F. ) ;
#14604=VECTOR ( 'NONE', #9114, 1000.000000000000000 ) ;
#14607=DIRECTION ( 'NONE',  ( -0.000000000000000000, -0.000000000000000000, -1.000000000000000000 ) ) ;
#14608=DIRECTION ( 'NONE',  ( -1.000000000000000000, 0.000000000000000000, 0.000000000000000000 ) ) ;
#14611=CARTESIAN_POINT ( 'NONE',  ( -95.00000000000000000, 171.6227766016838245, 0.000000000000000000 ) ) ;
#14613=CARTESIAN_POINT ( 'NONE',  ( 225.0000000000000000, 89.99999999999997158, 13.00000000000000000 ) ) ;
#14619=ORIENTED_EDGE ( 'NONE', *, *, #15870, .T. ) ;
#14625=CARTESIAN_POINT ( 'NONE',  ( -7.379000772444995526, 30.00000000000000000, 15.00000000000000355 ) ) ;
#14626=CARTESIAN_POINT ( 'NONE',  ( 11.37136921290580460, 130.9041960856249318, 11.49611652308843901 ) ) ;
#14631=AXIS2_PLACEMENT_3D ( 'NONE', #12204, #2900, #1667 ) ;
#14633=CARTESIAN_POINT ( 'NONE',  ( -75.00000000000002842, 146.6227766016838245, 21.54065922853802562 ) ) ;
#14637=EDGE_CURVE ( 'NONE', #9979, #5404, #9350, .T. ) ;
#14640=DIRECTION ( 'NONE',  ( 0.000000000000000000, 0.000000000000000000, -1.000000000000000000 ) ) ;
#14644=EDGE_LOOP ( 'NONE', ( #5979, #12045, #12884, #5715 ) ) ;
#14645=CONICAL_SURFACE ( 'NONE', #8720, 2.499999999999998668, 1.029744260000002187 ) ;
#14646=ORIENTED_EDGE ( 'NONE', *, *, #3347, .F. ) ;
#14651=ORIENTED_EDGE ( 'NONE', *, *, #6974, .T. ) ;
#14652=CARTESIAN_POINT ( 'NONE',  ( 0.000000000000000000, 2.000000000000000000, 0.000000000000000000 ) ) ;
#14653=CARTESIAN_POINT ( 'NONE',  ( -18.15427578192114666, 32.28835078156378557, 6.388283290543781412 ) ) ;
#14654=DIRECTION ( 'NONE',  ( -0.8571673013836870192, 0.000000000000000000, -0.5150380737757234151 ) ) ;
#14664=CARTESIAN_POINT ( 'NONE',  ( 19.36310082087489803, 29.94084738964976111, 13.97143931599698874 ) ) ;
#14665=EDGE_LOOP ( 'NONE', ( #14246, #15400, #8968, #9413 ) ) ;
#14668=DIRECTION ( 'NONE',  ( -1.000000000000000000, 0.000000000000000000, 0.000000000000000000 ) ) ;
#14669=EDGE_CURVE ( 'NONE', #5075, #12878, #6872, .T. ) ;
#14670=EDGE_CURVE ( 'NONE', #6919, #13751, #139, .T. ) ;
#14671=ORIENTED_EDGE ( 'NONE', *, *, #9211, .F. ) ;
#14673=VECTOR ( 'NONE', #12696, 1000.000000000000000 ) ;
#14676=DIRECTION ( 'NONE',  ( 0.000000000000000000, 0.000000000000000000, -1.000000000000000000 ) ) ;
#14677=CARTESIAN_POINT ( 'NONE',  ( -27.98221281347037959, 18.00000000000000355, 4.999999999999999112 ) ) ;
#14680=VERTEX_POINT ( 'NONE', #58 ) ;
#14689=ADVANCED_FACE ( 'NONE', ( #2712 ), #2628, .F. ) ;
#14692=ORIENTED_EDGE ( 'NONE', *, *, #5123, .F. ) ;
#14697=EDGE_LOOP ( 'NONE', ( #5865, #208 ) ) ;
#14698=CARTESIAN_POINT ( 'NONE',  ( 196.0000000000000000, 187.6227766016837961, 12.50000337241049309 ) ) ;
#14704=( BOUNDED_CURVE ( )  B_SPLINE_CURVE ( 3, ( #12344, #12253, #47, #2954 ),
 .UNSPECIFIED., .F., .F. ) 
 B_SPLINE_CURVE_WITH_KNOTS ( ( 4, 4 ),
 ( 3.141592653589792672, 4.712388980384690562 ),
 .UNSPECIFIED. ) 
 CURVE ( )  GEOMETRIC_REPRESENTATION_ITEM ( )  RATIONAL_B_SPLINE_CURVE ( ( 1.000000000000000000, 0.8047378541243646044, 0.8047378541243646044, 1.000000000000000000 ) ) 
 REPRESENTATION_ITEM ( '' )  );
#14706=DIRECTION ( 'NONE',  ( -1.000000000000000000, -0.000000000000000000, -0.000000000000000000 ) ) ;
#14707=PLANE ( 'NONE',  #13834 ) ;
#14711=DIRECTION ( 'NONE',  ( 1.000000000000000000, 6.938893903907228378E-16, -0.000000000000000000 ) ) ;
#14712=VECTOR ( 'NONE', #12006, 1000.000000000000000 ) ;
#14714=ORIENTED_EDGE ( 'NONE', *, *, #16570, .T. ) ;
#14715=ADVANCED_FACE ( 'NONE', ( #1477 ), #5541, .T. ) ;
#14716=DIRECTION ( 'NONE',  ( -1.000000000000000000, -0.000000000000000000, -0.000000000000000000 ) ) ;
#14720=CARTESIAN_POINT ( 'NONE',  ( -43.00000000000000000, 138.6227766016838245, 0.000000000000000000 ) ) ;
#14721=CARTESIAN_POINT ( 'NONE',  ( 26.46962346220079709, 139.5657242622003480, 7.835998493359402239 ) ) ;
#14722=ORIENTED_EDGE ( 'NONE', *, *, #4926, .F. ) ;
#14723=CARTESIAN_POINT ( 'NONE',  ( 18.15033819753324806, 29.95689775512239805, 14.47405640211066213 ) ) ;
#14726=AXIS2_PLACEMENT_3D ( 'NONE', #13236, #12436, #14745 ) ;
#14728=CARTESIAN_POINT ( 'NONE',  ( -725.0000000000000000, 30.00000000000000000, 25.00000000000000000 ) ) ;
#14731=VERTEX_POINT ( 'NONE', #8013 ) ;
#14732=CARTESIAN_POINT ( 'NONE',  ( 33.65445145306948405, 150.0509117818997424, 24.97535314687242902 ) ) ;
#14740=EDGE_LOOP ( 'NONE', ( #17277, #13221, #9280, #4040 ) ) ;
#14743=VERTEX_POINT ( 'NONE', #13778 ) ;
#14745=DIRECTION ( 'NONE',  ( 1.000000000000000000, 0.000000000000000000, -0.000000000000000000 ) ) ;
#14746=CARTESIAN_POINT ( 'NONE',  ( -14.60673078645093703, 31.57037919282903360, 12.49506642855920724 ) ) ;
#14748=AXIS2_PLACEMENT_3D ( 'NONE', #14206, #7808, #15783 ) ;
#14750=CARTESIAN_POINT ( 'NONE',  ( -77.43519705649855212, 150.9309764409412651, 25.70786830908635068 ) ) ;
#14758=DIRECTION ( 'NONE',  ( -1.000000000000000000, 0.000000000000000000, 0.000000000000000000 ) ) ;
#14762=ADVANCED_FACE ( 'NONE', ( #6698 ), #15513, .T. ) ;
#14768=CARTESIAN_POINT ( 'NONE',  ( -26.10410744458348020, 20.00000000000000000, 13.37721135299797659 ) ) ;
#14770=CARTESIAN_POINT ( 'NONE',  ( 39.99999999999998579, 20.00000000000000000, 30.00000000000001066 ) ) ;
#14771=LINE ( 'NONE', #14848, #1970 ) ;
#14772=EDGE_CURVE ( 'NONE', #12728, #1301, #8451, .T. ) ;
#14782=CARTESIAN_POINT ( 'NONE',  ( 196.0000000000000000, 191.6227766016837677, 5.571800142134975431 ) ) ;
#14783=CARTESIAN_POINT ( 'NONE',  ( 34.98026256913478704, 196.1036955441147995, 22.13227804827259959 ) ) ;
#14786=CARTESIAN_POINT ( 'NONE',  ( -48.00000000000000000, 154.3022685259950038, 9.999999999999900524 ) ) ;
#14788=ADVANCED_FACE ( 'NONE', ( #16701 ), #8458, .F. ) ;
#14791=EDGE_CURVE ( 'NONE', #13335, #5075, #5627, .T. ) ;
#14795=ORIENTED_EDGE ( 'NONE', *, *, #13389, .T. ) ;
#14796=DIRECTION ( 'NONE',  ( -0.000000000000000000, -0.000000000000000000, -1.000000000000000000 ) ) ;
#14797=FACE_BOUND ( 'NONE', #2891, .T. ) ;
#14798=VERTEX_POINT ( 'NONE', #11287 ) ;
#14799=CARTESIAN_POINT ( 'NONE',  ( -11.67692690462290273, 19.99999999999766587, 12.94410612366815272 ) ) ;
#14800=CARTESIAN_POINT ( 'NONE',  ( 14.46714703242257904, 138.5709836085849531, 4.391619799164913296 ) ) ;
#14802=CARTESIAN_POINT ( 'NONE',  ( 16.23418548573199516, 29.98246013044581915, 14.93677958672484785 ) ) ;
#14803=( BOUNDED_SURFACE ( )  B_SPLINE_SURFACE ( 3, 2, ( 
 ( #2321, #15681, #14199 ),
 ( #4636, #16941, #649 ),
 ( #3563, #4887, #14115 ),
 ( #986, #15429, #4974 ),
 ( #9047, #11688, #8706 ),
 ( #11529, #8955, #14455 ),
 ( #2143, #6046, #10205 ),
 ( #14365, #3305, #12953 ),
 ( #11359, #10110, #912 ),
 ( #17023, #17103, #10367 ),
 ( #2236, #7712, #10015 ),
 ( #11619, #7543, #7629 ),
 ( #13120, #6221, #13043 ),
 ( #10278, #1977, #15777 ),
 ( #6300, #15601, #11439 ),
 ( #7381, #12779, #16850 ),
 ( #3479, #15518, #4722 ),
 ( #8793, #2060, #738 ),
 ( #6134, #14274, #828 ),
 ( #4096, #10641, #9399 ),
 ( #24, #5067, #14723 ),
 ( #16228, #14887, #10733 ),
 ( #10817, #17192, #11968 ),
 ( #3926, #9476, #15951 ),
 ( #13478, #9220, #6663 ),
 ( #3830, #10462, #14802 ),
 ( #5428, #10545, #17285 ),
 ( #6485, #2502, #5239 ) ),
 .UNSPECIFIED., .F., .F., .F. ) 
 B_SPLINE_SURFACE_WITH_KNOTS ( ( 4, 2, 2, 2, 2, 2, 2, 2, 2, 2, 2, 2, 2, 4 ),
 ( 3, 3 ),
 ( 0.01342997177288654184, 0.01733910390705691029, 0.01929366997414209278, 0.02124823604122727527, 0.02515736817539764372, 0.02711193424248282968, 0.02906650030956801217, 0.03297563244373838409, 0.03493019851082356658, 0.03688476457790874907, 0.03883933064499393156, 0.03981661367853651934, 0.04079389671207911405, 0.04470302884624948597 ),
 ( 0.000000000000000000, 1.000000000000000000 ),
 .UNSPECIFIED. ) 
 GEOMETRIC_REPRESENTATION_ITEM ( )  RATIONAL_B_SPLINE_SURFACE ( (
 ( 1.000000000000000000, 0.7117435966472906994, 1.000000000000000000),
 ( 1.000000000000000000, 0.7117434842622788471, 1.000000000000000000),
 ( 1.000000000000000000, 0.7117144184576317256, 1.000000000000000000),
 ( 1.000000000000000000, 0.7116285301813536357, 1.000000000000000000),
 ( 1.000000000000000000, 0.7115928256594988843, 1.000000000000000000),
 ( 1.000000000000000000, 0.7115068832447583036, 1.000000000000000000),
 ( 1.000000000000000000, 0.7114564033771691998, 1.000000000000000000),
 ( 1.000000000000000000, 0.7112861117250206533, 1.000000000000000000),
 ( 1.000000000000000000, 0.7111469280185451769, 1.000000000000000000),
 ( 1.000000000000000000, 0.7108993804763810154, 1.000000000000000000),
 ( 1.000000000000000000, 0.7108100171490498997, 1.000000000000000000),
 ( 1.000000000000000000, 0.7106191415567917335, 1.000000000000000000),
 ( 1.000000000000000000, 0.7105185320923617098, 1.000000000000000000),
 ( 1.000000000000000000, 0.7102014790723296667, 1.000000000000000000),
 ( 1.000000000000000000, 0.7099699576741209661, 1.000000000000000000),
 ( 1.000000000000000000, 0.7095909300314675594, 1.000000000000000000),
 ( 1.000000000000000000, 0.7094593121158619953, 1.000000000000000000),
 ( 1.000000000000000000, 0.7091910831478104305, 1.000000000000000000),
 ( 1.000000000000000000, 0.7090537746377190143, 1.000000000000000000),
 ( 1.000000000000000000, 0.7087727591781516345, 1.000000000000000000),
 ( 1.000000000000000000, 0.7086290523620303317, 1.000000000000000000),
 ( 1.000000000000000000, 0.7084085592173990920, 1.000000000000000000),
 ( 1.000000000000000000, 0.7083342380282030559, 1.000000000000000000),
 ( 1.000000000000000000, 0.7081839094108949295, 1.000000000000000000),
 ( 1.000000000000000000, 0.7081077478408516201, 1.000000000000000000),
 ( 1.000000000000000000, 0.7077267031859736379, 1.000000000000000000),
 ( 1.000000000000000000, 0.7074184602292508117, 1.000000000000000000),
 ( 1.000000000000000000, 0.7071067811865475727, 1.000000000000000000) ) ) 
 REPRESENTATION_ITEM ( '' )  SURFACE ( )  );
#14810=CARTESIAN_POINT ( 'NONE',  ( 34.83193525651911671, 147.9395323639054141, 22.98372036160736798 ) ) ;
#14813=CARTESIAN_POINT ( 'NONE',  ( -27.99999999999998224, 10.00000000000000000, 10.00000000000000178 ) ) ;
#14814=ORIENTED_EDGE ( 'NONE', *, *, #6974, .F. ) ;
#14815=ORIENTED_EDGE ( 'NONE', *, *, #11755, .T. ) ;
#14816=ORIENTED_EDGE ( 'NONE', *, *, #16570, .F. ) ;
#14822=EDGE_CURVE ( 'NONE', #1044, #7220, #8723, .T. ) ;
#14823=CARTESIAN_POINT ( 'NONE',  ( 34.93420767853316988, 30.00000000000000000, 4.999999999999999112 ) ) ;
#14826=CARTESIAN_POINT ( 'NONE',  ( -81.55625601990109885, 151.3901271056993210, 26.07015880384263085 ) ) ;
#14830=CARTESIAN_POINT ( 'NONE',  ( 9.788850454972870097, 132.9181049171561995, 14.40474131580982231 ) ) ;
#14831=CARTESIAN_POINT ( 'NONE',  ( 19.49710218362280045, 17.99999999999999289, 24.48336163992366465 ) ) ;
#14833=PLANE ( 'NONE',  #15424 ) ;
#14839=EDGE_LOOP ( 'NONE', ( #10307, #6932, #5935, #6437 ) ) ;
#14840=CARTESIAN_POINT ( 'NONE',  ( -30.49999999999998224, 10.00000000000000000, 0.000000000000000000 ) ) ;
#14842=CARTESIAN_POINT ( 'NONE',  ( -40.00000000000000000, 4.000000000000000000, 33.00000000000000711 ) ) ;
#14844=CARTESIAN_POINT ( 'NONE',  ( -14.54670497998687217, 20.00000000000000000, 23.76610458325320607 ) ) ;
#14845=VERTEX_POINT ( 'NONE', #16867 ) ;
#14848=CARTESIAN_POINT ( 'NONE',  ( 39.99999999999998579, 20.00000000000000000, 30.00000000000001066 ) ) ;
#14851=SURFACE_SIDE_STYLE ('',( #4067 ) ) ;
#14861=EDGE_CURVE ( 'NONE', #14086, #3946, #13548, .T. ) ;
#14866=DIRECTION ( 'NONE',  ( 0.000000000000000000, 0.000000000000000000, 1.000000000000000000 ) ) ;
#14867=CARTESIAN_POINT ( 'NONE',  ( 34.89574631506663849, 195.5720014495397265, 22.70655749026626680 ) ) ;
#14870=CARTESIAN_POINT ( 'NONE',  ( 196.0000000000000000, 175.6227766016838530, 19.42820660268601074 ) ) ;
#14877=CYLINDRICAL_SURFACE ( 'NONE', #9762, 20.00000000000000355 ) ;
#14881=ORIENTED_EDGE ( 'NONE', *, *, #11083, .F. ) ;
#14887=CARTESIAN_POINT ( 'NONE',  ( 17.69056612348262192, 20.00000000000056488, 14.65191630173004711 ) ) ;
#14888=EDGE_CURVE ( 'NONE', #8372, #1583, #16784, .T. ) ;
#14894=CARTESIAN_POINT ( 'NONE',  ( 27.48361012698976324, 138.6227766016838245, 1.226160068396871639 ) ) ;
#14897=CARTESIAN_POINT ( 'NONE',  ( -5.000000000000000888, 171.6227766016838245, 20.00000000000000355 ) ) ;
#14901=PLANE ( 'NONE',  #3569 ) ;
#14904=ORIENTED_EDGE ( 'NONE', *, *, #968, .F. ) ;
#14905=ADVANCED_FACE ( 'NONE', ( #8810 ), #7876, .F. ) ;
#14907=AXIS2_PLACEMENT_3D ( 'NONE', #16651, #2105, #8758 ) ;
#14908=CARTESIAN_POINT ( 'NONE',  ( 8.904477399772744661, 142.4465447428235620, 19.33413753149157088 ) ) ;
#14910=AXIS2_PLACEMENT_3D ( 'NONE', #494, #8551, #16712 ) ;
#14912=CARTESIAN_POINT ( 'NONE',  ( 30.49999999999998224, 9.999999999999998224, 10.00000000000000178 ) ) ;
#14916=FACE_BOUND ( 'NONE', #14697, .T. ) ;
#14919=CARTESIAN_POINT ( 'NONE',  ( 48.00000000000000711, 191.6227766016837677, 5.571800142134975431 ) ) ;
#14923=CARTESIAN_POINT ( 'NONE',  ( 24.93507336697364707, 29.86842105263157876, 15.00000000000000000 ) ) ;
#14924=CARTESIAN_POINT ( 'NONE',  ( -50.00000000000000000, 171.6227766016838245, 20.00000000000000355 ) ) ;
#14926=ORIENTED_EDGE ( 'NONE', *, *, #15904, .F. ) ;
#14930=CARTESIAN_POINT ( 'NONE',  ( -70.00000000000000000, 204.6227766016838245, -2.020667218593133100E-15 ) ) ;
#14934=FACE_OUTER_BOUND ( 'NONE', #4949, .T. ) ;
#14940=VECTOR ( 'NONE', #2313, 1000.000000000000000 ) ;
#14945=FACE_BOUND ( 'NONE', #10216, .T. ) ;
#14951=EDGE_CURVE ( 'NONE', #6665, #11003, #4196, .T. ) ;
#14954=AXIS2_PLACEMENT_3D ( 'NONE', #11191, #11456, #484 ) ;
#14955=CARTESIAN_POINT ( 'NONE',  ( 31.90657348432143792, 191.9854139975491023, 25.96938468333276973 ) ) ;
#14957=FACE_OUTER_BOUND ( 'NONE', #5393, .T. ) ;
#14959=CARTESIAN_POINT ( 'NONE',  ( -3.000000000000000888, 171.6227766016838245, 20.00000000000000355 ) ) ;
#14965=LINE ( 'NONE', #17, #9594 ) ;
#14969=ORIENTED_EDGE ( 'NONE', *, *, #4304, .F. ) ;
#14970=CARTESIAN_POINT ( 'NONE',  ( -17.68452897573239824, 32.19524659542067013, 8.268362122121875046 ) ) ;
#14971=AXIS2_PLACEMENT_3D ( 'NONE', #12763, #8774, #15499 ) ;
#14980=EDGE_LOOP ( 'NONE', ( #4737, #14553, #13993, #1442 ) ) ;
#14982=TOROIDAL_SURFACE ( 'NONE', #8770, 240.0000000000000000, 8.000000000000000000 ) ;
#14984=CARTESIAN_POINT ( 'NONE',  ( 34.31805984300264356, 149.1480937705749170, 24.16447509748838840 ) ) ;
#14985=EDGE_CURVE ( 'NONE', #13756, #3929, #13666, .T. ) ;
#14987=CARTESIAN_POINT ( 'NONE',  ( 37.99999999999999289, 18.00000000000000355, 8.789265611615818404E-15 ) ) ;
#14988=CARTESIAN_POINT ( 'NONE',  ( -80.00000000000001421, 196.6227766016838245, 0.000000000000000000 ) ) ;
#14991=EDGE_LOOP ( 'NONE', ( #14422, #642, #12749, #9356 ) ) ;
#14992=CIRCLE ( 'NONE', #5099, 2.500000000000002220 ) ;
#14993=CIRCLE ( 'NONE', #16704, 2.499999999999998668 ) ;
#14995=CARTESIAN_POINT ( 'NONE',  ( 49.99999999999998579, 167.6227766016838530, 5.571800142134975431 ) ) ;
#15001=DIRECTION ( 'NONE',  ( 1.000000000000000000, 0.000000000000000000, 0.000000000000000000 ) ) ;
#15003=EDGE_LOOP ( 'NONE', ( #7845, #8875, #7832, #15261 ) ) ;
#15007=ADVANCED_FACE ( 'NONE', ( #4032 ), #13269, .F. ) ;
#15013=VERTEX_POINT ( 'NONE', #17479 ) ;
#15014=LINE ( 'NONE', #6875, #10176 ) ;
#15015=ORIENTED_EDGE ( 'NONE', *, *, #17384, .T. ) ;
#15018=ORIENTED_EDGE ( 'NONE', *, *, #5815, .F. ) ;
#15023=LINE ( 'NONE', #6882, #8407 ) ;
#15024=DIRECTION ( 'NONE',  ( 1.000000000000000000, 0.000000000000000000, -0.000000000000000000 ) ) ;
#15036=EDGE_CURVE ( 'NONE', #5017, #2637, #6769, .T. ) ;
#15041=CARTESIAN_POINT ( 'NONE',  ( -85.00000000000002842, 146.6227766016838245, 0.000000000000000000 ) ) ;
#15045=DIRECTION ( 'NONE',  ( -1.000000000000000000, 0.000000000000000000, 0.000000000000000000 ) ) ;
#15046=ADVANCED_FACE ( 'NONE', ( #11260 ), #7023, .F. ) ;
#15047=DIRECTION ( 'NONE',  ( 0.000000000000000000, 0.000000000000000000, 1.000000000000000000 ) ) ;
#15049=CARTESIAN_POINT ( 'NONE',  ( -17.27091434876127707, 32.11264161353675917, 9.179609695281474302 ) ) ;
#15051=VERTEX_POINT ( 'NONE', #15419 ) ;
#15058=ORIENTED_EDGE ( 'NONE', *, *, #5249, .T. ) ;
#15059=CARTESIAN_POINT ( 'NONE',  ( 27.44407568426044008, 138.8271129316868837, 3.666666666666658081 ) ) ;
#15062=DIRECTION ( 'NONE',  ( 0.000000000000000000, 0.000000000000000000, -1.000000000000000000 ) ) ;
#15063=EDGE_CURVE ( 'NONE', #15578, #14384, #4716, .T. ) ;
#15064=ORIENTED_EDGE ( 'NONE', *, *, #17303, .F. ) ;
#15065=EDGE_CURVE ( 'NONE', #12692, #17091, #15161, .T. ) ;
#15069=FACE_OUTER_BOUND ( 'NONE', #9670, .T. ) ;
#15071=ORIENTED_EDGE ( 'NONE', *, *, #12023, .T. ) ;
#15073=CARTESIAN_POINT ( 'NONE',  ( 17.58250999373982282, 125.2198453306090045, 5.979920648958140776E-13 ) ) ;
#15074=CARTESIAN_POINT ( 'NONE',  ( 8.608950980928550933, 133.4921716645119432, 14.72901497434506091 ) ) ;
#15076=PRODUCT_CONTEXT ( 'NONE', #15236, 'mechanical' ) ;
#15077=EDGE_CURVE ( 'NONE', #14256, #11533, #13931, .T. ) ;
#15080=LINE ( 'NONE', #8618, #13899 ) ;
#15081=CARTESIAN_POINT ( 'NONE',  ( 15.97577464858015617, 18.00000000000457234, 12.97048270532338243 ) ) ;
#15083=DIRECTION ( 'NONE',  ( -0.000000000000000000, -0.000000000000000000, -1.000000000000000000 ) ) ;
#15085=DIRECTION ( 'NONE',  ( 0.000000000000000000, 0.000000000000000000, -1.000000000000000000 ) ) ;
#15093=VERTEX_POINT ( 'NONE', #16681 ) ;
#15101=DIRECTION ( 'NONE',  ( -1.000000000000000000, -0.000000000000000000, -0.000000000000000000 ) ) ;
#15103=CARTESIAN_POINT ( 'NONE',  ( -5.000000000000004441, 144.1839557653416080, 18.33333333333336057 ) ) ;
#15105=FACE_BOUND ( 'NONE', #17256, .T. ) ;
#15111=FACE_BOUND ( 'NONE', #14579, .T. ) ;
#15112=DIRECTION ( 'NONE',  ( 1.000000000000000000, 0.000000000000000000, 1.445602896647339163E-16 ) ) ;
#15118=LINE ( 'NONE', #2831, #16597 ) ;
#15119=CARTESIAN_POINT ( 'NONE',  ( -25.49999999999998579, 10.00000000000000000, 0.000000000000000000 ) ) ;
#15120=AXIS2_PLACEMENT_3D ( 'NONE', #12843, #3289, #12767 ) ;
#15122=CARTESIAN_POINT ( 'NONE',  ( 14.93242934743710393, 30.00000000000000000, 13.00000000000000178 ) ) ;
#15124=CARTESIAN_POINT ( 'NONE',  ( -77.32133379281293628, 200.8588467739806163, 15.30956876290917457 ) ) ;
#15125=VECTOR ( 'NONE', #3244, 1000.000000000000000 ) ;
#15130=DIRECTION ( 'NONE',  ( 0.000000000000000000, 0.000000000000000000, -1.000000000000000000 ) ) ;
#15131=VERTEX_POINT ( 'NONE', #560 ) ;
#15133=CARTESIAN_POINT ( 'NONE',  ( -15.98664213571245440, 31.85373729401663212, 11.16351695777366082 ) ) ;
#15139=AXIS2_PLACEMENT_3D ( 'NONE', #11341, #10182, #14182 ) ;
#15143=LINE ( 'NONE', #3022, #6840 ) ;
#15144=DIRECTION ( 'NONE',  ( 1.000000000000000000, 0.000000000000000000, 0.000000000000000000 ) ) ;
#15145=B_SPLINE_CURVE_WITH_KNOTS ( 'NONE', 3,
 ( #5937, #13989, #4431, #6899, #12656, #8496, #15312, #10970, #8305, #1592, #16652, #11061, #266, #5672, #4519, #3185, #9725, #9552, #13640, #8402, #1852, #172, #15122 ),
 .UNSPECIFIED., .F., .F.,
 ( 4, 2, 2, 2, 2, 2, 2, 2, 1, 2, 2, 4 ),
 ( 0.000000000000000000, 0.001562580732212274365, 0.002343871098318411547, 0.003125161464424548730, 0.004687742196636830901, 0.006250322928849113939, 0.007812903661061397845, 0.008594194027167533292, 0.009375484393273670475, 0.01015677475937980939, 0.01093806512548594484, 0.01250064585769823135 ),
 .UNSPECIFIED. ) ;
#15146=DIRECTION ( 'NONE',  ( -0.000000000000000000, -0.000000000000000000, -1.000000000000000000 ) ) ;
#15148=VERTEX_POINT ( 'NONE', #5775 ) ;
#15151=ORIENTED_EDGE ( 'NONE', *, *, #7317, .T. ) ;
#15154=DIRECTION ( 'NONE',  ( -0.000000000000000000, -0.000000000000000000, -1.000000000000000000 ) ) ;
#15155=CIRCLE ( 'NONE', #12334, 12.00000000000000000 ) ;
#15161=B_SPLINE_CURVE_WITH_KNOTS ( 'NONE', 3,
 ( #7108, #8523, #14015, #1885 ),
 .UNSPECIFIED., .F., .F.,
 ( 4, 4 ),
 ( 0.000000000000000000, 0.003888888888888887042 ),
 .UNSPECIFIED. ) ;
#15162=CARTESIAN_POINT ( 'NONE',  ( 17.52204077229825785, 125.6458339596819798, 5.684362142990314837 ) ) ;
#15166=ORIENTED_EDGE ( 'NONE', *, *, #6963, .T. ) ;
#15173=DIRECTION ( 'NONE',  ( 1.000000000000000000, 0.000000000000000000, 0.000000000000000000 ) ) ;
#15175=CARTESIAN_POINT ( 'NONE',  ( 20.11141720500412333, 18.00000000000000000, 24.32074799214299077 ) ) ;
#15181=CARTESIAN_POINT ( 'NONE',  ( 32.99999999999998579, 9.999999999999998224, 35.00200000000000244 ) ) ;
#15184=AXIS2_PLACEMENT_3D ( 'NONE', #12655, #7252, #7345 ) ;
#15185=ORIENTED_EDGE ( 'NONE', *, *, #17287, .F. ) ;
#15188=ORIENTED_EDGE ( 'NONE', *, *, #847, .T. ) ;
#15191=CARTESIAN_POINT ( 'NONE',  ( -45.00000000000000000, 120.0000000000000142, 0.000000000000000000 ) ) ;
#15199=EDGE_LOOP ( 'NONE', ( #15541, #6652, #12242, #11781 ) ) ;
#15202=DIRECTION ( 'NONE',  ( -1.000000000000000000, -0.000000000000000000, -0.000000000000000000 ) ) ;
#15208=EDGE_LOOP ( 'NONE', ( #8546, #2995, #11956, #11691, #3525, #710 ) ) ;
#15212=ORIENTED_EDGE ( 'NONE', *, *, #7428, .T. ) ;
#15213=SURFACE_SIDE_STYLE ('',( #4510 ) ) ;
#15216=CARTESIAN_POINT ( 'NONE',  ( 25.00000000000000000, 196.6227766016838245, 21.54065922853802562 ) ) ;
#15217=DIRECTION ( 'NONE',  ( 0.000000000000000000, -1.000000000000000000, 0.000000000000000000 ) ) ;
#15219=LINE ( 'NONE', #12392, #11555 ) ;
#15223=ORIENTED_EDGE ( 'NONE', *, *, #5054, .F. ) ;
#15224=EDGE_CURVE ( 'NONE', #15613, #8372, #7610, .T. ) ;
#15228=DIRECTION ( 'NONE',  ( -0.000000000000000000, -0.000000000000000000, -1.000000000000000000 ) ) ;
#15231=ORIENTED_EDGE ( 'NONE', *, *, #9584, .T. ) ;
#15234=AXIS2_PLACEMENT_3D ( 'NONE', #14424, #13090, #8916 ) ;
#15236=APPLICATION_CONTEXT ( 'automotive_design' ) ;
#15243=DIRECTION ( 'NONE',  ( 0.000000000000000000, 0.000000000000000000, 1.000000000000000000 ) ) ;
#15249=AXIS2_PLACEMENT_3D ( 'NONE', #12946, #7448, #8860 ) ;
#15254=EDGE_LOOP ( 'NONE', ( #11552, #6106, #708, #7133 ) ) ;
#15258=CARTESIAN_POINT ( 'NONE',  ( 15.14881438696876614, 128.6905335926829252, 10.89137921944116449 ) ) ;
#15260=CIRCLE ( 'NONE', #4247, 2.500000000000002220 ) ;
#15261=ORIENTED_EDGE ( 'NONE', *, *, #16199, .T. ) ;
#15262=CARTESIAN_POINT ( 'NONE',  ( -38.00000000000000000, 18.00000000000000355, 0.000000000000000000 ) ) ;
#15263=CIRCLE ( 'NONE', #5664, 12.00000000000001421 ) ;
#15265=CARTESIAN_POINT ( 'NONE',  ( -84.91986817799207188, 195.5664139939901531, 22.72185355927995687 ) ) ;
#15268=CARTESIAN_POINT ( 'NONE',  ( 14.93242934743710570, 30.00000000000000000, 13.00000000000000178 ) ) ;
#15269=CYLINDRICAL_SURFACE ( 'NONE', #13695, 2.500000000000000444 ) ;
#15274=DIRECTION ( 'NONE',  ( 0.000000000000000000, 0.000000000000000000, 1.000000000000000000 ) ) ;
#15275=DIRECTION ( 'NONE',  ( 1.000000000000000000, 0.000000000000000000, 0.000000000000000000 ) ) ;
#15282=CARTESIAN_POINT ( 'NONE',  ( 13.85534145189780197, 143.5014890223674229, 17.26861023069377410 ) ) ;
#15283=EDGE_LOOP ( 'NONE', ( #12537, #9140, #10108, #17275 ) ) ;
#15285=ORIENTED_EDGE ( 'NONE', *, *, #1704, .T. ) ;
#15287=LINE ( 'NONE', #15364, #5959 ) ;
#15289=CARTESIAN_POINT ( 'NONE',  ( -45.00000000000000000, 134.2062027339443944, 15.00000000000000000 ) ) ;
#15291=DIRECTION ( 'NONE',  ( 0.8660254037844378194, -0.5000000000000015543, -0.000000000000000000 ) ) ;
#15293=ORIENTED_EDGE ( 'NONE', *, *, #8283, .T. ) ;
#15294=CARTESIAN_POINT ( 'NONE',  ( 26.35862406984590578, 143.1840127716920961, 16.74578779913501947 ) ) ;
#15300=LINE ( 'NONE', #3351, #7630 ) ;
#15305=CARTESIAN_POINT ( 'NONE',  ( 18.97648483518030815, 140.5725221174451747, 16.15500418213391143 ) ) ;
#15309=CARTESIAN_POINT ( 'NONE',  ( 196.0000000000000000, 183.6227766016837961, 5.571800142134975431 ) ) ;
#15310=PLANE ( 'NONE',  #9528 ) ;
#15312=CARTESIAN_POINT ( 'NONE',  ( 22.42614717998981178, 29.85190128815754917, 7.820018500632365033 ) ) ;
#15315=ORIENTED_EDGE ( 'NONE', *, *, #9995, .T. ) ;
#15319=ORIENTED_EDGE ( 'NONE', *, *, #1992, .T. ) ;
#15320=DIRECTION ( 'NONE',  ( 1.000000000000000000, 0.000000000000000000, 0.000000000000000000 ) ) ;
#15321=LINE ( 'NONE', #16915, #3847 ) ;
#15325=EDGE_CURVE ( 'NONE', #16876, #13316, #8949, .T. ) ;
#15327=EDGE_CURVE ( 'NONE', #11165, #14513, #16933, .T. ) ;
#15330=LINE ( 'NONE', #16756, #4580 ) ;
#15332=CARTESIAN_POINT ( 'NONE',  ( 40.00000000000000711, 146.6227766016838245, 0.000000000000000000 ) ) ;
#15333=ORIENTED_EDGE ( 'NONE', *, *, #3215, .F. ) ;
#15337=CARTESIAN_POINT ( 'NONE',  ( 27.50000000000000355, 196.6227766016838245, 0.000000000000000000 ) ) ;
#15338=ORIENTED_EDGE ( 'NONE', *, *, #8571, .F. ) ;
#15339=DIRECTION ( 'NONE',  ( -1.000000000000000000, 0.000000000000000000, 0.000000000000000000 ) ) ;
#15341=CARTESIAN_POINT ( 'NONE',  ( 16.26529498815395769, 136.8354558863973409, 4.782531348471837696 ) ) ;
#15343=ORIENTED_EDGE ( 'NONE', *, *, #9138, .F. ) ;
#15348=CARTESIAN_POINT ( 'NONE',  ( 21.36708699129047773, 18.00000000000000000, 23.94811280430834088 ) ) ;
#15350=DIRECTION ( 'NONE',  ( 0.000000000000000000, 1.000000000000000000, 0.000000000000000000 ) ) ;
#15351=ORIENTED_EDGE ( 'NONE', *, *, #4352, .T. ) ;
#15355=CARTESIAN_POINT ( 'NONE',  ( 49.99999999999998579, 175.6227766016838530, 19.42820660268601074 ) ) ;
#15358=ORIENTED_EDGE ( 'NONE', *, *, #9046, .T. ) ;
#15361=EDGE_CURVE ( 'NONE', #2062, #5181, #1408, .T. ) ;
#15364=CARTESIAN_POINT ( 'NONE',  ( -48.00000000000000000, 206.6227766016838245, -2.143131898507868248E-15 ) ) ;
#15365=CARTESIAN_POINT ( 'NONE',  ( -48.00000000000000000, 191.6227766016837961, -1.224646799147353454E-15 ) ) ;
#15367=CARTESIAN_POINT ( 'NONE',  ( 17.00000000000000000, 206.6227766016838245, -2.143131898507868248E-15 ) ) ;
#15371=CARTESIAN_POINT ( 'NONE',  ( -100.0000000000000000, 100.0000000000000142, 0.000000000000000000 ) ) ;
#15372=DIRECTION ( 'NONE',  ( 1.000000000000000000, 0.000000000000000000, 0.000000000000000000 ) ) ;
#15375=CARTESIAN_POINT ( 'NONE',  ( -34.99999999999999289, 122.0000000000000000, 0.000000000000000000 ) ) ;
#15376=ORIENTED_EDGE ( 'NONE', *, *, #823, .T. ) ;
#15377=EDGE_CURVE ( 'NONE', #1349, #3629, #7890, .T. ) ;
#15390=CARTESIAN_POINT ( 'NONE',  ( 34.93420767853316988, 18.00000000000000355, 0.000000000000000000 ) ) ;
#15391=LINE ( 'NONE', #3620, #12973 ) ;
#15400=ORIENTED_EDGE ( 'NONE', *, *, #15450, .T. ) ;
#15401=LINE ( 'NONE', #541, #12066 ) ;
#15407=CARTESIAN_POINT ( 'NONE',  ( -25.15885279626527549, 18.00000000000000355, 15.13659797665870066 ) ) ;
#15409=AXIS2_PLACEMENT_3D ( 'NONE', #2705, #13510, #1380 ) ;
#15412=CARTESIAN_POINT ( 'NONE',  ( -7.970809231268917827, 17.99999999998357936, 12.80353734461080428 ) ) ;
#15413=LINE ( 'NONE', #16578, #4097 ) ;
#15417=B_SPLINE_CURVE_WITH_KNOTS ( 'NONE', 3,
 ( #1018, #5098, #15981, #14482, #16974, #2265, #861, #10492, #6168, #2347, #3866, #11563, #17049, #10397, #3687, #7740, #6253, #2436, #14399, #15897 ),
 .UNSPECIFIED., .F., .F.,
 ( 4, 2, 2, 2, 2, 2, 2, 2, 2, 4 ),
 ( 0.000000000000000000, 0.002318945972243265704, 0.003478418958364892268, 0.004637891944486519265, 0.006956837916729771525, 0.009275783888973026386, 0.01159472986121627865, 0.01391367583345953091, 0.01623262180570278490, 0.01855156777794603890 ),
 .UNSPECIFIED. ) ;
#15419=CARTESIAN_POINT ( 'NONE',  ( -45.00000000000000000, 130.0000000000000000, 15.00000000000000000 ) ) ;
#15421=EDGE_CURVE ( 'NONE', #16427, #570, #15527, .T. ) ;
#15423=EDGE_CURVE ( 'NONE', #1164, #12878, #6201, .T. ) ;
#15424=AXIS2_PLACEMENT_3D ( 'NONE', #2713, #8100, #1024 ) ;
#15425=EDGE_CURVE ( 'NONE', #5381, #16355, #5330, .T. ) ;
#15428=VECTOR ( 'NONE', #16078, 1000.000000000000000 ) ;
#15429=CARTESIAN_POINT ( 'NONE',  ( 24.80291332262510196, 19.99999999999999645, 7.298429162487363620 ) ) ;
#15430=CARTESIAN_POINT ( 'NONE',  ( 21.38051303314620810, 139.8000659834381736, 14.57605648433057510 ) ) ;
#15434=CARTESIAN_POINT ( 'NONE',  ( 27.44407568426044008, 126.9014170516880284, 4.999999999999997335 ) ) ;
#15435=CARTESIAN_POINT ( 'NONE',  ( -76.58855154275256893, 192.9634543217044893, 25.17141653689332870 ) ) ;
#15436=LINE ( 'NONE', #8448, #9922 ) ;
#15437=DIRECTION ( 'NONE',  ( 0.000000000000000000, 0.000000000000000000, 1.000000000000000000 ) ) ;
#15443=EDGE_LOOP ( 'NONE', ( #12336, #15838 ) ) ;
#15446=ADVANCED_FACE ( 'NONE', ( #13299 ), #16138, .T. ) ;
#15448=EDGE_CURVE ( 'NONE', #3421, #10977, #262, .T. ) ;
#15449=ORIENTED_EDGE ( 'NONE', *, *, #13843, .F. ) ;
#15450=EDGE_CURVE ( 'NONE', #2358, #5417, #14965, .T. ) ;
#15453=CIRCLE ( 'NONE', #8383, 2.500000000000002220 ) ;
#15456=VECTOR ( 'NONE', #6088, 1000.000000000000000 ) ;
#15457=EDGE_LOOP ( 'NONE', ( #10232, #15808, #11886, #3041 ) ) ;
#15459=CARTESIAN_POINT ( 'NONE',  ( 12.04170873690402566, 130.2202688438208327, 11.06482237631273868 ) ) ;
#15463=ORIENTED_EDGE ( 'NONE', *, *, #16073, .F. ) ;
#15472=DIRECTION ( 'NONE',  ( -0.000000000000000000, -0.000000000000000000, -1.000000000000000000 ) ) ;
#15476=AXIS2_PLACEMENT_3D ( 'NONE', #13801, #3984, #9440 ) ;
#15477=LINE ( 'NONE', #3521, #6798 ) ;
#15478=AXIS2_PLACEMENT_3D ( 'NONE', #4206, #3948, #1462 ) ;
#15483=FACE_OUTER_BOUND ( 'NONE', #1303, .T. ) ;
#15488=ORIENTED_EDGE ( 'NONE', *, *, #1766, .T. ) ;
#15492=ORIENTED_EDGE ( 'NONE', *, *, #2506, .F. ) ;
#15499=DIRECTION ( 'NONE',  ( -1.000000000000000000, 0.000000000000000000, 0.000000000000000000 ) ) ;
#15505=CARTESIAN_POINT ( 'NONE',  ( -11.06002279671335131, 17.99999999999999645, 10.55202560282026703 ) ) ;
#15509=CARTESIAN_POINT ( 'NONE',  ( 25.00000000000000000, 196.6227766016838245, 0.000000000000000000 ) ) ;
#15510=ORIENTED_EDGE ( 'NONE', *, *, #15803, .T. ) ;
#15511=CARTESIAN_POINT ( 'NONE',  ( -15.00000000000002487, 120.0000000000000284, 4.999999999999999112 ) ) ;
#15513=TOROIDAL_SURFACE ( 'NONE', #1956, 25.00000000000000000, 10.00000000000000000 ) ;
#15514=ORIENTED_EDGE ( 'NONE', *, *, #34, .T. ) ;
#15517=ADVANCED_FACE ( 'NONE', ( #16222 ), #14877, .F. ) ;
#15518=CARTESIAN_POINT ( 'NONE',  ( 19.96520957614361436, 19.99999999999771916, 13.72477420846906249 ) ) ;
#15519=CARTESIAN_POINT ( 'NONE',  ( 25.87766738269516509, 137.9415577646583415, 9.529521052671011461 ) ) ;
#15521=CARTESIAN_POINT ( 'NONE',  ( 6.134011831684053284, 142.5209969267753820, 19.44444444444444642 ) ) ;
#15524=DIRECTION ( 'NONE',  ( 0.000000000000000000, 0.000000000000000000, 1.000000000000000000 ) ) ;
#15527=CIRCLE ( 'NONE', #558, 2.500000000000000000 ) ;
#15528=CARTESIAN_POINT ( 'NONE',  ( 25.00000000000000711, 146.6227766016838245, 0.000000000000000000 ) ) ;
#15530=ORIENTED_EDGE ( 'NONE', *, *, #13394, .F. ) ;
#15541=ORIENTED_EDGE ( 'NONE', *, *, #13216, .T. ) ;
#15544=VERTEX_POINT ( 'NONE', #8313 ) ;
#15547=CARTESIAN_POINT ( 'NONE',  ( 7.438682885632053932, 133.7774783946093464, 12.91151668396746111 ) ) ;
#15549=EDGE_CURVE ( 'NONE', #5356, #14594, #13829, .T. ) ;
#15550=EDGE_CURVE ( 'NONE', #15970, #14256, #4436, .T. ) ;
#15551=CARTESIAN_POINT ( 'NONE',  ( 27.44407568426047561, 138.8271129316868837, 3.666666666666728247 ) ) ;
#15554=LINE ( 'NONE', #3430, #11800 ) ;
#15559=CIRCLE ( 'NONE', #7919, 2.500000000000002220 ) ;
#15567=DIRECTION ( 'NONE',  ( -1.000000000000000000, 0.000000000000000000, 0.000000000000000000 ) ) ;
#15572=DIRECTION ( 'NONE',  ( -0.000000000000000000, 0.000000000000000000, 1.000000000000000000 ) ) ;
#15578=VERTEX_POINT ( 'NONE', #5756 ) ;
#15581=VERTEX_POINT ( 'NONE', #9731 ) ;
#15582=CARTESIAN_POINT ( 'NONE',  ( -50.00000000000000000, 154.3022685259950038, 9.999999999999900524 ) ) ;
#15585=EDGE_CURVE ( 'NONE', #16986, #3929, #10034, .T. ) ;
#15586=LINE ( 'NONE', #7439, #15819 ) ;
#15587=ADVANCED_FACE ( 'NONE', ( #11239 ), #7089, .F. ) ;
#15590=DIRECTION ( 'NONE',  ( 1.000000000000000000, -0.000000000000000000, -0.000000000000000000 ) ) ;
#15591=CARTESIAN_POINT ( 'NONE',  ( -16.01409026037699945, 32.68451876144969503, 7.109513113881434698 ) ) ;
#15593=DIRECTION ( 'NONE',  ( 5.638339401448894059E-16, -0.000000000000000000, -1.000000000000000000 ) ) ;
#15594=ORIENTED_EDGE ( 'NONE', *, *, #5128, .F. ) ;
#15597=DIRECTION ( 'NONE',  ( -0.8571673013836870192, 0.000000000000000000, -0.5150380737757234151 ) ) ;
#15600=DIRECTION ( 'NONE',  ( 0.000000000000000000, -0.8660254037844413721, 0.4999999999999953371 ) ) ;
#15601=CARTESIAN_POINT ( 'NONE',  ( 21.08563699167523353, 19.99999999999771561, 13.01331479026599602 ) ) ;
#15602=EDGE_CURVE ( 'NONE', #805, #4320, #4956, .T. ) ;
#15604=CARTESIAN_POINT ( 'NONE',  ( 35.00000000000000000, 196.6227766016838245, 0.000000000000000000 ) ) ;
#15613=VERTEX_POINT ( 'NONE', #12543 ) ;
#15621=EDGE_CURVE ( 'NONE', #17286, #216, #1287, .T. ) ;
#15624=ORIENTED_EDGE ( 'NONE', *, *, #13824, .T. ) ;
#15626=FACE_OUTER_BOUND ( 'NONE', #10546, .T. ) ;
#15628=CARTESIAN_POINT ( 'NONE',  ( 22.56235622051156042, 18.00000000000113332, 7.873592366086867855 ) ) ;
#15629=FACE_OUTER_BOUND ( 'NONE', #5923, .T. ) ;
#15630=ORIENTED_EDGE ( 'NONE', *, *, #2170, .T. ) ;
#15631=CARTESIAN_POINT ( 'NONE',  ( 49.99999999999998579, 187.6227766016837961, 15.00000337241049486 ) ) ;
#15633=DIRECTION ( 'NONE',  ( -1.000000000000000000, 0.000000000000000000, 0.000000000000000000 ) ) ;
#15635=DIRECTION ( 'NONE',  ( -0.000000000000000000, -0.000000000000000000, -1.000000000000000000 ) ) ;
#15636=B_SPLINE_CURVE_WITH_KNOTS ( 'NONE', 3,
 ( #5734, #6078, #13893, #2015, #3076, #9967, #8558, #7232, #16798, #11122, #682, #16540, #3167, #6000, #12729, #1752, #8477, #10146, #11211, #8648, #13969, #5911, #14061, #14227, #11390, #4665, #16721, #412, #4411, #11304, #15294, #4587, #11472, #1925, #16883, #7147, #7323, #4759 ),
 .UNSPECIFIED., .F., .F.,
 ( 4, 2, 2, 2, 2, 2, 2, 2, 2, 2, 2, 2, 2, 2, 2, 2, 2, 2, 4 ),
 ( 0.01870878530979003598, 0.02011211734399855761, 0.02151544937820707576, 0.02432211344662417798, 0.02572544548083270655, 0.02712877751504123164, 0.02783044353214549071, 0.02853210954924975326, 0.02923377556635403315, 0.02993544158345830958, 0.03063710760056260335, 0.03133877361766689018, 0.03204043963477118395, 0.03274210565187547078, 0.03414543768608402363, 0.03554876972029256954, 0.03695210175450111545, 0.03835543378870967524, 0.04116209785712676705 ),
 .UNSPECIFIED. ) ;
#15637=CARTESIAN_POINT ( 'NONE',  ( 32.06052738088115461, 201.1823876344234066, 14.67159435888867769 ) ) ;
#15642=CARTESIAN_POINT ( 'NONE',  ( -725.0000000000000000, 19.99999999999995737, 0.000000000000000000 ) ) ;
#15646=CARTESIAN_POINT ( 'NONE',  ( -68.00000000000000000, 191.6227766016837961, -1.224646799147353454E-15 ) ) ;
#15649=CARTESIAN_POINT ( 'NONE',  ( 49.99999999999998579, 175.6227766016838530, 21.92820660268601074 ) ) ;
#15650=CYLINDRICAL_SURFACE ( 'NONE', #14389, 2.499999999999998668 ) ;
#15653=ORIENTED_EDGE ( 'NONE', *, *, #687, .T. ) ;
#15656=VECTOR ( 'NONE', #660, 1000.000000000000000 ) ;
#15657=CARTESIAN_POINT ( 'NONE',  ( 40.00000000000000711, 171.6227766016838245, 0.000000000000000000 ) ) ;
#15658=ADVANCED_FACE ( 'NONE', ( #3073 ), #4662, .F. ) ;
#15659=ORIENTED_EDGE ( 'NONE', *, *, #78, .T. ) ;
#15660=DIRECTION ( 'NONE',  ( -1.000000000000000000, 0.000000000000000000, 0.000000000000000000 ) ) ;
#15666=CONICAL_SURFACE ( 'NONE', #2675, 2.499999999999998668, 1.029744260000002187 ) ;
#15668=CARTESIAN_POINT ( 'NONE',  ( -12.76199592490470636, 17.99999999999999645, 6.193401609026034649 ) ) ;
#15675=EDGE_CURVE ( 'NONE', #5614, #1074, #3341, .T. ) ;
#15680=AXIS2_PLACEMENT_3D ( 'NONE', #16837, #8519, #11256 ) ;
#15681=CARTESIAN_POINT ( 'NONE',  ( 25.06493225413665016, 20.00000000000000000, 5.000000000000004441 ) ) ;
#15692=EDGE_LOOP ( 'NONE', ( #1316, #15315, #2613, #2776 ) ) ;
#15696=CARTESIAN_POINT ( 'NONE',  ( -24.99999999999999645, 120.0000000000000284, 0.000000000000000000 ) ) ;
#15697=AXIS2_PLACEMENT_3D ( 'NONE', #7838, #14570, #13249 ) ;
#15704=EDGE_CURVE ( 'NONE', #8580, #9736, #7321, .T. ) ;
#15706=VERTEX_POINT ( 'NONE', #12727 ) ;
#15713=CARTESIAN_POINT ( 'NONE',  ( 15.60228996708985072, 124.9392590763940518, 1.450155947765682260E-14 ) ) ;
#15715=CARTESIAN_POINT ( 'NONE',  ( 48.00000000000000711, 167.6227766016838530, 8.071800142134975431 ) ) ;
#15718=CARTESIAN_POINT ( 'NONE',  ( 24.67988836892261872, 29.87169161469932277, 7.267893787782148785 ) ) ;
#15719=EDGE_LOOP ( 'NONE', ( #3722, #13131, #15071 ) ) ;
#15722=AXIS2_PLACEMENT_3D ( 'NONE', #15965, #5253, #7818 ) ;
#15724=CARTESIAN_POINT ( 'NONE',  ( 29.74080762574056180, 201.6174249061529338, 13.75941557453018582 ) ) ;
#15730=LINE ( 'NONE', #2455, #10457 ) ;
#15732=CARTESIAN_POINT ( 'NONE',  ( -26.89314795393037372, 18.00000000000000000, 11.55702759004479852 ) ) ;
#15740=CARTESIAN_POINT ( 'NONE',  ( -68.00000000000000000, 171.6227766016838245, 0.000000000000000000 ) ) ;
#15746=VERTEX_POINT ( 'NONE', #16881 ) ;
#15749=CONICAL_SURFACE ( 'NONE', #6984, 35.00000000000000000, 0.5235987755983005920 ) ;
#15753=VECTOR ( 'NONE', #15994, 1000.000000000000000 ) ;
#15756=CARTESIAN_POINT ( 'NONE',  ( 49.99999999999998579, 191.6227766016837677, 3.071800142134975431 ) ) ;
#15758=CYLINDRICAL_SURFACE ( 'NONE', #10645, 2.500000000000000444 ) ;
#15760=CARTESIAN_POINT ( 'NONE',  ( -8.542481054582452771, 30.38359229753140767, 12.94984885967198451 ) ) ;
#15761=ADVANCED_FACE ( 'NONE', ( #12982 ), #12316, .T. ) ;
#15762=EDGE_CURVE ( 'NONE', #9957, #5131, #10144, .T. ) ;
#15764=AXIS2_PLACEMENT_3D ( 'NONE', #10695, #2643, #10784 ) ;
#15765=PLANE ( 'NONE',  #12566 ) ;
#15770=DIRECTION ( 'NONE',  ( -1.000000000000000000, 0.000000000000000000, 0.000000000000000000 ) ) ;
#15771=EDGE_LOOP ( 'NONE', ( #14283, #4177 ) ) ;
#15774=VERTEX_POINT ( 'NONE', #14302 ) ;
#15775=CARTESIAN_POINT ( 'NONE',  ( 34.26588824652853305, 20.00000000000000355, 10.16858984204336736 ) ) ;
#15777=CARTESIAN_POINT ( 'NONE',  ( 21.54097706593338302, 29.91227807600463606, 12.53500607440986236 ) ) ;
#15783=DIRECTION ( 'NONE',  ( 0.000000000000000000, 0.000000000000000000, -1.000000000000000000 ) ) ;
#15786=CARTESIAN_POINT ( 'NONE',  ( -7.379000772445021283, 30.00000000000000000, 25.00000000000000000 ) ) ;
#15787=AXIS2_PLACEMENT_3D ( 'NONE', #5866, #11258, #15062 ) ;
#15788=ORIENTED_EDGE ( 'NONE', *, *, #15602, .F. ) ;
#15797=AXIS2_PLACEMENT_3D ( 'NONE', #16493, #368, #8692 ) ;
#15798=ORIENTED_EDGE ( 'NONE', *, *, #1075, .T. ) ;
#15800=EDGE_CURVE ( 'NONE', #12169, #16221, #11906, .T. ) ;
#15801=AXIS2_PLACEMENT_3D ( 'NONE', #15511, #3126, #5965 ) ;
#15802=FACE_OUTER_BOUND ( 'NONE', #9496, .T. ) ;
#15803=EDGE_CURVE ( 'NONE', #4609, #12155, #7481, .T. ) ;
#15807=CARTESIAN_POINT ( 'NONE',  ( -84.92227909014668796, 147.6670862717896000, 22.70911985051488102 ) ) ;
#15808=ORIENTED_EDGE ( 'NONE', *, *, #1704, .F. ) ;
#15813=CARTESIAN_POINT ( 'NONE',  ( 22.87571619445694182, 29.89494019521412582, 11.08657135066705379 ) ) ;
#15815=DIRECTION ( 'NONE',  ( 1.000000000000000000, 0.000000000000000000, 0.000000000000000000 ) ) ;
#15818=VECTOR ( 'NONE', #14359, 1000.000000000000000 ) ;
#15819=VECTOR ( 'NONE', #3378, 1000.000000000000000 ) ;
#15820=CARTESIAN_POINT ( 'NONE',  ( 26.35433596972580972, 200.0568792608333410, 16.75365501014454139 ) ) ;
#15824=DIRECTION ( 'NONE',  ( -0.000000000000000000, -0.000000000000000000, 1.000000000000000000 ) ) ;
#15829=CIRCLE ( 'NONE', #7623, 12.00000000000000000 ) ;
#15832=DIRECTION ( 'NONE',  ( -1.000000000000000000, 0.000000000000000000, 0.000000000000000000 ) ) ;
#15835=ADVANCED_FACE ( 'NONE', ( #15629 ), #769, .F. ) ;
#15837=EDGE_CURVE ( 'NONE', #7694, #13835, #8643, .T. ) ;
#15838=ORIENTED_EDGE ( 'NONE', *, *, #2005, .F. ) ;
#15841=VERTEX_POINT ( 'NONE', #3506 ) ;
#15843=AXIS2_PLACEMENT_3D ( 'NONE', #10235, #14401, #15633 ) ;
#15845=EDGE_LOOP ( 'NONE', ( #7359, #8179, #3880, #16588 ) ) ;
#15854=LINE ( 'NONE', #12039, #10072 ) ;
#15855=CARTESIAN_POINT ( 'NONE',  ( -2.428612866367531510E-15, 18.00000000000000355, 28.00000000000000711 ) ) ;
#15856=DIRECTION ( 'NONE',  ( -0.000000000000000000, -0.000000000000000000, -1.000000000000000000 ) ) ;
#15857=CARTESIAN_POINT ( 'NONE',  ( -20.86241502029199424, 18.00000000000000000, 20.14618526197082460 ) ) ;
#15858=CARTESIAN_POINT ( 'NONE',  ( 35.00000000000000711, 146.6227766016838245, 0.000000000000000000 ) ) ;
#15859=ORIENTED_EDGE ( 'NONE', *, *, #11264, .T. ) ;
#15860=CARTESIAN_POINT ( 'NONE',  ( 22.99999999999997868, 9.999999999999998224, 0.000000000000000000 ) ) ;
#15864=B_SPLINE_CURVE_WITH_KNOTS ( 'NONE', 3,
 ( #6464, #10713, #14783, #14867, #14517, #8138, #2384, #13549, #6368, #11765, #7780, #11857, #17267, #5141, #1765, #14955, #13637, #5576, #3092, #2914, #9635, #4164, #4334, #11133, #13715, #8572, #9721, #16471, #6824, #16292, #1502, #7162, #8302, #9546, #347, #16553, #3182, #8493, #5486, #15216 ),
 .UNSPECIFIED., .F., .F.,
 ( 4, 2, 2, 2, 2, 2, 2, 2, 2, 2, 2, 2, 2, 2, 2, 2, 2, 2, 2, 4 ),
 ( 0.02243093923957175523, 0.02359459467514160580, 0.02475825011071145984, 0.02592190554628131041, 0.02708556098185116445, 0.02766738869963611402, 0.02824921641742106360, 0.02941287185299096621, 0.03057652728856086882, 0.03115835500634580799, 0.03174018272413074715, 0.03232201044191568284, 0.03290383815970061854, 0.03348566587748556117, 0.03406749359527049686, 0.03523114903084040295, 0.03639480446641030209, 0.03755845990198020123, 0.03872211533755010038, 0.04104942620868985009 ),
 .UNSPECIFIED. ) ;
#15867=CARTESIAN_POINT ( 'NONE',  ( 12.31199832339570577, 129.9194306174879046, 10.85217099066659685 ) ) ;
#15870=EDGE_CURVE ( 'NONE', #15148, #5896, #12721, .T. ) ;
#15872=ADVANCED_FACE ( 'NONE', ( #6945, #14916, #2795 ), #9342, .F. ) ;
#15880=ORIENTED_EDGE ( 'NONE', *, *, #17473, .T. ) ;
#15882=DIRECTION ( 'NONE',  ( 2.312964634635742464E-16, 0.000000000000000000, -1.000000000000000000 ) ) ;
#15889=ORIENTED_EDGE ( 'NONE', *, *, #4304, .T. ) ;
#15891=CARTESIAN_POINT ( 'NONE',  ( -15.96992528024541613, 32.67167891243749978, 7.259156848219323166 ) ) ;
#15894=CARTESIAN_POINT ( 'NONE',  ( 32.90650748920769075, 18.00000000000000000, 13.87185692903161360 ) ) ;
#15897=CARTESIAN_POINT ( 'NONE',  ( 16.17028938446068764, 143.0439382767918346, 16.49999999999050360 ) ) ;
#15900=CARTESIAN_POINT ( 'NONE',  ( 31.20890926080315353, 18.00000000000000000, 16.64259892333393154 ) ) ;
#15903=CARTESIAN_POINT ( 'NONE',  ( 17.00000000000000000, 171.6227766016838245, 0.000000000000000000 ) ) ;
#15904=EDGE_CURVE ( 'NONE', #13139, #14743, #6789, .T. ) ;
#15909=ORIENTED_EDGE ( 'NONE', *, *, #15377, .F. ) ;
#15911=CARTESIAN_POINT ( 'NONE',  ( -80.48051234362822015, 141.6406938050144504, 13.78697217532817554 ) ) ;
#15915=VERTEX_POINT ( 'NONE', #12087 ) ;
#15916=CARTESIAN_POINT ( 'NONE',  ( -23.00000000000002842, 120.0000000000000284, 4.999999999999999112 ) ) ;
#15918=CARTESIAN_POINT ( 'NONE',  ( 48.00000000000000711, 183.6227766016837961, 3.071800142134975431 ) ) ;
#15919=DIRECTION ( 'NONE',  ( -0.8660254037844378194, -0.5000000000000015543, -0.000000000000000000 ) ) ;
#15923=LINE ( 'NONE', #5305, #16335 ) ;
#15924=VERTEX_POINT ( 'NONE', #132 ) ;
#15928=ORIENTED_EDGE ( 'NONE', *, *, #14888, .T. ) ;
#15929=CARTESIAN_POINT ( 'NONE',  ( 22.93524650466158832, 29.84210526315789380, 0.000000000000000000 ) ) ;
#15930=CARTESIAN_POINT ( 'NONE',  ( -38.00000000000000000, 18.00000000000000355, 0.000000000000000000 ) ) ;
#15931=EDGE_CURVE ( 'NONE', #12504, #11533, #1547, .T. ) ;
#15934=DIRECTION ( 'NONE',  ( 0.000000000000000000, 0.000000000000000000, 1.000000000000000000 ) ) ;
#15936=( BOUNDED_SURFACE ( )  B_SPLINE_SURFACE ( 3, 2, ( 
 ( #9673, #4294, #8264 ),
 ( #9497, #8177, #12079 ),
 ( #14908, #9591, #5358 ),
 ( #11010, #17389, #15074 ),
 ( #1537, #10754, #2788 ),
 ( #1373, #16337, #16070 ),
 ( #4037, #13502, #5526 ),
 ( #6777, #12174, #44 ),
 ( #6860, #13592, #124 ),
 ( #12249, #10913, #2951 ),
 ( #6935, #12339, #8345 ),
 ( #13760, #1634, #7032 ),
 ( #7118, #12517, #12780 ),
 ( #12433, #16686, #381 ),
 ( #10017, #3399, #14200 ),
 ( #15430, #13858, #650 ),
 ( #13940, #9854, #1802 ),
 ( #11176, #7197, #12599 ),
 ( #14024, #5874, #15258 ),
 ( #465, #12691, #567 ),
 ( #7286, #4375, #4467 ),
 ( #15519, #11268, #8530 ),
 ( #4555, #9941, #3133 ),
 ( #8794, #8613, #1724 ),
 ( #8707, #16506, #2061 ),
 ( #9764, #15341, #3306 ),
 ( #14116, #5971, #1890 ),
 ( #3216, #306, #5707 ),
 ( #11360, #11092, #15162 ),
 ( #6047, #16770, #3040 ) ),
 .UNSPECIFIED., .F., .F., .F. ) 
 B_SPLINE_SURFACE_WITH_KNOTS ( ( 4, 2, 2, 2, 2, 2, 2, 2, 2, 2, 2, 2, 2, 2, 4 ),
 ( 3, 3 ),
 ( 0.01165250788892074896, 0.01579789672993320987, 0.01787059115043944033, 0.01890693836069255729, 0.01994328557094567078, 0.02408867441195813169, 0.02616136883246436215, 0.02823406325297059261, 0.03030675767347682306, 0.03237945209398305352, 0.03652484093499551443, 0.03859753535550174142, 0.03963388256575485491, 0.04067022977600797534, 0.04481561861702043625 ),
 ( 0.000000000000000000, 1.000000000000000000 ),
 .UNSPECIFIED. ) 
 GEOMETRIC_REPRESENTATION_ITEM ( )  RATIONAL_B_SPLINE_SURFACE ( (
 ( 1.000000000000000000, 0.8819171036881967574, 1.000000000000000000),
 ( 1.000000000000000000, 0.8793942645247267986, 1.000000000000000000),
 ( 1.000000000000000000, 0.8749458316895478704, 1.000000000000000000),
 ( 1.000000000000000000, 0.8656814021268812720, 1.000000000000000000),
 ( 1.000000000000000000, 0.8621600075896179716, 1.000000000000000000),
 ( 1.000000000000000000, 0.8562492930711324002, 1.000000000000000000),
 ( 1.000000000000000000, 0.8541736901085718037, 1.000000000000000000),
 ( 1.000000000000000000, 0.8498659178639272893, 1.000000000000000000),
 ( 1.000000000000000000, 0.8476283308601378907, 1.000000000000000000),
 ( 1.000000000000000000, 0.8360458749412158497, 1.000000000000000000),
 ( 1.000000000000000000, 0.8255221978280062878, 1.000000000000000000),
 ( 1.000000000000000000, 0.8082270345002190437, 1.000000000000000000),
 ( 1.000000000000000000, 0.8022128341710524913, 1.000000000000000000),
 ( 1.000000000000000000, 0.7899684886178014454, 1.000000000000000000),
 ( 1.000000000000000000, 0.7837128169315926707, 1.000000000000000000),
 ( 1.000000000000000000, 0.7710263478624882483, 1.000000000000000000),
 ( 1.000000000000000000, 0.7645952338536526893, 1.000000000000000000),
 ( 1.000000000000000000, 0.7516613202048504361, 1.000000000000000000),
 ( 1.000000000000000000, 0.7451386183437513910, 1.000000000000000000),
 ( 1.000000000000000000, 0.7257808243684673588, 1.000000000000000000),
 ( 1.000000000000000000, 0.7133953845776390690, 1.000000000000000000),
 ( 1.000000000000000000, 0.6965170042221164870, 1.000000000000000000),
 ( 1.000000000000000000, 0.6911767420095684678, 1.000000000000000000),
 ( 1.000000000000000000, 0.6837405640632492343, 1.000000000000000000),
 ( 1.000000000000000000, 0.6813577907325653049, 1.000000000000000000),
 ( 1.000000000000000000, 0.6768117804539316440, 1.000000000000000000),
 ( 1.000000000000000000, 0.6746439590912862716, 1.000000000000000000),
 ( 1.000000000000000000, 0.6645663254999056857, 1.000000000000000000),
 ( 1.000000000000000000, 0.6588263891901358082, 1.000000000000000000),
 ( 1.000000000000000000, 0.6558243695371221982, 1.000000000000000000) ) ) 
 REPRESENTATION_ITEM ( '' )  SURFACE ( )  );
#15937=CARTESIAN_POINT ( 'NONE',  ( 37.99999999999999289, 20.00000000000000000, 0.000000000000000000 ) ) ;
#15939=CARTESIAN_POINT ( 'NONE',  ( -80.00000000000002842, 146.6227766016838245, 10.00000000000000178 ) ) ;
#15941=DIRECTION ( 'NONE',  ( -0.000000000000000000, 0.000000000000000000, -1.000000000000000000 ) ) ;
#15944=ORIENTED_EDGE ( 'NONE', *, *, #4463, .F. ) ;
#15949=CARTESIAN_POINT ( 'NONE',  ( 13.35668486245713282, 128.6964509245273405, 9.918424562684259982 ) ) ;
#15951=CARTESIAN_POINT ( 'NONE',  ( 17.20299680575017831, 29.96951112202298262, 14.74034971990100296 ) ) ;
#15954=AXIS2_PLACEMENT_3D ( 'NONE', #12337, #16504, #9761 ) ;
#15960=PLANE ( 'NONE',  #1645 ) ;
#15962=EDGE_CURVE ( 'NONE', #6874, #15013, #4371, .T. ) ;
#15965=CARTESIAN_POINT ( 'NONE',  ( -80.00000000000001421, 196.6227766016838245, 10.00000000000000178 ) ) ;
#15970=VERTEX_POINT ( 'NONE', #10682 ) ;
#15977=CARTESIAN_POINT ( 'NONE',  ( -82.50000000000001421, 196.6227766016838245, 10.00000000000000178 ) ) ;
#15978=CARTESIAN_POINT ( 'NONE',  ( 29.97257796258590901, 18.00000000000000000, 18.20111186907413980 ) ) ;
#15981=CARTESIAN_POINT ( 'NONE',  ( 27.32038637416026816, 139.0270950805171424, 5.204462201318943215 ) ) ;
#15985=CARTESIAN_POINT ( 'NONE',  ( 6.134011831684053284, 134.2062027339443944, 15.00000000000000000 ) ) ;
#15988=CARTESIAN_POINT ( 'NONE',  ( 20.22393135579957502, 29.92951751662230109, 13.49252536210626197 ) ) ;
#15990=FACE_BOUND ( 'NONE', #12943, .T. ) ;
#15991=CARTESIAN_POINT ( 'NONE',  ( 26.56193816801034302, 200.2660383695261999, 16.39286986631262266 ) ) ;
#15994=DIRECTION ( 'NONE',  ( 1.000000000000000000, 0.000000000000000000, 0.000000000000000000 ) ) ;
#15996=VERTEX_POINT ( 'NONE', #7193 ) ;
#16002=AXIS2_PLACEMENT_3D ( 'NONE', #2945, #15154, #16332 ) ;
#16003=AXIS2_PLACEMENT_3D ( 'NONE', #11882, #2146, #2505 ) ;
#16005=CARTESIAN_POINT ( 'NONE',  ( 15.78015847649388448, 143.0439382767918346, 16.49999999999050360 ) ) ;
#16012=ORIENTED_EDGE ( 'NONE', *, *, #8189, .T. ) ;
#16014=CARTESIAN_POINT ( 'NONE',  ( 0.000000000000000000, 2.000000000000000000, 0.000000000000000000 ) ) ;
#16016=VERTEX_POINT ( 'NONE', #210 ) ;
#16023=DIRECTION ( 'NONE',  ( 0.000000000000000000, 8.410780489584519664E-16, -1.000000000000000000 ) ) ;
#16026=ADVANCED_FACE ( 'NONE', ( #8438 ), #8342, .T. ) ;
#16031=DIRECTION ( 'NONE',  ( -0.000000000000000000, -0.000000000000000000, 1.000000000000000000 ) ) ;
#16032=DIRECTION ( 'NONE',  ( -1.000000000000000000, -0.000000000000000000, -0.000000000000000000 ) ) ;
#16035=LINE ( 'NONE', #6147, #16147 ) ;
#16041=AXIS2_PLACEMENT_3D ( 'NONE', #12105, #2890, #8109 ) ;
#16042=EDGE_CURVE ( 'NONE', #14845, #15774, #8016, .T. ) ;
#16045=CARTESIAN_POINT ( 'NONE',  ( -8.091731396663927711, 30.16237610810089365, 15.00000000000000355 ) ) ;
#16046=CARTESIAN_POINT ( 'NONE',  ( 27.42233521511133887, 138.9393305618597481, 4.670371664028303726 ) ) ;
#16048=ORIENTED_EDGE ( 'NONE', *, *, #12848, .F. ) ;
#16051=AXIS2_PLACEMENT_3D ( 'NONE', #15740, #13175, #17248 ) ;
#16059=CARTESIAN_POINT ( 'NONE',  ( 34.23838175495608027, 149.2800176679284903, 24.28646496670947741 ) ) ;
#16069=( GEOMETRIC_REPRESENTATION_CONTEXT ( 3 ) GLOBAL_UNCERTAINTY_ASSIGNED_CONTEXT ( ( #5203 ) ) GLOBAL_UNIT_ASSIGNED_CONTEXT ( ( #2996, #16382, #9717 ) ) REPRESENTATION_CONTEXT ( 'NONE', 'WORKASPACE' ) );
#16070=CARTESIAN_POINT ( 'NONE',  ( 9.474973892937489595, 133.0798911729450538, 14.49933486760529355 ) ) ;
#16073=EDGE_CURVE ( 'NONE', #11660, #16675, #13982, .T. ) ;
#16075=CARTESIAN_POINT ( 'NONE',  ( -11.03695849842137910, 30.81357570984703642, 14.42948753805835871 ) ) ;
#16077=LINE ( 'NONE', #5266, #12754 ) ;
#16078=DIRECTION ( 'NONE',  ( -0.000000000000000000, -0.000000000000000000, -1.000000000000000000 ) ) ;
#16080=CIRCLE ( 'NONE', #12689, 2.500000000000000444 ) ;
#16082=ORIENTED_EDGE ( 'NONE', *, *, #5474, .F. ) ;
#16083=PLANE ( 'NONE',  #8143 ) ;
#16087=CARTESIAN_POINT ( 'NONE',  ( 40.00000000000000711, 171.6227766016838245, 0.000000000000000000 ) ) ;
#16088=VERTEX_POINT ( 'NONE', #5284 ) ;
#16090=DIRECTION ( 'NONE',  ( -0.000000000000000000, -0.000000000000000000, -1.000000000000000000 ) ) ;
#16092=CARTESIAN_POINT ( 'NONE',  ( 32.99999999999998579, 9.999999999999998224, 28.00000000000001066 ) ) ;
#16096=AXIS2_PLACEMENT_3D ( 'NONE', #10839, #13866, #7038 ) ;
#16098=EDGE_CURVE ( 'NONE', #5825, #14287, #14536, .T. ) ;
#16104=DIRECTION ( 'NONE',  ( -0.000000000000000000, 0.000000000000000000, -1.000000000000000000 ) ) ;
#16106=CARTESIAN_POINT ( 'NONE',  ( -25.15885279626527193, 20.00000000000000355, 15.13659797665870776 ) ) ;
#16109=VECTOR ( 'NONE', #8213, 1000.000000000000000 ) ;
#16131=CARTESIAN_POINT ( 'NONE',  ( -725.0000000000000000, 19.99999999999995737, 15.00000000000000000 ) ) ;
#16134=ORIENTED_EDGE ( 'NONE', *, *, #3359, .T. ) ;
#16138=PLANE ( 'NONE',  #10438 ) ;
#16139=CIRCLE ( 'NONE', #2842, 2.500000000000002220 ) ;
#16141=ORIENTED_EDGE ( 'NONE', *, *, #15962, .F. ) ;
#16143=CARTESIAN_POINT ( 'NONE',  ( -11.18069906337402664, 30.84474844633047397, 14.38199110044527274 ) ) ;
#16144=CARTESIAN_POINT ( 'NONE',  ( 19.90854668962690255, 142.0789032940274410, 14.70609183182490298 ) ) ;
#16147=VECTOR ( 'NONE', #11542, 1000.000000000000000 ) ;
#16149=VECTOR ( 'NONE', #4726, 1000.000000000000000 ) ;
#16155=CARTESIAN_POINT ( 'NONE',  ( 25.46873702927104333, 148.7415597018667199, 23.77993541092453711 ) ) ;
#16156=ORIENTED_EDGE ( 'NONE', *, *, #14013, .T. ) ;
#16158=CARTESIAN_POINT ( 'NONE',  ( -5.000000000000004441, 142.8100939375178200, 16.63501009223129756 ) ) ;
#16159=VECTOR ( 'NONE', #477, 1000.000000000000000 ) ;
#16161=ORIENTED_EDGE ( 'NONE', *, *, #12092, .T. ) ;
#16164=DIRECTION ( 'NONE',  ( -0.000000000000000000, -0.000000000000000000, -1.000000000000000000 ) ) ;
#16165=EDGE_CURVE ( 'NONE', #5035, #2441, #16811, .T. ) ;
#16166=VERTEX_POINT ( 'NONE', #7627 ) ;
#16172=VECTOR ( 'NONE', #9839, 1000.000000000000000 ) ;
#16173=DIRECTION ( 'NONE',  ( 0.000000000000000000, 0.000000000000000000, -1.000000000000000000 ) ) ;
#16174=CARTESIAN_POINT ( 'NONE',  ( -78.65474156909843373, 151.4423111973152061, 26.11038153352143709 ) ) ;
#16176=DIRECTION ( 'NONE',  ( 0.000000000000000000, -1.000000000000000000, 0.000000000000000000 ) ) ;
#16180=CARTESIAN_POINT ( 'NONE',  ( -95.00000000000000000, 199.3133755249253056, 1.695560166891042033E-15 ) ) ;
#16186=ORIENTED_EDGE ( 'NONE', *, *, #17492, .F. ) ;
#16192=CARTESIAN_POINT ( 'NONE',  ( -19.79962810613638169, 20.00000000000000355, 20.97942696524415851 ) ) ;
#16194=DIRECTION ( 'NONE',  ( -2.312964634635742464E-16, 0.000000000000000000, 1.000000000000000000 ) ) ;
#16196=DIRECTION ( 'NONE',  ( 1.000000000000000000, 0.000000000000000000, 0.000000000000000000 ) ) ;
#16199=EDGE_CURVE ( 'NONE', #16869, #6523, #4683, .T. ) ;
#16200=EDGE_CURVE ( 'NONE', #16488, #2665, #6220, .T. ) ;
#16201=ORIENTED_EDGE ( 'NONE', *, *, #1796, .T. ) ;
#16202=CARTESIAN_POINT ( 'NONE',  ( -5.000000000000000888, 204.6227766016838245, -2.020667218593133100E-15 ) ) ;
#16205=CARTESIAN_POINT ( 'NONE',  ( -27.99999999999998224, 10.00000000000000000, 11.50215154306610188 ) ) ;
#16206=EDGE_LOOP ( 'NONE', ( #3461, #1344, #10432, #9439 ) ) ;
#16207=DIRECTION ( 'NONE',  ( 0.000000000000000000, 0.000000000000000000, -1.000000000000000000 ) ) ;
#16208=DIRECTION ( 'NONE',  ( 1.000000000000000000, 0.000000000000000000, 0.000000000000000000 ) ) ;
#16209=CARTESIAN_POINT ( 'NONE',  ( 27.48361012698968864, 138.6227766016838245, 1.063447695028166570E-14 ) ) ;
#16218=DIRECTION ( 'NONE',  ( 0.000000000000000000, -0.8660254037844413721, 0.4999999999999953371 ) ) ;
#16220=ADVANCED_FACE ( 'NONE', ( #8863 ), #14113, .F. ) ;
#16221=VERTEX_POINT ( 'NONE', #14720 ) ;
#16222=FACE_OUTER_BOUND ( 'NONE', #10537, .T. ) ;
#16223=DIRECTION ( 'NONE',  ( -1.000000000000000000, -0.000000000000000000, -0.000000000000000000 ) ) ;
#16224=ORIENTED_EDGE ( 'NONE', *, *, #3991, .T. ) ;
#16226=CARTESIAN_POINT ( 'NONE',  ( 15.07980489400154056, 126.2730657262978724, 7.274180996386617970 ) ) ;
#16228=CARTESIAN_POINT ( 'NONE',  ( 20.42763382733002686, 19.99999999999999645, 24.23318166603087676 ) ) ;
#16230=FACE_OUTER_BOUND ( 'NONE', #10418, .T. ) ;
#16232=CARTESIAN_POINT ( 'NONE',  ( 48.00000000000000711, 183.6227766016837961, 5.571800142134975431 ) ) ;
#16236=CARTESIAN_POINT ( 'NONE',  ( 25.92568854015031121, 149.5391923287904490, 24.52402115671403493 ) ) ;
#16242=ORIENTED_EDGE ( 'NONE', *, *, #17492, .T. ) ;
#16245=LINE ( 'NONE', #10661, #16630 ) ;
#16246=ORIENTED_EDGE ( 'NONE', *, *, #4473, .T. ) ;
#16249=CARTESIAN_POINT ( 'NONE',  ( -96.00000000000001421, 141.6227766016838245, -5.510910596163088767E-15 ) ) ;
#16250=DIRECTION ( 'NONE',  ( 1.000000000000000000, 0.000000000000000000, 0.000000000000000000 ) ) ;
#16252=CARTESIAN_POINT ( 'NONE',  ( -79.22094317722377355, 151.5769270156786206, 26.21405625665653005 ) ) ;
#16255=ORIENTED_EDGE ( 'NONE', *, *, #17387, .T. ) ;
#16257=DIRECTION ( 'NONE',  ( -0.000000000000000000, -0.000000000000000000, -1.000000000000000000 ) ) ;
#16262=EDGE_CURVE ( 'NONE', #17055, #5035, #10542, .T. ) ;
#16266=VECTOR ( 'NONE', #5954, 1000.000000000000000 ) ;
#16268=DIRECTION ( 'NONE',  ( 0.000000000000000000, 1.734723475976807094E-15, 1.000000000000000000 ) ) ;
#16270=DIRECTION ( 'NONE',  ( -1.000000000000000000, -0.000000000000000000, -0.000000000000000000 ) ) ;
#16273=VERTEX_POINT ( 'NONE', #7895 ) ;
#16274=CARTESIAN_POINT ( 'NONE',  ( -48.00000000000000000, 154.3022685259950038, 9.999999999999900524 ) ) ;
#16277=LINE ( 'NONE', #9536, #10602 ) ;
#16291=CIRCLE ( 'NONE', #15722, 2.500000000000002220 ) ;
#16292=CARTESIAN_POINT ( 'NONE',  ( 27.43384137083016583, 192.3153571870206235, 25.70724251753713929 ) ) ;
#16300=VERTEX_POINT ( 'NONE', #14529 ) ;
#16315=ADVANCED_FACE ( 'NONE', ( #5236 ), #9152, .F. ) ;
#16316=ADVANCED_FACE ( 'NONE', ( #8242 ), #100, .T. ) ;
#16323=VECTOR ( 'NONE', #9007, 1000.000000000000000 ) ;
#16328=CARTESIAN_POINT ( 'NONE',  ( 27.42854581659407742, 150.9146311475675759, 25.69413650784048642 ) ) ;
#16332=DIRECTION ( 'NONE',  ( -1.000000000000000000, 0.000000000000000000, 0.000000000000000000 ) ) ;
#16333=EDGE_LOOP ( 'NONE', ( #9408, #1085, #14795, #11257 ) ) ;
#16335=VECTOR ( 'NONE', #1051, 1000.000000000000000 ) ;
#16337=CARTESIAN_POINT ( 'NONE',  ( 10.45945364060320237, 139.0001874602887995, 13.88305366436938115 ) ) ;
#16342=DIRECTION ( 'NONE',  ( -1.156482317317868274E-16, 1.000000000000000000, 0.000000000000000000 ) ) ;
#16347=ORIENTED_EDGE ( 'NONE', *, *, #16638, .F. ) ;
#16349=CIRCLE ( 'NONE', #5021, 27.69059892324149175 ) ;
#16350=CARTESIAN_POINT ( 'NONE',  ( 13.59940502541562246, 130.1762661646492063, 12.36432683418100353 ) ) ;
#16353=CARTESIAN_POINT ( 'NONE',  ( -100.0000000000000000, 171.6227766016838245, 27.69059892324149175 ) ) ;
#16355=VERTEX_POINT ( 'NONE', #12403 ) ;
#16358=ORIENTED_EDGE ( 'NONE', *, *, #14204, .F. ) ;
#16361=EDGE_LOOP ( 'NONE', ( #8251, #14904 ) ) ;
#16364=CARTESIAN_POINT ( 'NONE',  ( -91.33974596215564645, 171.6227766016838245, 0.000000000000000000 ) ) ;
#16381=EDGE_LOOP ( 'NONE', ( #438, #1182, #6674, #15058 ) ) ;
#16382=( NAMED_UNIT ( * ) PLANE_ANGLE_UNIT ( ) SI_UNIT ( $, .RADIAN. ) );
#16385=CIRCLE ( 'NONE', #15234, 2.500000000000000000 ) ;
#16386=ADVANCED_FACE ( 'NONE', ( #11670 ), #9992, .F. ) ;
#16390=VECTOR ( 'NONE', #8327, 1000.000000000000000 ) ;
#16391=DIRECTION ( 'NONE',  ( -1.000000000000000000, -0.000000000000000000, -0.000000000000000000 ) ) ;
#16397=CARTESIAN_POINT ( 'NONE',  ( -3.000000000000000888, 154.3022685259950038, 9.999999999999900524 ) ) ;
#16402=ADVANCED_FACE ( 'NONE', ( #892 ), #2118, .T. ) ;
#16404=CARTESIAN_POINT ( 'NONE',  ( -17.89548297089572060, 32.23709896788771090, 7.636891392351368602 ) ) ;
#16410=DIRECTION ( 'NONE',  ( -1.000000000000000000, 0.000000000000000000, 0.000000000000000000 ) ) ;
#16414=DIRECTION ( 'NONE',  ( 0.000000000000000000, -0.4999999999999952816, -0.8660254037844413721 ) ) ;
#16415=ORIENTED_EDGE ( 'NONE', *, *, #5030, .T. ) ;
#16416=PLANE ( 'NONE',  #11705 ) ;
#16423=SHAPE_REPRESENTATION ( 'Left Housing Shell', ( #3583 ), #11517 ) ;
#16425=DIRECTION ( 'NONE',  ( 0.000000000000000000, 0.000000000000000000, -1.000000000000000000 ) ) ;
#16427=VERTEX_POINT ( 'NONE', #11340 ) ;
#16432=DIRECTION ( 'NONE',  ( -1.000000000000000000, 0.000000000000000000, 0.000000000000000000 ) ) ;
#16434=ORIENTED_EDGE ( 'NONE', *, *, #2970, .T. ) ;
#16440=CARTESIAN_POINT ( 'NONE',  ( 18.97220464449422295, 17.99999999999999645, 12.00279687791388383 ) ) ;
#16444=CARTESIAN_POINT ( 'NONE',  ( -20.85786437626906675, 124.1421356237309652, 14.99999999999998401 ) ) ;
#16449=EDGE_CURVE ( 'NONE', #11802, #10963, #15401, .T. ) ;
#16452=DIRECTION ( 'NONE',  ( -1.000000000000000000, -0.000000000000000000, -0.000000000000000000 ) ) ;
#16460=FACE_BOUND ( 'NONE', #6859, .T. ) ;
#16462=DIRECTION ( 'NONE',  ( -1.000000000000000000, -0.000000000000000000, -0.000000000000000000 ) ) ;
#16464=ORIENTED_EDGE ( 'NONE', *, *, #10670, .T. ) ;
#16467=ORIENTED_EDGE ( 'NONE', *, *, #61, .F. ) ;
#16469=CARTESIAN_POINT ( 'NONE',  ( -50.00000000000000000, 143.0439382767972631, 16.49999999999984013 ) ) ;
#16471=CARTESIAN_POINT ( 'NONE',  ( 28.10980041848796063, 191.9899036175949618, 25.96511099662696509 ) ) ;
#16476=ADVANCED_FACE ( 'NONE', ( #12836 ), #7516, .T. ) ;
#16488=VERTEX_POINT ( 'NONE', #15582 ) ;
#16493=CARTESIAN_POINT ( 'NONE',  ( 17.00000000000000000, 171.6227766016838245, 0.000000000000000000 ) ) ;
#16495=LINE ( 'NONE', #13845, #2679 ) ;
#16496=ORIENTED_EDGE ( 'NONE', *, *, #14562, .F. ) ;
#16497=DIRECTION ( 'NONE',  ( 1.000000000000000000, 0.000000000000000000, 0.000000000000000000 ) ) ;
#16498=ORIENTED_EDGE ( 'NONE', *, *, #16889, .T. ) ;
#16501=DIRECTION ( 'NONE',  ( 1.000000000000000000, 0.000000000000000000, 0.000000000000000000 ) ) ;
#16504=DIRECTION ( 'NONE',  ( 0.000000000000000000, 0.000000000000000000, 1.000000000000000000 ) ) ;
#16505=DIRECTION ( 'NONE',  ( -1.000000000000000000, 0.000000000000000000, 0.000000000000000000 ) ) ;
#16506=CARTESIAN_POINT ( 'NONE',  ( 16.30283403932918063, 136.8379281265527254, 4.993081733805470712 ) ) ;
#16507=EDGE_LOOP ( 'NONE', ( #13402, #12623, #7605, #7618, #7512 ) ) ;
#16512=CARTESIAN_POINT ( 'NONE',  ( 27.44407568426044008, 138.8271129316868837, 3.666666666666658081 ) ) ;
#16513=ADVANCED_FACE ( 'NONE', ( #3459 ), #3542, .F. ) ;
#16514=CARTESIAN_POINT ( 'NONE',  ( 18.26135686777217160, 17.99999999999999289, 12.35203162874035065 ) ) ;
#16519=DIRECTION ( 'NONE',  ( 0.000000000000000000, 0.000000000000000000, -1.000000000000000000 ) ) ;
#16520=DIRECTION ( 'NONE',  ( -1.000000000000000000, -6.938893903907228378E-16, 0.000000000000000000 ) ) ;
#16521=AXIS2_PLACEMENT_3D ( 'NONE', #15309, #3183, #6989 ) ;
#16524=CARTESIAN_POINT ( 'NONE',  ( 6.714477151836450552, 134.0780154003031726, 13.00000000000000000 ) ) ;
#16525=ORIENTED_EDGE ( 'NONE', *, *, #8981, .F. ) ;
#16526=CARTESIAN_POINT ( 'NONE',  ( 27.50000000000001066, 146.6227766016838245, 10.00000000000000178 ) ) ;
#16536=AXIS2_PLACEMENT_3D ( 'NONE', #13648, #9564, #7173 ) ;
#16537=EDGE_CURVE ( 'NONE', #570, #14499, #7771, .T. ) ;
#16540=CARTESIAN_POINT ( 'NONE',  ( 32.22389789336222776, 142.1412512070565413, 14.82809033015228195 ) ) ;
#16541=CARTESIAN_POINT ( 'NONE',  ( -43.00000000000000000, 134.2062027339443944, 25.00000000000000000 ) ) ;
#16542=DIRECTION ( 'NONE',  ( -1.000000000000000000, -0.000000000000000000, -0.000000000000000000 ) ) ;
#16547=DIRECTION ( 'NONE',  ( -1.000000000000000000, 0.000000000000000000, 0.000000000000000000 ) ) ;
#16548=ORIENTED_EDGE ( 'NONE', *, *, #10692, .F. ) ;
#16549=( LENGTH_UNIT ( ) NAMED_UNIT ( * ) SI_UNIT ( .MILLI., .METRE. ) );
#16553=CARTESIAN_POINT ( 'NONE',  ( 25.46628596442746684, 194.4926179048318602, 23.79294127240566681 ) ) ;
#16554=LINE ( 'NONE', #16813, #9728 ) ;
#16558=( GEOMETRIC_REPRESENTATION_CONTEXT ( 3 ) GLOBAL_UNCERTAINTY_ASSIGNED_CONTEXT ( ( #1007 ) ) GLOBAL_UNIT_ASSIGNED_CONTEXT ( ( #2734, #74, #17337 ) ) REPRESENTATION_CONTEXT ( 'NONE', 'WORKASPACE' ) );
#16559=CARTESIAN_POINT ( 'NONE',  ( -78.47686795807116766, 201.3896308033655487, 14.24607874381215744 ) ) ;
#16563=DIRECTION ( 'NONE',  ( 0.000000000000000000, 1.000000000000000000, 0.000000000000000000 ) ) ;
#16569=ORIENTED_EDGE ( 'NONE', *, *, #11007, .T. ) ;
#16570=EDGE_CURVE ( 'NONE', #6571, #9979, #1230, .T. ) ;
#16576=CARTESIAN_POINT ( 'NONE',  ( 49.99999999999998579, 167.6227766016838530, 8.071800142134975431 ) ) ;
#16577=DIRECTION ( 'NONE',  ( 0.000000000000000000, 0.8660254037844413721, -0.4999999999999952816 ) ) ;
#16578=CARTESIAN_POINT ( 'NONE',  ( -40.00000000000000000, 20.00000000000000000, 30.00000000000000355 ) ) ;
#16580=CARTESIAN_POINT ( 'NONE',  ( -80.00000000000001421, 196.6227766016838245, 10.00000000000000178 ) ) ;
#16584=VECTOR ( 'NONE', #14214, 1000.000000000000000 ) ;
#16588=ORIENTED_EDGE ( 'NONE', *, *, #11334, .F. ) ;
#16597=VECTOR ( 'NONE', #12293, 1000.000000000000000 ) ;
#16599=DIRECTION ( 'NONE',  ( -1.000000000000000000, 0.000000000000000000, 0.000000000000000000 ) ) ;
#16601=CARTESIAN_POINT ( 'NONE',  ( -84.24272906227606939, 193.9598103731634353, 24.29383909379281192 ) ) ;
#16602=DIRECTION ( 'NONE',  ( 1.000000000000000000, 0.000000000000000000, 0.000000000000000000 ) ) ;
#16603=CARTESIAN_POINT ( 'NONE',  ( 15.97392895077415531, 29.97895215653467815, 12.94942366938410139 ) ) ;
#16604=FACE_OUTER_BOUND ( 'NONE', #14665, .T. ) ;
#16611=CARTESIAN_POINT ( 'NONE',  ( -95.00000000000000000, 171.6227766016838245, 0.000000000000000000 ) ) ;
#16612=AXIS2_PLACEMENT_3D ( 'NONE', #10606, #13096, #13181 ) ;
#16614=CIRCLE ( 'NONE', #8957, 2.499999999999998668 ) ;
#16615=ORIENTED_EDGE ( 'NONE', *, *, #1993, .F. ) ;
#16618=CARTESIAN_POINT ( 'NONE',  ( 6.134011831684059501, 144.1839557653415795, 18.33333333333333215 ) ) ;
#16619=ADVANCED_FACE ( 'NONE', ( #4244 ), #9629, .F. ) ;
#16625=CARTESIAN_POINT ( 'NONE',  ( -725.0000000000000000, 30.00000000000000000, 25.00000000000000000 ) ) ;
#16630=VECTOR ( 'NONE', #13407, 1000.000000000000000 ) ;
#16633=DIRECTION ( 'NONE',  ( 0.000000000000000000, 0.000000000000000000, -1.000000000000000000 ) ) ;
#16635=LINE ( 'NONE', #13897, #13456 ) ;
#16637=DIRECTION ( 'NONE',  ( -1.000000000000000000, 0.000000000000000000, 0.000000000000000000 ) ) ;
#16638=EDGE_CURVE ( 'NONE', #1130, #16300, #10651, .T. ) ;
#16639=ADVANCED_FACE ( 'NONE', ( #9540, #8391, #9714, #14945, #12288, #15111, #2907, #5401, #5742, #6980, #7074, #2993, #255, #13540 ), #5657, .F. ) ;
#16647=CARTESIAN_POINT ( 'NONE',  ( 21.93446201513734550, 139.6105936900751203, 14.17700481206107455 ) ) ;
#16648=CARTESIAN_POINT ( 'NONE',  ( 48.00000000000000711, 175.6227766016838245, 8.071800142134975431 ) ) ;
#16651=CARTESIAN_POINT ( 'NONE',  ( -15.00000000000002132, 90.00000000000000000, 4.999999999999999112 ) ) ;
#16652=CARTESIAN_POINT ( 'NONE',  ( 20.96141083122825322, 29.88026331201747254, 10.28670731940101923 ) ) ;
#16654=CARTESIAN_POINT ( 'NONE',  ( -74.99999999999998579, 197.2379877313572081, 20.82664773619437071 ) ) ;
#16657=ORIENTED_EDGE ( 'NONE', *, *, #6923, .T. ) ;
#16658=ORIENTED_EDGE ( 'NONE', *, *, #3571, .T. ) ;
#16662=CARTESIAN_POINT ( 'NONE',  ( -26.90043998676167192, 19.99999999999999645, 11.53672424425260878 ) ) ;
#16664=AXIS2_PLACEMENT_3D ( 'NONE', #7424, #10251, #12826 ) ;
#16665=ORIENTED_EDGE ( 'NONE', *, *, #7160, .F. ) ;
#16666=AXIS2_PLACEMENT_3D ( 'NONE', #2801, #1554, #17504 ) ;
#16668=CIRCLE ( 'NONE', #12978, 2.499999999999998668 ) ;
#16669=CARTESIAN_POINT ( 'NONE',  ( -27.98221281347037959, 18.00000000000000711, 5.670874406215274277 ) ) ;
#16671=LINE ( 'NONE', #9838, #2122 ) ;
#16674=DIRECTION ( 'NONE',  ( -0.000000000000000000, -0.000000000000000000, -1.000000000000000000 ) ) ;
#16675=VERTEX_POINT ( 'NONE', #10960 ) ;
#16677=VECTOR ( 'NONE', #4760, 1000.000000000000000 ) ;
#16678=VECTOR ( 'NONE', #6835, 1000.000000000000000 ) ;
#16681=CARTESIAN_POINT ( 'NONE',  ( -5.000000000000000888, 154.3022685259950038, 9.999999999999900524 ) ) ;
#16686=CARTESIAN_POINT ( 'NONE',  ( 14.69130379018311316, 137.7259585328908713, 10.44822943247861602 ) ) ;
#16688=ORIENTED_EDGE ( 'NONE', *, *, #3062, .T. ) ;
#16693=CARTESIAN_POINT ( 'NONE',  ( 49.99999999999998579, 179.6227766016838245, 12.50000337241049309 ) ) ;
#16694=CARTESIAN_POINT ( 'NONE',  ( 16.61976933981454962, 29.96600215813370838, 12.82127072618890118 ) ) ;
#16701=FACE_OUTER_BOUND ( 'NONE', #15692, .T. ) ;
#16704=AXIS2_PLACEMENT_3D ( 'NONE', #10310, #941, #5011 ) ;
#16709=CARTESIAN_POINT ( 'NONE',  ( 0.000000000000000000, 18.00000000000000355, 0.000000000000000000 ) ) ;
#16710=ORIENTED_EDGE ( 'NONE', *, *, #15377, .T. ) ;
#16712=DIRECTION ( 'NONE',  ( 0.000000000000000000, 0.000000000000000000, -1.000000000000000000 ) ) ;
#16713=EDGE_CURVE ( 'NONE', #14743, #9236, #12741, .T. ) ;
#16714=ORIENTED_EDGE ( 'NONE', *, *, #8565, .T. ) ;
#16715=CARTESIAN_POINT ( 'NONE',  ( -38.00000000000000000, 20.00000000000000000, 0.000000000000000000 ) ) ;
#16716=CYLINDRICAL_SURFACE ( 'NONE', #3265, 12.00000000000000000 ) ;
#16720=VERTEX_POINT ( 'NONE', #517 ) ;
#16721=CARTESIAN_POINT ( 'NONE',  ( 27.76496263192228042, 142.1468147500166594, 14.83914868552980160 ) ) ;
#16728=VERTEX_POINT ( 'NONE', #12907 ) ;
#16731=CARTESIAN_POINT ( 'NONE',  ( -16.30611068361787019, 32.76923076923078781, 15.00000000000000000 ) ) ;
#16748=ORIENTED_EDGE ( 'NONE', *, *, #7458, .F. ) ;
#16756=CARTESIAN_POINT ( 'NONE',  ( -90.80384757729339640, 204.6227766016838245, 0.000000000000000000 ) ) ;
#16760=ADVANCED_FACE ( 'NONE', ( #11315 ), #6977, .F. ) ;
#16768=CARTESIAN_POINT ( 'NONE',  ( 34.42405209918207731, 19.99999999999999289, 9.535225002503356251 ) ) ;
#16770=CARTESIAN_POINT ( 'NONE',  ( 15.93460003626540100, 136.8193095811535045, 3.708327557688629650 ) ) ;
#16774=ADVANCED_FACE ( 'NONE', ( #783 ), #8831, .F. ) ;
#16775=CYLINDRICAL_SURFACE ( 'NONE', #9784, 20.00000000000000355 ) ;
#16776=CARTESIAN_POINT ( 'NONE',  ( -75.34838324441767554, 194.7673412502506096, 23.52603474534219430 ) ) ;
#16778=DIRECTION ( 'NONE',  ( 0.000000000000000000, 0.000000000000000000, 1.000000000000000000 ) ) ;
#16780=ORIENTED_EDGE ( 'NONE', *, *, #6112, .F. ) ;
#16784=LINE ( 'NONE', #4649, #5348 ) ;
#16786=ORIENTED_EDGE ( 'NONE', *, *, #7458, .T. ) ;
#16787=ORIENTED_EDGE ( 'NONE', *, *, #14223, .F. ) ;
#16788=VERTEX_POINT ( 'NONE', #420 ) ;
#16789=CARTESIAN_POINT ( 'NONE',  ( 7.863372401969320968, 140.4786490112420552, 12.74411896114139076 ) ) ;
#16790=EDGE_LOOP ( 'NONE', ( #6456, #14265, #3541, #14048 ) ) ;
#16793=EDGE_CURVE ( 'NONE', #10702, #17386, #2166, .T. ) ;
#16794=DIRECTION ( 'NONE',  ( -1.000000000000000000, -0.000000000000000000, -0.000000000000000000 ) ) ;
#16798=CARTESIAN_POINT ( 'NONE',  ( 33.42618164656464330, 142.9679699711796275, 16.37278862731308493 ) ) ;
#16800=FACE_BOUND ( 'NONE', #10735, .T. ) ;
#16801=EDGE_CURVE ( 'NONE', #1199, #13709, #611, .T. ) ;
#16802=DIRECTION ( 'NONE',  ( 1.000000000000000000, 0.000000000000000000, 0.000000000000000000 ) ) ;
#16803=DIRECTION ( 'NONE',  ( -1.156482317317868274E-16, 1.000000000000000000, 0.000000000000000000 ) ) ;
#16808=AXIS2_PLACEMENT_3D ( 'NONE', #748, #5884, #5978 ) ;
#16809=ORIENTED_EDGE ( 'NONE', *, *, #14822, .F. ) ;
#16811=CIRCLE ( 'NONE', #7742, 2.499999999999998668 ) ;
#16813=CARTESIAN_POINT ( 'NONE',  ( -45.00000000000000000, 140.0000000000000000, 15.00000000000000000 ) ) ;
#16814=EDGE_LOOP ( 'NONE', ( #8040, #15788 ) ) ;
#16815=FACE_BOUND ( 'NONE', #6540, .T. ) ;
#16819=AXIS2_PLACEMENT_3D ( 'NONE', #2485, #6288, #7529 ) ;
#16821=AXIS2_PLACEMENT_3D ( 'NONE', #12586, #2939, #12418 ) ;
#16828=ORIENTED_EDGE ( 'NONE', *, *, #5535, .T. ) ;
#16830=CARTESIAN_POINT ( 'NONE',  ( 32.50000000000000711, 146.6227766016838245, 0.000000000000000000 ) ) ;
#16831=AXIS2_PLACEMENT_3D ( 'NONE', #813, #15590, #10351 ) ;
#16833=DIRECTION ( 'NONE',  ( 1.000000000000000000, 0.000000000000000000, 0.000000000000000000 ) ) ;
#16835=CARTESIAN_POINT ( 'NONE',  ( -11.94789857657465681, 17.99999999999885603, 9.192893430571174918 ) ) ;
#16837=CARTESIAN_POINT ( 'NONE',  ( 225.0000000000000000, 89.99999999999997158, 0.000000000000000000 ) ) ;
#16839=DIRECTION ( 'NONE',  ( -0.000000000000000000, -0.000000000000000000, -1.000000000000000000 ) ) ;
#16840=ORIENTED_EDGE ( 'NONE', *, *, #8773, .F. ) ;
#16841=DIRECTION ( 'NONE',  ( -1.000000000000000000, -0.000000000000000000, -0.000000000000000000 ) ) ;
#16844=AXIS2_PLACEMENT_3D ( 'NONE', #8993, #15635, #10152 ) ;
#16845=EDGE_LOOP ( 'NONE', ( #4712, #11871, #13566, #12396, #2252, #9406, #9242, #2766, #2698, #14881, #1818, #17164, #14267, #4804 ) ) ;
#16847=AXIS2_PLACEMENT_3D ( 'NONE', #3130, #16090, #15339 ) ;
#16850=CARTESIAN_POINT ( 'NONE',  ( 20.21654089865888437, 29.92961455958988637, 13.49713695059922891 ) ) ;
#16858=CARTESIAN_POINT ( 'NONE',  ( -82.06570270424580826, 192.0656250386302020, 25.90562197801994060 ) ) ;
#16865=CARTESIAN_POINT ( 'NONE',  ( 27.99999999999998224, 9.999999999999998224, 0.000000000000000000 ) ) ;
#16866=ORIENTED_EDGE ( 'NONE', *, *, #14180, .T. ) ;
#16867=CARTESIAN_POINT ( 'NONE',  ( -91.33974596215563224, 136.6227766016838245, 0.000000000000000000 ) ) ;
#16869=VERTEX_POINT ( 'NONE', #1841 ) ;
#16872=AXIS2_PLACEMENT_3D ( 'NONE', #3727, #5409, #14608 ) ;
#16876=VERTEX_POINT ( 'NONE', #14158 ) ;
#16878=FACE_OUTER_BOUND ( 'NONE', #15208, .T. ) ;
#16879=CARTESIAN_POINT ( 'NONE',  ( 9.186438336152177087, 132.7758989760081931, 12.51111164240594675 ) ) ;
#16881=CARTESIAN_POINT ( 'NONE',  ( 30.49999999999998224, 9.999999999999998224, 0.000000000000000000 ) ) ;
#16883=CARTESIAN_POINT ( 'NONE',  ( 25.40874610515435705, 144.6221806392915141, 18.97834816100454702 ) ) ;
#16886=DIRECTION ( 'NONE',  ( 0.000000000000000000, 0.000000000000000000, 1.000000000000000000 ) ) ;
#16888=LINE ( 'NONE', #4764, #11730 ) ;
#16889=EDGE_CURVE ( 'NONE', #11331, #3796, #7417, .T. ) ;
#16892=ORIENTED_EDGE ( 'NONE', *, *, #2107, .T. ) ;
#16893=CARTESIAN_POINT ( 'NONE',  ( -95.00000000000000000, 143.9321776784423150, -5.086680500673126297E-15 ) ) ;
#16894=VERTEX_POINT ( 'NONE', #17056 ) ;
#16895=AXIS2_PLACEMENT_3D ( 'NONE', #7833, #14305, #1115 ) ;
#16896=CARTESIAN_POINT ( 'NONE',  ( 11.02544963116560517, 142.2295695439714791, 19.00161275228506952 ) ) ;
#16898=EDGE_CURVE ( 'NONE', #9236, #8681, #2549, .T. ) ;
#16903=CARTESIAN_POINT ( 'NONE',  ( 40.00000000000000711, 0.000000000000000000, 0.000000000000000000 ) ) ;
#16905=CARTESIAN_POINT ( 'NONE',  ( -79.54766608249138926, 201.6036812327912457, 13.78933345224466933 ) ) ;
#16915=CARTESIAN_POINT ( 'NONE',  ( 196.0000000000000000, 167.6227766016838530, 3.071800142134975431 ) ) ;
#16922=AXIS2_PLACEMENT_3D ( 'NONE', #1623, #16497, #9751 ) ;
#16924=DIRECTION ( 'NONE',  ( 1.000000000000000000, 0.000000000000000000, 8.673617379884037937E-17 ) ) ;
#16926=CARTESIAN_POINT ( 'NONE',  ( -22.80699178664539772, 18.00000000000000000, 18.33022619056923119 ) ) ;
#16930=CARTESIAN_POINT ( 'NONE',  ( 196.0000000000000000, 163.6227766016838530, 15.00000337241049486 ) ) ;
#16931=EDGE_CURVE ( 'NONE', #12800, #6747, #2276, .T. ) ;
#16932=EDGE_LOOP ( 'NONE', ( #7862, #8319, #11170, #5422, #7536 ) ) ;
#16933=LINE ( 'NONE', #10199, #13849 ) ;
#16941=CARTESIAN_POINT ( 'NONE',  ( 25.06493225369642630, 19.99999999999999645, 5.669446505520304491 ) ) ;
#16944=CARTESIAN_POINT ( 'NONE',  ( -75.00000000000000000, 196.6227766016838245, 21.54065922853802206 ) ) ;
#16946=CIRCLE ( 'NONE', #1406, 20.00000000000000355 ) ;
#16951=CIRCLE ( 'NONE', #2821, 20.00000000000000355 ) ;
#16952=ORIENTED_EDGE ( 'NONE', *, *, #7117, .F. ) ;
#16954=EDGE_CURVE ( 'NONE', #7220, #14384, #5296, .T. ) ;
#16955=EDGE_CURVE ( 'NONE', #15131, #1074, #491, .T. ) ;
#16970=CARTESIAN_POINT ( 'NONE',  ( 15.41470791700940879, 125.6764093509959963, 6.286214449974339757 ) ) ;
#16972=DIRECTION ( 'NONE',  ( 1.000000000000000000, 0.000000000000000000, 0.000000000000000000 ) ) ;
#16974=CARTESIAN_POINT ( 'NONE',  ( 26.92745052348471546, 139.3035600351462904, 6.678622460562388952 ) ) ;
#16980=VECTOR ( 'NONE', #13793, 1000.000000000000000 ) ;
#16982=CARTESIAN_POINT ( 'NONE',  ( 30.09541270076643471, 201.6232707959689208, 13.74664867617480901 ) ) ;
#16983=ORIENTED_EDGE ( 'NONE', *, *, #7428, .F. ) ;
#16986=VERTEX_POINT ( 'NONE', #1659 ) ;
#16992=VERTEX_POINT ( 'NONE', #14930 ) ;
#16999=ORIENTED_EDGE ( 'NONE', *, *, #9944, .T. ) ;
#17004=DIRECTION ( 'NONE',  ( 0.000000000000000000, 0.000000000000000000, -1.000000000000000000 ) ) ;
#17008=ADVANCED_FACE ( 'NONE', ( #63 ), #6986, .F. ) ;
#17009=LINE ( 'NONE', #7697, #8678 ) ;
#17010=CARTESIAN_POINT ( 'NONE',  ( 49.99999999999998579, 167.6227766016838530, 5.571800142134975431 ) ) ;
#17011=CARTESIAN_POINT ( 'NONE',  ( -14.45029498972267668, 32.22448475281832003, 9.930813566224275135 ) ) ;
#17012=FACE_OUTER_BOUND ( 'NONE', #6183, .T. ) ;
#17014=EDGE_LOOP ( 'NONE', ( #1145, #5214, #16255 ) ) ;
#17017=EDGE_CURVE ( 'NONE', #12455, #9911, #2719, .T. ) ;
#17023=CARTESIAN_POINT ( 'NONE',  ( 31.20232444246483894, 19.99999999999999645, 16.65183244246150451 ) ) ;
#17024=EDGE_LOOP ( 'NONE', ( #15488, #11553, #1175, #594 ) ) ;
#17030=ORIENTED_EDGE ( 'NONE', *, *, #10851, .F. ) ;
#17037=ORIENTED_EDGE ( 'NONE', *, *, #250, .F. ) ;
#17040=ORIENTED_EDGE ( 'NONE', *, *, #3787, .F. ) ;
#17046=CARTESIAN_POINT ( 'NONE',  ( 34.93420767853318409, 18.00000000000000000, 5.000000000000010658 ) ) ;
#17048=ORIENTED_EDGE ( 'NONE', *, *, #11403, .F. ) ;
#17049=CARTESIAN_POINT ( 'NONE',  ( 22.64347415271929265, 141.1870565414818941, 12.76399958404563684 ) ) ;
#17051=FACE_OUTER_BOUND ( 'NONE', #14644, .T. ) ;
#17054=CARTESIAN_POINT ( 'NONE',  ( 27.75123839167244810, 201.0919203481101079, 14.85271610579516555 ) ) ;
#17055=VERTEX_POINT ( 'NONE', #16526 ) ;
#17056=CARTESIAN_POINT ( 'NONE',  ( 49.99999999999998579, 155.6227766016839098, 15.00000337241049486 ) ) ;
#17061=CARTESIAN_POINT ( 'NONE',  ( -75.21246548080814875, 145.1525832006840346, 19.71138291685208799 ) ) ;
#17062=EDGE_CURVE ( 'NONE', #11495, #17220, #236, .T. ) ;
#17063=ADVANCED_FACE ( 'NONE', ( #4315 ), #9694, .F. ) ;
#17064=CARTESIAN_POINT ( 'NONE',  ( -16.40540729975244716, 18.00000000000000000, 23.03124090058167184 ) ) ;
#17069=CARTESIAN_POINT ( 'NONE',  ( 15.39006516123636281, 143.0404737187717785, 16.50200026350847793 ) ) ;
#17074=ORIENTED_EDGE ( 'NONE', *, *, #5921, .F. ) ;
#17076=VECTOR ( 'NONE', #10693, 1000.000000000000000 ) ;
#17079=EDGE_CURVE ( 'NONE', #9609, #5427, #5014, .T. ) ;
#17081=CARTESIAN_POINT ( 'NONE',  ( -2.428612866367531510E-15, 2.000000000000000000, 28.00000000000000711 ) ) ;
#17085=VECTOR ( 'NONE', #7274, 1000.000000000000000 ) ;
#17086=DIRECTION ( 'NONE',  ( 0.000000000000000000, 1.000000000000000000, 0.000000000000000000 ) ) ;
#17087=CARTESIAN_POINT ( 'NONE',  ( -7.965954974912850872, 30.19485118722929329, 13.00000000000000178 ) ) ;
#17089=DIRECTION ( 'NONE',  ( -1.000000000000000000, 0.000000000000000000, 0.000000000000000000 ) ) ;
#17091=VERTEX_POINT ( 'NONE', #8468 ) ;
#17095=FACE_OUTER_BOUND ( 'NONE', #15443, .T. ) ;
#17096=ADVANCED_FACE ( 'NONE', ( #6158 ), #5023, .F. ) ;
#17099=CARTESIAN_POINT ( 'NONE',  ( 33.66231827095856488, 20.00000000000000000, 12.04861179558545636 ) ) ;
#17103=CARTESIAN_POINT ( 'NONE',  ( 23.15530394309853435, 20.00000000000112976, 10.88800651875285297 ) ) ;
#17116=DIRECTION ( 'NONE',  ( -1.000000000000000000, 0.000000000000000000, 0.000000000000000000 ) ) ;
#17117=ORIENTED_EDGE ( 'NONE', *, *, #15448, .F. ) ;
#17119=ORIENTED_EDGE ( 'NONE', *, *, #8283, .F. ) ;
#17124=CIRCLE ( 'NONE', #4427, 5.000000000000000888 ) ;
#17125=CARTESIAN_POINT ( 'NONE',  ( -10.05507621332305668, 30.59909908010286372, 14.70163937327580328 ) ) ;
#17127=CARTESIAN_POINT ( 'NONE',  ( 30.00000000000001066, 146.6227766016838245, 10.00000000000000178 ) ) ;
#17128=CARTESIAN_POINT ( 'NONE',  ( 22.81311145407750374, 18.00000000000113687, 7.108351238697862229 ) ) ;
#17130=ORIENTED_EDGE ( 'NONE', *, *, #17079, .F. ) ;
#17131=DIRECTION ( 'NONE',  ( -1.000000000000000000, 0.000000000000000000, 0.000000000000000000 ) ) ;
#17136=FACE_OUTER_BOUND ( 'NONE', #3499, .T. ) ;
#17138=EDGE_CURVE ( 'NONE', #13884, #17055, #673, .T. ) ;
#17140=CARTESIAN_POINT ( 'NONE',  ( 25.40795165748616569, 198.6215000397447739, 18.98099903503497288 ) ) ;
#17142=CARTESIAN_POINT ( 'NONE',  ( 27.99999999999998224, 9.999999999999998224, 0.000000000000000000 ) ) ;
#17143=DIRECTION ( 'NONE',  ( 1.000000000000000000, 0.000000000000000000, 0.000000000000000000 ) ) ;
#17144=ORIENTED_EDGE ( 'NONE', *, *, #13103, .F. ) ;
#17154=LINE ( 'NONE', #1220, #16323 ) ;
#17155=CARTESIAN_POINT ( 'NONE',  ( 13.57836111649853450, 143.5532840108684525, 17.35359164609418059 ) ) ;
#17164=ORIENTED_EDGE ( 'NONE', *, *, #15621, .T. ) ;
#17172=DIRECTION ( 'NONE',  ( 1.000000000000000000, 0.000000000000000000, 0.000000000000000000 ) ) ;
#17175=CARTESIAN_POINT ( 'NONE',  ( -95.00000000000000000, 171.6227766016838245, 30.00000000000000000 ) ) ;
#17176=LINE ( 'NONE', #7879, #2444 ) ;
#17177=DIRECTION ( 'NONE',  ( -1.000000000000000000, 0.000000000000000000, 0.000000000000000000 ) ) ;
#17178=CARTESIAN_POINT ( 'NONE',  ( -12.63209758636676305, 18.00000000000116174, 7.167151760391626603 ) ) ;
#17179=AXIS2_PLACEMENT_3D ( 'NONE', #11647, #7661, #13070 ) ;
#17181=CIRCLE ( 'NONE', #8976, 2.499999999999998668 ) ;
#17182=CARTESIAN_POINT ( 'NONE',  ( 34.93420767853318409, 30.00000000000000000, 5.000000000000010658 ) ) ;
#17184=DIRECTION ( 'NONE',  ( -1.000000000000000000, -0.000000000000000000, -0.000000000000000000 ) ) ;
#17189=CARTESIAN_POINT ( 'NONE',  ( -13.95500183466744382, 31.43484250012364001, 12.98634364776042638 ) ) ;
#17190=CARTESIAN_POINT ( 'NONE',  ( 14.16484689353800697, 138.6662281288708982, 3.797024489650498325 ) ) ;
#17192=CARTESIAN_POINT ( 'NONE',  ( 17.53130567297317910, 19.99999999999999289, 14.69383831151754727 ) ) ;
#17201=CIRCLE ( 'NONE', #16922, 2.500000000000000000 ) ;
#17205=DIRECTION ( 'NONE',  ( 1.000000000000000000, -0.000000000000000000, 0.000000000000000000 ) ) ;
#17208=ORIENTED_EDGE ( 'NONE', *, *, #9328, .T. ) ;
#17209=LINE ( 'NONE', #2521, #5587 ) ;
#17211=ORIENTED_EDGE ( 'NONE', *, *, #10692, .T. ) ;
#17214=DIRECTION ( 'NONE',  ( -0.000000000000000000, -0.000000000000000000, -1.000000000000000000 ) ) ;
#17217=CARTESIAN_POINT ( 'NONE',  ( 21.99569976772868074, 17.99999999999999645, 9.076888812463767664 ) ) ;
#17218=CARTESIAN_POINT ( 'NONE',  ( -84.69896753943838519, 148.3373224442695175, 23.38426449892924452 ) ) ;
#17220=VERTEX_POINT ( 'NONE', #3336 ) ;
#17221=FACE_OUTER_BOUND ( 'NONE', #11510, .T. ) ;
#17224=DIRECTION ( 'NONE',  ( 0.000000000000000000, 0.000000000000000000, -1.000000000000000000 ) ) ;
#17226=ORIENTED_EDGE ( 'NONE', *, *, #13026, .F. ) ;
#17229=EDGE_CURVE ( 'NONE', #15578, #1044, #2475, .T. ) ;
#17234=CARTESIAN_POINT ( 'NONE',  ( 25.11100433194186721, 197.8164829328480607, 20.09296681051159439 ) ) ;
#17240=CARTESIAN_POINT ( 'NONE',  ( -81.54154366038537205, 141.8618947663538279, 14.25856086977511339 ) ) ;
#17248=DIRECTION ( 'NONE',  ( 0.000000000000000000, 0.000000000000000000, -1.000000000000000000 ) ) ;
#17251=DIRECTION ( 'NONE',  ( 1.000000000000000000, 0.000000000000000000, 0.000000000000000000 ) ) ;
#17252=ORIENTED_EDGE ( 'NONE', *, *, #14369, .T. ) ;
#17256=EDGE_LOOP ( 'NONE', ( #7188, #15064 ) ) ;
#17258=VECTOR ( 'NONE', #7316, 1000.000000000000000 ) ;
#17262=LINE ( 'NONE', #1061, #3680 ) ;
#17264=EDGE_CURVE ( 'NONE', #7796, #3840, #17209, .T. ) ;
#17265=EDGE_CURVE ( 'NONE', #9474, #16675, #12972, .T. ) ;
#17267=CARTESIAN_POINT ( 'NONE',  ( 33.28260143222578904, 192.8472041258102934, 25.26942977006888569 ) ) ;
#17268=LINE ( 'NONE', #8933, #10915 ) ;
#17270=CARTESIAN_POINT ( 'NONE',  ( -68.00000000000000000, 171.6227766016838245, 20.00000000000000355 ) ) ;
#17275=ORIENTED_EDGE ( 'NONE', *, *, #10404, .F. ) ;
#17276=LINE ( 'NONE', #5328, #10125 ) ;
#17277=ORIENTED_EDGE ( 'NONE', *, *, #5450, .F. ) ;
#17279=CARTESIAN_POINT ( 'NONE',  ( -96.00000000000001421, 171.6227766016838245, 0.000000000000000000 ) ) ;
#17282=CARTESIAN_POINT ( 'NONE',  ( 14.92136712345229554, 126.5341449364669728, 7.654582290614115436 ) ) ;
#17283=TOROIDAL_SURFACE ( 'NONE', #4006, 240.0000000000000000, 10.00000000000000000 ) ;
#17285=CARTESIAN_POINT ( 'NONE',  ( 15.58496356726128873, 29.99118438505512430, 15.00000000000000000 ) ) ;
#17286=VERTEX_POINT ( 'NONE', #5443 ) ;
#17287=EDGE_CURVE ( 'NONE', #6948, #2358, #7564, .T. ) ;
#17289=ADVANCED_FACE ( 'NONE', ( #2615 ), #8086, .T. ) ;
#17300=ORIENTED_EDGE ( 'NONE', *, *, #4788, .F. ) ;
#17302=ORIENTED_EDGE ( 'NONE', *, *, #394, .F. ) ;
#17303=EDGE_CURVE ( 'NONE', #4748, #4908, #10948, .T. ) ;
#17308=CARTESIAN_POINT ( 'NONE',  ( -15.27350142870561811, 32.46802521863179436, 8.792838265516087048 ) ) ;
#17309=CARTESIAN_POINT ( 'NONE',  ( -7.379000772444994638, 30.00000000000000000, 15.00000000000000000 ) ) ;
#17311=CARTESIAN_POINT ( 'NONE',  ( 28.14717441101696593, 18.00000000000000000, 20.07001214884044415 ) ) ;
#17312=CARTESIAN_POINT ( 'NONE',  ( -84.07431145984972432, 149.5391923287904490, 24.52402115671404204 ) ) ;
#17315=DIRECTION ( 'NONE',  ( 0.000000000000000000, -0.000000000000000000, -1.000000000000000000 ) ) ;
#17316=CARTESIAN_POINT ( 'NONE',  ( 10.11940563665161541, 132.7319563576625399, 14.29042643364863885 ) ) ;
#17318=VERTEX_POINT ( 'NONE', #2697 ) ;
#17319=LINE ( 'NONE', #12101, #6367 ) ;
#17320=CARTESIAN_POINT ( 'NONE',  ( 34.89002926043553288, 197.8146641845671923, 20.09570409464927465 ) ) ;
#17321=ORIENTED_EDGE ( 'NONE', *, *, #3814, .F. ) ;
#17325=ORIENTED_EDGE ( 'NONE', *, *, #13141, .T. ) ;
#17328=LINE ( 'NONE', #1305, #8913 ) ;
#17329=DIRECTION ( 'NONE',  ( 1.000000000000000000, 0.000000000000000000, -0.000000000000000000 ) ) ;
#17330=EDGE_CURVE ( 'NONE', #16016, #11646, #16245, .T. ) ;
#17332=ADVANCED_FACE ( 'NONE', ( #4113 ), #15936, .F. ) ;
#17336=DIRECTION ( 'NONE',  ( 1.000000000000000000, 0.000000000000000000, 0.000000000000000000 ) ) ;
#17337=( NAMED_UNIT ( * ) SI_UNIT ( $, .STERADIAN. ) SOLID_ANGLE_UNIT ( ) );
#17345=CARTESIAN_POINT ( 'NONE',  ( -80.00000000000001421, 196.6227766016838245, 0.000000000000000000 ) ) ;
#17346=DIRECTION ( 'NONE',  ( -1.000000000000000000, 0.000000000000000000, 0.000000000000000000 ) ) ;
#17349=LINE ( 'NONE', #1063, #11490 ) ;
#17352=DIRECTION ( 'NONE',  ( 1.000000000000000000, 0.000000000000000000, 0.000000000000000000 ) ) ;
#17353=CYLINDRICAL_SURFACE ( 'NONE', #1027, 2.499999999999998668 ) ;
#17356=LINE ( 'NONE', #5326, #9176 ) ;
#17361=DIRECTION ( 'NONE',  ( 1.000000000000000000, 0.000000000000000000, 0.000000000000000000 ) ) ;
#17365=CARTESIAN_POINT ( 'NONE',  ( -8.720613081040568204, 20.00000000000000000, 24.99999999951824492 ) ) ;
#17366=CARTESIAN_POINT ( 'NONE',  ( 26.13287303778632165, 139.7415755892579341, 8.533400866158022069 ) ) ;
#17368=DIRECTION ( 'NONE',  ( 1.000000000000000000, 0.000000000000000000, 0.000000000000000000 ) ) ;
#17370=VERTEX_POINT ( 'NONE', #1150 ) ;
#17372=CARTESIAN_POINT ( 'NONE',  ( 15.00000000000903455, 143.2058235767352983, 16.77804593520375676 ) ) ;
#17374=CARTESIAN_POINT ( 'NONE',  ( 196.0000000000000000, 167.6227766016838530, 5.571800142134975431 ) ) ;
#17377=CARTESIAN_POINT ( 'NONE',  ( 26.98389851090235680, 150.6144458722572779, 25.44936967851739595 ) ) ;
#17382=EDGE_CURVE ( 'NONE', #3326, #8820, #2577, .T. ) ;
#17384=EDGE_CURVE ( 'NONE', #17318, #4434, #17181, .T. ) ;
#17385=CIRCLE ( 'NONE', #15680, 250.0000000000000000 ) ;
#17386=VERTEX_POINT ( 'NONE', #15929 ) ;
#17387=EDGE_CURVE ( 'NONE', #16273, #13530, #6439, .T. ) ;
#17389=CARTESIAN_POINT ( 'NONE',  ( 9.380362127004868711, 139.2112497869900949, 14.33999639901018242 ) ) ;
#17390=ORIENTED_EDGE ( 'NONE', *, *, #13274, .F. ) ;
#17394=CIRCLE ( 'NONE', #13431, 10.00000000000000000 ) ;
#17397=CARTESIAN_POINT ( 'NONE',  ( -75.01941192507108269, 147.1381844727103214, 22.12819033745954300 ) ) ;
#17399=VECTOR ( 'NONE', #16972, 1000.000000000000000 ) ;
#17405=CARTESIAN_POINT ( 'NONE',  ( 17.21487247493544714, 29.96934980803111159, 14.74175109707249831 ) ) ;
#17406=EDGE_LOOP ( 'NONE', ( #15293, #4991, #2251, #8175, #3594, #7095, #319, #13446 ) ) ;
#17413=CARTESIAN_POINT ( 'NONE',  ( -68.00000000000000000, 171.6227766016838245, 20.00000000000000355 ) ) ;
#17418=CARTESIAN_POINT ( 'NONE',  ( -8.719536044788661400, 19.99999999999999645, 24.99999999999999645 ) ) ;
#17421=EDGE_LOOP ( 'NONE', ( #4865, #2920 ) ) ;
#17444=LINE ( 'NONE', #13192, #14604 ) ;
#17448=DIRECTION ( 'NONE',  ( -1.000000000000000000, 0.000000000000000000, 0.000000000000000000 ) ) ;
#17461=EDGE_CURVE ( 'NONE', #15706, #11986, #17470, .T. ) ;
#17462=CARTESIAN_POINT ( 'NONE',  ( -13.91527097789397160, 19.99999999999999645, 23.98152295253190758 ) ) ;
#17467=EDGE_LOOP ( 'NONE', ( #10925, #2451, #1439, #9826 ) ) ;
#17470=CIRCLE ( 'NONE', #9824, 2.500000000000000000 ) ;
#17473=EDGE_CURVE ( 'NONE', #8813, #15581, #215, .T. ) ;
#17475=CARTESIAN_POINT ( 'NONE',  ( 49.99999999999998579, 155.6227766016839098, 10.00000337241049309 ) ) ;
#17477=CARTESIAN_POINT ( 'NONE',  ( 32.86958794498660552, 150.7324203247391381, 25.54751979981074683 ) ) ;
#17479=CARTESIAN_POINT ( 'NONE',  ( -25.00000000000002132, 100.0000000000000142, 4.999999999999999112 ) ) ;
#17481=ORIENTED_EDGE ( 'NONE', *, *, #16955, .T. ) ;
#17483=EDGE_LOOP ( 'NONE', ( #7997, #5063 ) ) ;
#17484=ORIENTED_EDGE ( 'NONE', *, *, #7071, .F. ) ;
#17490=CARTESIAN_POINT ( 'NONE',  ( -23.00000000000000000, 120.0000000000000284, 15.00000000000000000 ) ) ;
#17491=CARTESIAN_POINT ( 'NONE',  ( 196.0000000000000000, 175.6227766016838245, 5.571800142134975431 ) ) ;
#17492=EDGE_CURVE ( 'NONE', #4434, #17318, #8708, .T. ) ;
#17494=ADVANCED_FACE ( 'NONE', ( #9452 ), #3902, .F. ) ;
#17495=CARTESIAN_POINT ( 'NONE',  ( -75.76161824504397657, 149.2800176679284903, 24.28646496670947386 ) ) ;
#17497=ADVANCED_FACE ( 'NONE', ( #5312 ), #12861, .F. ) ;
#17499=ORIENTED_EDGE ( 'NONE', *, *, #14106, .T. ) ;
#17501=CARTESIAN_POINT ( 'NONE',  ( 15.60228996708978855, 124.9392590763941371, -1.387778780781445676E-14 ) ) ;
#17502=CARTESIAN_POINT ( 'NONE',  ( 6.927042533203191965, 134.0880917650273716, 15.00000000000000533 ) ) ;
#17504=DIRECTION ( 'NONE',  ( 0.000000000000000000, 0.000000000000000000, 1.000000000000000000 ) ) ;
#17511=CIRCLE ( 'NONE', #547, 20.00000000000000355 ) ;
#17518=EDGE_CURVE ( 'NONE', #5075, #13335, #5875, .T. ) ;
#17519=CARTESIAN_POINT ( 'NONE',  ( 49.99999999999998579, 191.6227766016837677, 8.071800142134975431 ) ) ;
#17521=CYLINDRICAL_SURFACE ( 'NONE', #14631, 2.499999999999998668 ) ;
ENDSEC;
END-ISO-10303-21;
